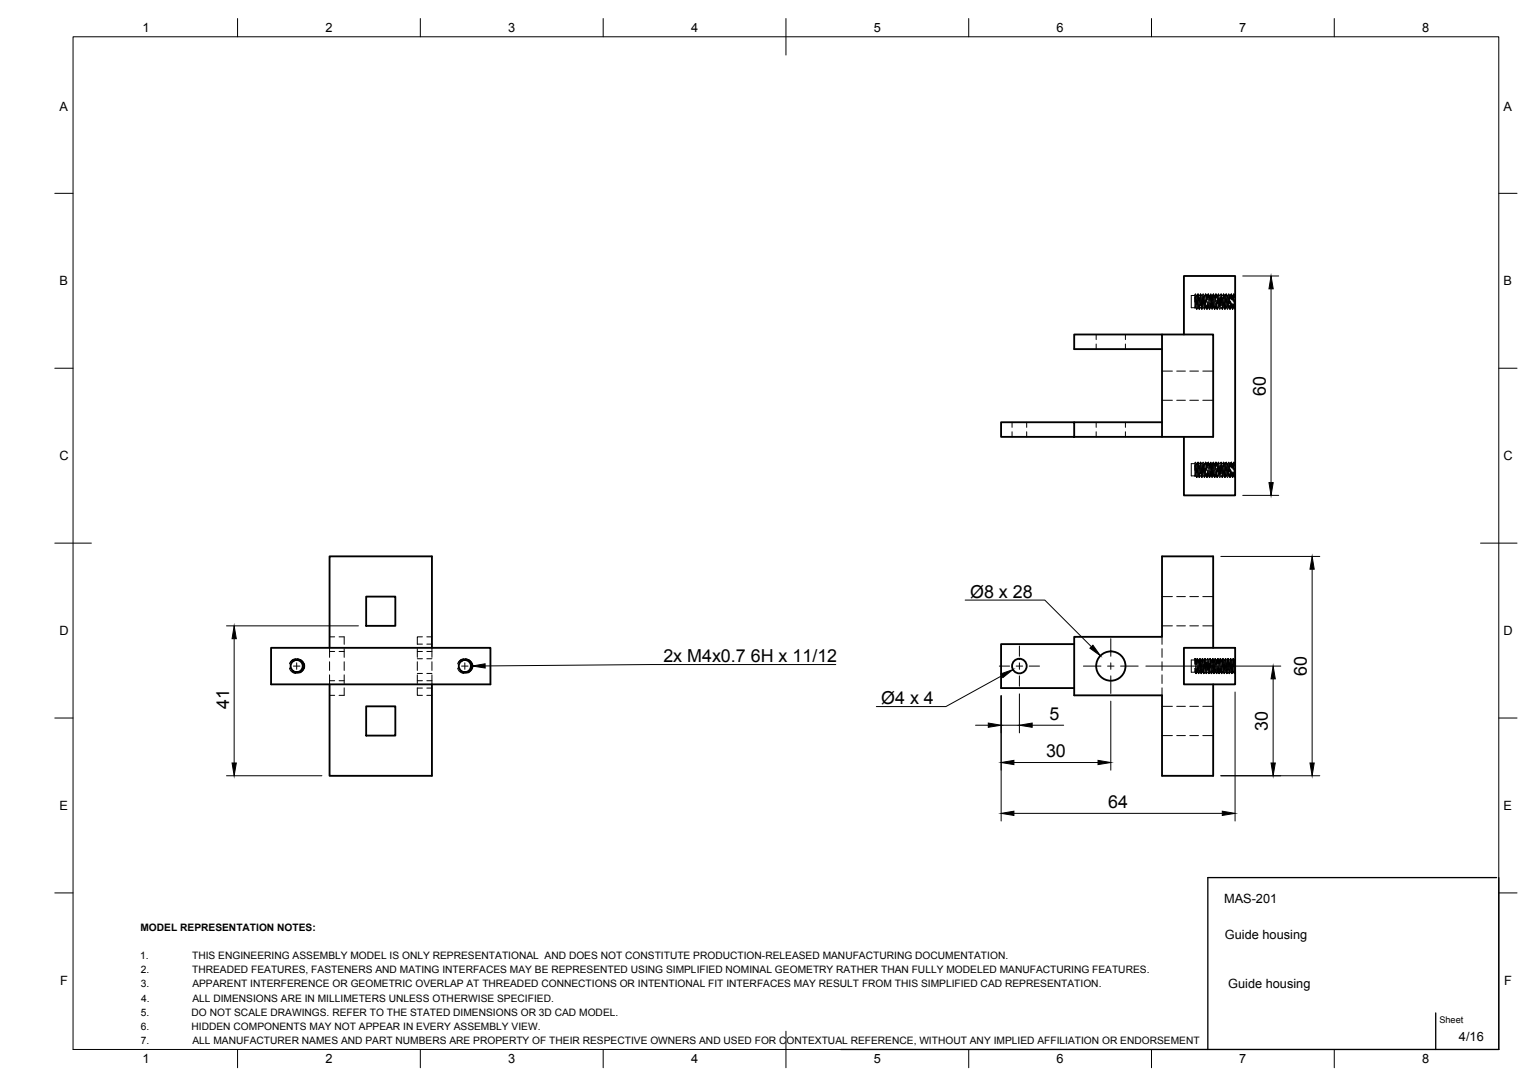
ISO-10303-21;
HEADER;
/* Generated by software containing ST-Developer
 * from STEP Tools, Inc. (www.steptools.com) 
 */

FILE_DESCRIPTION(
/* description */ ('Independent manual two-gate roller-track escapement for nominal30mm d
iameter20mm wide feed rollers. Opposed gates are driven by native capt
ured pin-slot loops with positive curved-slot travel stops at\X\B116de
g. Repeated gate/pin/washer/clip instances, adapted native common bear
ing families, full retaining lips and rotating polymer grip. External 
workpieces, gravity feeder/incline and mount anchors outside assembly.
 No powered-feed compatibility, impact, capacity, safety, force, wear 
or life rating.'),
/* implementation_level */ '2;1');

FILE_NAME(
/* name */ 'Guide housing.step',
/* time_stamp */ '2026-11-08T18:43:23-08:00',
/* author */ (''),
/* organization */ (''),
/* preprocessor_version */ 'ST-DEVELOPER v20.2',
/* originating_system */ 'Autodesk Translation Framework v15.17.0.0',
/* authorisation */ '');

FILE_SCHEMA (('AUTOMOTIVE_DESIGN { 1 0 10303 214 3 1 1 }'));
ENDSEC;

DATA;
#10=MECHANICAL_DESIGN_GEOMETRIC_PRESENTATION_REPRESENTATION('',(#456),#19863);
#117=B_SPLINE_SURFACE_WITH_KNOTS('',3,3,((#11345,#11346,#11347,#11348,#11349,
#11350,#11351,#11352,#11353,#11354,#11355,#11356,#11357,#11358,#11359,#11360,
#11361,#11362,#11363,#11364,#11365,#11366,#11367,#11368,#11369,#11370,#11371,
#11372,#11373,#11374,#11375,#11376,#11377,#11378,#11379,#11380,#11381,#11382,
#11383,#11384,#11385,#11386,#11387,#11388,#11389,#11390,#11391,#11392,#11393,
#11394,#11395,#11396,#11397,#11398,#11399,#11400,#11401,#11402,#11403,#11404,
#11405,#11406,#11407,#11408,#11409,#11410,#11411,#11412,#11413,#11414,#11415,
#11416,#11417,#11418,#11419,#11420,#11421,#11422,#11423,#11424,#11425,#11426,
#11427,#11428,#11429,#11430,#11431,#11432,#11433,#11434,#11435,#11436,#11437,
#11438,#11439,#11440,#11441,#11442,#11443,#11444,#11445,#11446,#11447,#11448),
(#11449,#11450,#11451,#11452,#11453,#11454,#11455,#11456,#11457,#11458,
#11459,#11460,#11461,#11462,#11463,#11464,#11465,#11466,#11467,#11468,#11469,
#11470,#11471,#11472,#11473,#11474,#11475,#11476,#11477,#11478,#11479,#11480,
#11481,#11482,#11483,#11484,#11485,#11486,#11487,#11488,#11489,#11490,#11491,
#11492,#11493,#11494,#11495,#11496,#11497,#11498,#11499,#11500,#11501,#11502,
#11503,#11504,#11505,#11506,#11507,#11508,#11509,#11510,#11511,#11512,#11513,
#11514,#11515,#11516,#11517,#11518,#11519,#11520,#11521,#11522,#11523,#11524,
#11525,#11526,#11527,#11528,#11529,#11530,#11531,#11532,#11533,#11534,#11535,
#11536,#11537,#11538,#11539,#11540,#11541,#11542,#11543,#11544,#11545,#11546,
#11547,#11548,#11549,#11550,#11551,#11552),(#11553,#11554,#11555,#11556,
#11557,#11558,#11559,#11560,#11561,#11562,#11563,#11564,#11565,#11566,#11567,
#11568,#11569,#11570,#11571,#11572,#11573,#11574,#11575,#11576,#11577,#11578,
#11579,#11580,#11581,#11582,#11583,#11584,#11585,#11586,#11587,#11588,#11589,
#11590,#11591,#11592,#11593,#11594,#11595,#11596,#11597,#11598,#11599,#11600,
#11601,#11602,#11603,#11604,#11605,#11606,#11607,#11608,#11609,#11610,#11611,
#11612,#11613,#11614,#11615,#11616,#11617,#11618,#11619,#11620,#11621,#11622,
#11623,#11624,#11625,#11626,#11627,#11628,#11629,#11630,#11631,#11632,#11633,
#11634,#11635,#11636,#11637,#11638,#11639,#11640,#11641,#11642,#11643,#11644,
#11645,#11646,#11647,#11648,#11649,#11650,#11651,#11652,#11653,#11654,#11655,
#11656),(#11657,#11658,#11659,#11660,#11661,#11662,#11663,#11664,#11665,
#11666,#11667,#11668,#11669,#11670,#11671,#11672,#11673,#11674,#11675,#11676,
#11677,#11678,#11679,#11680,#11681,#11682,#11683,#11684,#11685,#11686,#11687,
#11688,#11689,#11690,#11691,#11692,#11693,#11694,#11695,#11696,#11697,#11698,
#11699,#11700,#11701,#11702,#11703,#11704,#11705,#11706,#11707,#11708,#11709,
#11710,#11711,#11712,#11713,#11714,#11715,#11716,#11717,#11718,#11719,#11720,
#11721,#11722,#11723,#11724,#11725,#11726,#11727,#11728,#11729,#11730,#11731,
#11732,#11733,#11734,#11735,#11736,#11737,#11738,#11739,#11740,#11741,#11742,
#11743,#11744,#11745,#11746,#11747,#11748,#11749,#11750,#11751,#11752,#11753,
#11754,#11755,#11756,#11757,#11758,#11759,#11760)),.UNSPECIFIED.,.F.,.F.,
 .F.,(4,4),(4,1,1,1,1,1,1,1,1,1,1,1,1,1,1,1,1,1,1,1,1,1,1,1,1,1,1,1,1,1,
1,1,1,1,1,1,1,1,1,1,1,1,1,1,1,1,1,1,1,1,1,1,1,1,1,1,1,1,1,1,1,1,1,1,1,1,
1,1,1,1,1,1,1,1,1,1,1,1,1,1,1,1,1,1,1,1,1,1,1,1,1,1,1,1,1,1,1,1,1,1,1,4),
(0.,0.0448889834294942),(11.8615800042566,12.8591085386932,13.8566370731298,
14.8541656075664,15.851694142003,16.8492226764396,17.8467512108762,18.8442797453128,
19.8418082797494,20.839336814186,21.8368653486226,22.8343938830592,23.8319224174958,
24.8294509519324,25.826979486369,26.8245080208056,27.8220365552422,28.8195650896788,
29.8170936241154,30.814622158552,31.8121506929886,32.8096792274252,33.8072077618618,
34.8047362962984,35.802264830735,36.7997933651716,37.7973218996082,38.7948504340448,
39.7923789684814,40.789907502918,41.7874360373546,42.7849645717912,43.7824931062278,
44.7800216406644,45.777550175101,46.7750787095376,47.7726072439742,48.7701357784108,
49.7676643128474,50.765192847284,51.7627213817206,52.7602499161572,53.7577784505938,
54.7553069850304,55.752835519467,56.7503640539036,57.7478925883402,58.7454211227768,
59.7429496572134,60.74047819165,61.7380067260866,62.7355352605232,63.7330637949598,
64.7305923293964,65.728120863833,66.7256493982696,67.7231779327062,68.7207064671428,
69.7182350015794,70.715763536016,71.7132920704526,72.7108206048892,73.7083491393258,
74.7058776737624,75.703406208199,76.7009347426356,77.6984632770722,78.6959918115088,
79.6935203459454,80.691048880382,81.6885774148186,82.6861059492552,83.6836344836918,
84.6811630181284,85.678691552565,86.6762200870016,87.6737486214382,88.6712771558748,
89.6688056903114,90.666334224748,91.6638627591846,92.6613912936212,93.6589198280578,
94.6564483624944,95.653976896931,96.6515054313676,97.6490339658042,98.6465625002408,
99.6440910346774,100.641619569114,101.639148103551,102.636676637987,103.634205172424,
104.63173370686,105.629262241297,106.626790775734,107.62431931017,108.621847844607,
109.619376379043,110.61690491348,111.614433447917,112.611961982353),
 .UNSPECIFIED.);
#118=B_SPLINE_SURFACE_WITH_KNOTS('',3,3,((#11868,#11869,#11870,#11871,#11872,
#11873,#11874,#11875,#11876,#11877,#11878,#11879,#11880,#11881,#11882,#11883,
#11884,#11885,#11886,#11887,#11888,#11889,#11890,#11891,#11892,#11893,#11894,
#11895,#11896,#11897,#11898,#11899,#11900,#11901,#11902,#11903,#11904,#11905,
#11906,#11907,#11908,#11909,#11910,#11911,#11912,#11913,#11914,#11915,#11916,
#11917,#11918,#11919,#11920,#11921,#11922,#11923,#11924,#11925,#11926,#11927,
#11928,#11929,#11930,#11931,#11932,#11933,#11934,#11935,#11936,#11937,#11938,
#11939,#11940,#11941,#11942,#11943,#11944,#11945,#11946,#11947,#11948,#11949,
#11950,#11951,#11952,#11953,#11954,#11955,#11956,#11957,#11958,#11959,#11960,
#11961,#11962,#11963,#11964,#11965,#11966,#11967,#11968,#11969,#11970,#11971),
(#11972,#11973,#11974,#11975,#11976,#11977,#11978,#11979,#11980,#11981,
#11982,#11983,#11984,#11985,#11986,#11987,#11988,#11989,#11990,#11991,#11992,
#11993,#11994,#11995,#11996,#11997,#11998,#11999,#12000,#12001,#12002,#12003,
#12004,#12005,#12006,#12007,#12008,#12009,#12010,#12011,#12012,#12013,#12014,
#12015,#12016,#12017,#12018,#12019,#12020,#12021,#12022,#12023,#12024,#12025,
#12026,#12027,#12028,#12029,#12030,#12031,#12032,#12033,#12034,#12035,#12036,
#12037,#12038,#12039,#12040,#12041,#12042,#12043,#12044,#12045,#12046,#12047,
#12048,#12049,#12050,#12051,#12052,#12053,#12054,#12055,#12056,#12057,#12058,
#12059,#12060,#12061,#12062,#12063,#12064,#12065,#12066,#12067,#12068,#12069,
#12070,#12071,#12072,#12073,#12074,#12075),(#12076,#12077,#12078,#12079,
#12080,#12081,#12082,#12083,#12084,#12085,#12086,#12087,#12088,#12089,#12090,
#12091,#12092,#12093,#12094,#12095,#12096,#12097,#12098,#12099,#12100,#12101,
#12102,#12103,#12104,#12105,#12106,#12107,#12108,#12109,#12110,#12111,#12112,
#12113,#12114,#12115,#12116,#12117,#12118,#12119,#12120,#12121,#12122,#12123,
#12124,#12125,#12126,#12127,#12128,#12129,#12130,#12131,#12132,#12133,#12134,
#12135,#12136,#12137,#12138,#12139,#12140,#12141,#12142,#12143,#12144,#12145,
#12146,#12147,#12148,#12149,#12150,#12151,#12152,#12153,#12154,#12155,#12156,
#12157,#12158,#12159,#12160,#12161,#12162,#12163,#12164,#12165,#12166,#12167,
#12168,#12169,#12170,#12171,#12172,#12173,#12174,#12175,#12176,#12177,#12178,
#12179),(#12180,#12181,#12182,#12183,#12184,#12185,#12186,#12187,#12188,
#12189,#12190,#12191,#12192,#12193,#12194,#12195,#12196,#12197,#12198,#12199,
#12200,#12201,#12202,#12203,#12204,#12205,#12206,#12207,#12208,#12209,#12210,
#12211,#12212,#12213,#12214,#12215,#12216,#12217,#12218,#12219,#12220,#12221,
#12222,#12223,#12224,#12225,#12226,#12227,#12228,#12229,#12230,#12231,#12232,
#12233,#12234,#12235,#12236,#12237,#12238,#12239,#12240,#12241,#12242,#12243,
#12244,#12245,#12246,#12247,#12248,#12249,#12250,#12251,#12252,#12253,#12254,
#12255,#12256,#12257,#12258,#12259,#12260,#12261,#12262,#12263,#12264,#12265,
#12266,#12267,#12268,#12269,#12270,#12271,#12272,#12273,#12274,#12275,#12276,
#12277,#12278,#12279,#12280,#12281,#12282,#12283)),.UNSPECIFIED.,.F.,.F.,
 .F.,(4,4),(4,1,1,1,1,1,1,1,1,1,1,1,1,1,1,1,1,1,1,1,1,1,1,1,1,1,1,1,1,1,
1,1,1,1,1,1,1,1,1,1,1,1,1,1,1,1,1,1,1,1,1,1,1,1,1,1,1,1,1,1,1,1,1,1,1,1,
1,1,1,1,1,1,1,1,1,1,1,1,1,1,1,1,1,1,1,1,1,1,1,1,1,1,1,1,1,1,1,1,1,1,1,4),
(0.,0.0448889834294942),(14.3981410127769,15.3956695472135,16.3931980816501,
17.3907266160867,18.3882551505233,19.3857836849599,20.3833122193965,21.3808407538331,
22.3783692882697,23.3758978227063,24.3734263571429,25.3709548915795,26.3684834260161,
27.3660119604527,28.3635404948893,29.3610690293259,30.3585975637625,31.3561260981991,
32.3536546326357,33.3511831670723,34.3487117015089,35.3462402359455,36.3437687703821,
37.3412973048187,38.3388258392553,39.3363543736919,40.3338829081285,41.3314114425651,
42.3289399770017,43.3264685114383,44.3239970458749,45.3215255803115,46.3190541147481,
47.3165826491847,48.3141111836213,49.3116397180579,50.3091682524945,51.3066967869311,
52.3042253213677,53.3017538558043,54.2992823902409,55.2968109246775,56.294339459114,
57.2918679935507,58.2893965279873,59.2869250624238,60.2844535968605,61.281982131297,
62.2795106657336,63.2770392001703,64.2745677346068,65.2720962690434,66.26962480348,
67.2671533379167,68.2646818723532,69.2622104067898,70.2597389412264,71.257267475663,
72.2547960100996,73.2523245445362,74.2498530789728,75.2473816134094,76.244910147846,
77.2424386822826,78.2399672167192,79.2374957511558,80.2350242855924,81.232552820029,
82.2300813544656,83.2276098889022,84.2251384233388,85.2226669577754,86.220195492212,
87.2177240266486,88.2152525610852,89.2127810955218,90.2103096299584,91.207838164395,
92.2053666988316,93.2028952332682,94.2004237677048,95.1979523021414,96.195480836578,
97.1930093710146,98.1905379054512,99.1880664398878,100.185594974324,101.183123508761,
102.180652043198,103.178180577634,104.175709112071,105.173237646507,106.170766180944,
107.168294715381,108.165823249817,109.163351784254,110.16088031869,111.158408853127,
112.155937387564,113.153465922,114.150994456437,115.148522990873),
 .UNSPECIFIED.);
#119=B_SPLINE_SURFACE_WITH_KNOTS('',3,3,((#12588,#12589,#12590,#12591,#12592,
#12593,#12594,#12595,#12596,#12597,#12598,#12599,#12600,#12601,#12602,#12603,
#12604,#12605,#12606,#12607,#12608,#12609,#12610,#12611,#12612,#12613,#12614,
#12615,#12616,#12617,#12618,#12619,#12620,#12621,#12622,#12623,#12624,#12625,
#12626,#12627,#12628,#12629,#12630,#12631,#12632,#12633,#12634,#12635,#12636,
#12637,#12638,#12639,#12640,#12641,#12642,#12643,#12644,#12645,#12646,#12647,
#12648,#12649,#12650,#12651,#12652,#12653,#12654,#12655,#12656,#12657,#12658,
#12659,#12660,#12661,#12662,#12663,#12664,#12665,#12666,#12667,#12668,#12669,
#12670,#12671,#12672,#12673,#12674,#12675,#12676,#12677,#12678,#12679,#12680,
#12681,#12682,#12683,#12684,#12685,#12686,#12687,#12688,#12689,#12690,#12691),
(#12692,#12693,#12694,#12695,#12696,#12697,#12698,#12699,#12700,#12701,
#12702,#12703,#12704,#12705,#12706,#12707,#12708,#12709,#12710,#12711,#12712,
#12713,#12714,#12715,#12716,#12717,#12718,#12719,#12720,#12721,#12722,#12723,
#12724,#12725,#12726,#12727,#12728,#12729,#12730,#12731,#12732,#12733,#12734,
#12735,#12736,#12737,#12738,#12739,#12740,#12741,#12742,#12743,#12744,#12745,
#12746,#12747,#12748,#12749,#12750,#12751,#12752,#12753,#12754,#12755,#12756,
#12757,#12758,#12759,#12760,#12761,#12762,#12763,#12764,#12765,#12766,#12767,
#12768,#12769,#12770,#12771,#12772,#12773,#12774,#12775,#12776,#12777,#12778,
#12779,#12780,#12781,#12782,#12783,#12784,#12785,#12786,#12787,#12788,#12789,
#12790,#12791,#12792,#12793,#12794,#12795),(#12796,#12797,#12798,#12799,
#12800,#12801,#12802,#12803,#12804,#12805,#12806,#12807,#12808,#12809,#12810,
#12811,#12812,#12813,#12814,#12815,#12816,#12817,#12818,#12819,#12820,#12821,
#12822,#12823,#12824,#12825,#12826,#12827,#12828,#12829,#12830,#12831,#12832,
#12833,#12834,#12835,#12836,#12837,#12838,#12839,#12840,#12841,#12842,#12843,
#12844,#12845,#12846,#12847,#12848,#12849,#12850,#12851,#12852,#12853,#12854,
#12855,#12856,#12857,#12858,#12859,#12860,#12861,#12862,#12863,#12864,#12865,
#12866,#12867,#12868,#12869,#12870,#12871,#12872,#12873,#12874,#12875,#12876,
#12877,#12878,#12879,#12880,#12881,#12882,#12883,#12884,#12885,#12886,#12887,
#12888,#12889,#12890,#12891,#12892,#12893,#12894,#12895,#12896,#12897,#12898,
#12899),(#12900,#12901,#12902,#12903,#12904,#12905,#12906,#12907,#12908,
#12909,#12910,#12911,#12912,#12913,#12914,#12915,#12916,#12917,#12918,#12919,
#12920,#12921,#12922,#12923,#12924,#12925,#12926,#12927,#12928,#12929,#12930,
#12931,#12932,#12933,#12934,#12935,#12936,#12937,#12938,#12939,#12940,#12941,
#12942,#12943,#12944,#12945,#12946,#12947,#12948,#12949,#12950,#12951,#12952,
#12953,#12954,#12955,#12956,#12957,#12958,#12959,#12960,#12961,#12962,#12963,
#12964,#12965,#12966,#12967,#12968,#12969,#12970,#12971,#12972,#12973,#12974,
#12975,#12976,#12977,#12978,#12979,#12980,#12981,#12982,#12983,#12984,#12985,
#12986,#12987,#12988,#12989,#12990,#12991,#12992,#12993,#12994,#12995,#12996,
#12997,#12998,#12999,#13000,#13001,#13002,#13003)),.UNSPECIFIED.,.F.,.F.,
 .F.,(4,4),(4,1,1,1,1,1,1,1,1,1,1,1,1,1,1,1,1,1,1,1,1,1,1,1,1,1,1,1,1,1,
1,1,1,1,1,1,1,1,1,1,1,1,1,1,1,1,1,1,1,1,1,1,1,1,1,1,1,1,1,1,1,1,1,1,1,1,
1,1,1,1,1,1,1,1,1,1,1,1,1,1,1,1,1,1,1,1,1,1,1,1,1,1,1,1,1,1,1,1,1,1,1,4),
(0.,0.0448889834294942),(11.8615800042566,12.8591085386932,13.8566370731298,
14.8541656075664,15.851694142003,16.8492226764396,17.8467512108762,18.8442797453128,
19.8418082797494,20.839336814186,21.8368653486226,22.8343938830592,23.8319224174958,
24.8294509519324,25.826979486369,26.8245080208056,27.8220365552422,28.8195650896788,
29.8170936241154,30.814622158552,31.8121506929886,32.8096792274252,33.8072077618618,
34.8047362962984,35.802264830735,36.7997933651716,37.7973218996082,38.7948504340448,
39.7923789684814,40.789907502918,41.7874360373546,42.7849645717912,43.7824931062278,
44.7800216406644,45.777550175101,46.7750787095376,47.7726072439742,48.7701357784108,
49.7676643128474,50.765192847284,51.7627213817206,52.7602499161572,53.7577784505938,
54.7553069850304,55.752835519467,56.7503640539036,57.7478925883402,58.7454211227768,
59.7429496572134,60.74047819165,61.7380067260866,62.7355352605232,63.7330637949598,
64.7305923293964,65.728120863833,66.7256493982696,67.7231779327062,68.7207064671428,
69.7182350015794,70.715763536016,71.7132920704526,72.7108206048892,73.7083491393258,
74.7058776737624,75.703406208199,76.7009347426356,77.6984632770722,78.6959918115088,
79.6935203459454,80.691048880382,81.6885774148186,82.6861059492552,83.6836344836918,
84.6811630181284,85.678691552565,86.6762200870016,87.6737486214382,88.6712771558748,
89.6688056903114,90.666334224748,91.6638627591846,92.6613912936212,93.6589198280578,
94.6564483624944,95.653976896931,96.6515054313676,97.6490339658042,98.6465625002408,
99.6440910346774,100.641619569114,101.639148103551,102.636676637987,103.634205172424,
104.63173370686,105.629262241297,106.626790775734,107.62431931017,108.621847844607,
109.619376379043,110.61690491348,111.614433447917,112.611961982353),
 .UNSPECIFIED.);
#120=B_SPLINE_SURFACE_WITH_KNOTS('',3,3,((#13111,#13112,#13113,#13114,#13115,
#13116,#13117,#13118,#13119,#13120,#13121,#13122,#13123,#13124,#13125,#13126,
#13127,#13128,#13129,#13130,#13131,#13132,#13133,#13134,#13135,#13136,#13137,
#13138,#13139,#13140,#13141,#13142,#13143,#13144,#13145,#13146,#13147,#13148,
#13149,#13150,#13151,#13152,#13153,#13154,#13155,#13156,#13157,#13158,#13159,
#13160,#13161,#13162,#13163,#13164,#13165,#13166,#13167,#13168,#13169,#13170,
#13171,#13172,#13173,#13174,#13175,#13176,#13177,#13178,#13179,#13180,#13181,
#13182,#13183,#13184,#13185,#13186,#13187,#13188,#13189,#13190,#13191,#13192,
#13193,#13194,#13195,#13196,#13197,#13198,#13199,#13200,#13201,#13202,#13203,
#13204,#13205,#13206,#13207,#13208,#13209,#13210,#13211,#13212,#13213,#13214),
(#13215,#13216,#13217,#13218,#13219,#13220,#13221,#13222,#13223,#13224,
#13225,#13226,#13227,#13228,#13229,#13230,#13231,#13232,#13233,#13234,#13235,
#13236,#13237,#13238,#13239,#13240,#13241,#13242,#13243,#13244,#13245,#13246,
#13247,#13248,#13249,#13250,#13251,#13252,#13253,#13254,#13255,#13256,#13257,
#13258,#13259,#13260,#13261,#13262,#13263,#13264,#13265,#13266,#13267,#13268,
#13269,#13270,#13271,#13272,#13273,#13274,#13275,#13276,#13277,#13278,#13279,
#13280,#13281,#13282,#13283,#13284,#13285,#13286,#13287,#13288,#13289,#13290,
#13291,#13292,#13293,#13294,#13295,#13296,#13297,#13298,#13299,#13300,#13301,
#13302,#13303,#13304,#13305,#13306,#13307,#13308,#13309,#13310,#13311,#13312,
#13313,#13314,#13315,#13316,#13317,#13318),(#13319,#13320,#13321,#13322,
#13323,#13324,#13325,#13326,#13327,#13328,#13329,#13330,#13331,#13332,#13333,
#13334,#13335,#13336,#13337,#13338,#13339,#13340,#13341,#13342,#13343,#13344,
#13345,#13346,#13347,#13348,#13349,#13350,#13351,#13352,#13353,#13354,#13355,
#13356,#13357,#13358,#13359,#13360,#13361,#13362,#13363,#13364,#13365,#13366,
#13367,#13368,#13369,#13370,#13371,#13372,#13373,#13374,#13375,#13376,#13377,
#13378,#13379,#13380,#13381,#13382,#13383,#13384,#13385,#13386,#13387,#13388,
#13389,#13390,#13391,#13392,#13393,#13394,#13395,#13396,#13397,#13398,#13399,
#13400,#13401,#13402,#13403,#13404,#13405,#13406,#13407,#13408,#13409,#13410,
#13411,#13412,#13413,#13414,#13415,#13416,#13417,#13418,#13419,#13420,#13421,
#13422),(#13423,#13424,#13425,#13426,#13427,#13428,#13429,#13430,#13431,
#13432,#13433,#13434,#13435,#13436,#13437,#13438,#13439,#13440,#13441,#13442,
#13443,#13444,#13445,#13446,#13447,#13448,#13449,#13450,#13451,#13452,#13453,
#13454,#13455,#13456,#13457,#13458,#13459,#13460,#13461,#13462,#13463,#13464,
#13465,#13466,#13467,#13468,#13469,#13470,#13471,#13472,#13473,#13474,#13475,
#13476,#13477,#13478,#13479,#13480,#13481,#13482,#13483,#13484,#13485,#13486,
#13487,#13488,#13489,#13490,#13491,#13492,#13493,#13494,#13495,#13496,#13497,
#13498,#13499,#13500,#13501,#13502,#13503,#13504,#13505,#13506,#13507,#13508,
#13509,#13510,#13511,#13512,#13513,#13514,#13515,#13516,#13517,#13518,#13519,
#13520,#13521,#13522,#13523,#13524,#13525,#13526)),.UNSPECIFIED.,.F.,.F.,
 .F.,(4,4),(4,1,1,1,1,1,1,1,1,1,1,1,1,1,1,1,1,1,1,1,1,1,1,1,1,1,1,1,1,1,
1,1,1,1,1,1,1,1,1,1,1,1,1,1,1,1,1,1,1,1,1,1,1,1,1,1,1,1,1,1,1,1,1,1,1,1,
1,1,1,1,1,1,1,1,1,1,1,1,1,1,1,1,1,1,1,1,1,1,1,1,1,1,1,1,1,1,1,1,1,1,1,4),
(0.,0.0448889834294942),(14.3981410127769,15.3956695472135,16.3931980816501,
17.3907266160867,18.3882551505233,19.3857836849599,20.3833122193965,21.3808407538331,
22.3783692882697,23.3758978227063,24.3734263571429,25.3709548915795,26.3684834260161,
27.3660119604527,28.3635404948893,29.3610690293259,30.3585975637625,31.3561260981991,
32.3536546326357,33.3511831670723,34.3487117015089,35.3462402359455,36.3437687703821,
37.3412973048187,38.3388258392553,39.3363543736919,40.3338829081285,41.3314114425651,
42.3289399770017,43.3264685114383,44.3239970458749,45.3215255803115,46.3190541147481,
47.3165826491847,48.3141111836213,49.3116397180579,50.3091682524945,51.3066967869311,
52.3042253213677,53.3017538558043,54.2992823902409,55.2968109246775,56.294339459114,
57.2918679935507,58.2893965279873,59.2869250624238,60.2844535968605,61.281982131297,
62.2795106657336,63.2770392001703,64.2745677346068,65.2720962690434,66.26962480348,
67.2671533379167,68.2646818723532,69.2622104067898,70.2597389412264,71.257267475663,
72.2547960100996,73.2523245445362,74.2498530789728,75.2473816134094,76.244910147846,
77.2424386822826,78.2399672167192,79.2374957511558,80.2350242855924,81.232552820029,
82.2300813544656,83.2276098889022,84.2251384233388,85.2226669577754,86.220195492212,
87.2177240266486,88.2152525610852,89.2127810955218,90.2103096299584,91.207838164395,
92.2053666988316,93.2028952332682,94.2004237677048,95.1979523021414,96.195480836578,
97.1930093710146,98.1905379054512,99.1880664398878,100.185594974324,101.183123508761,
102.180652043198,103.178180577634,104.175709112071,105.173237646507,106.170766180944,
107.168294715381,108.165823249817,109.163351784254,110.16088031869,111.158408853127,
112.155937387564,113.153465922,114.150994456437,115.148522990873),
 .UNSPECIFIED.);
#127=B_SPLINE_CURVE_WITH_KNOTS('',3,(#8912,#8913,#8914,#8915,#8916,#8917,
#8918,#8919,#8920,#8921,#8922,#8923,#8924,#8925,#8926,#8927,#8928,#8929,
#8930),.UNSPECIFIED.,.F.,.F.,(4,3,3,3,3,3,4),(95.5576018628658,95.7627393059135,
96.7602678403501,97.7577963747867,98.7553249092233,99.7528534436599,100.750381978097),
 .UNSPECIFIED.);
#128=B_SPLINE_CURVE_WITH_KNOTS('',3,(#8934,#8935,#8936,#8937),
 .UNSPECIFIED.,.F.,.F.,(4,4),(-98.7357691128221,-98.0941628713861),
 .UNSPECIFIED.);
#129=B_SPLINE_CURVE_WITH_KNOTS('',3,(#8941,#8942,#8943,#8944,#8945,#8946,
#8947,#8948,#8949,#8950,#8951,#8952,#8953,#8954,#8955,#8956,#8957,#8958,
#8959,#8960,#8961,#8962),.UNSPECIFIED.,.F.,.F.,(4,3,3,3,3,3,3,4),(-98.0941628713861,
-97.7577963747867,-96.7602678403501,-95.7627393059135,-94.7652107714769,
-93.7676822370403,-92.7701537026037,-91.8109775642065),.UNSPECIFIED.);
#130=B_SPLINE_CURVE_WITH_KNOTS('',3,(#8967,#8968,#8969,#8970,#8971,#8972,
#8973,#8974,#8975,#8976,#8977,#8978,#8979,#8980,#8981,#8982,#8983,#8984,
#8985,#8986,#8987,#8988),.UNSPECIFIED.,.F.,.F.,(4,3,3,3,3,3,3,4),(89.2744165556862,
89.7775680992939,90.7750966337306,91.7726251681671,92.7701537026037,93.7676822370403,
94.7652107714769,95.5576018628658),.UNSPECIFIED.);
#131=B_SPLINE_CURVE_WITH_KNOTS('',3,(#8989,#8990,#8991,#8992,#8993,#8994,
#8995,#8996,#8997,#8998,#8999,#9000,#9001,#9002,#9003,#9004,#9005,#9006,
#9007,#9008,#9009,#9010,#9011,#9012,#9013),.UNSPECIFIED.,.F.,.F.,(4,3,3,
3,3,3,3,3,4),(-91.8109775642065,-91.7726251681671,-90.7750966337305,-89.7775680992939,
-88.7800395648573,-87.7825110304207,-86.7849824959842,-85.7874539615476,
-85.5277922570269),.UNSPECIFIED.);
#132=B_SPLINE_CURVE_WITH_KNOTS('',3,(#9018,#9019,#9020,#9021,#9022,#9023,
#9024,#9025,#9026,#9027,#9028,#9029,#9030,#9031,#9032,#9033,#9034,#9035,
#9036,#9037,#9038,#9039),.UNSPECIFIED.,.F.,.F.,(4,3,3,3,3,3,3,4),(82.9912312485066,
83.7923968926743,84.7899254271109,85.7874539615476,86.7849824959841,87.7825110304207,
88.7800395648573,89.2744165556862),.UNSPECIFIED.);
#133=B_SPLINE_CURVE_WITH_KNOTS('',3,(#9040,#9041,#9042,#9043,#9044,#9045,
#9046,#9047,#9048,#9049,#9050,#9051,#9052,#9053,#9054,#9055,#9056,#9057,
#9058,#9059,#9060,#9061),.UNSPECIFIED.,.F.,.F.,(4,3,3,3,3,3,3,4),(-85.5277922570269,
-84.789925427111,-83.7923968926743,-82.7948683582377,-81.7973398238011,
-80.7998112893646,-79.8022827549279,-79.2446069498473),.UNSPECIFIED.);
#134=B_SPLINE_CURVE_WITH_KNOTS('',3,(#9066,#9067,#9068,#9069,#9070,#9071,
#9072,#9073,#9074,#9075,#9076,#9077,#9078,#9079,#9080,#9081,#9082,#9083,
#9084,#9085,#9086,#9087,#9088,#9089,#9090),.UNSPECIFIED.,.F.,.F.,(4,3,3,
3,3,3,3,3,4),(76.708045941327,76.8096971516181,77.8072256860547,78.8047542204914,
79.8022827549279,80.7998112893646,81.7973398238011,82.7948683582377,82.9912312485066),
 .UNSPECIFIED.);
#135=B_SPLINE_CURVE_WITH_KNOTS('',3,(#9091,#9092,#9093,#9094,#9095,#9096,
#9097,#9098,#9099,#9100,#9101,#9102,#9103,#9104,#9105,#9106,#9107,#9108,
#9109,#9110,#9111,#9112),.UNSPECIFIED.,.F.,.F.,(4,3,3,3,3,3,3,4),(-79.2446069498473,
-78.8047542204913,-77.8072256860547,-76.8096971516181,-75.8121686171815,
-74.8146400827449,-73.8171115483083,-72.9614216426677),.UNSPECIFIED.);
#136=B_SPLINE_CURVE_WITH_KNOTS('',3,(#9117,#9118,#9119,#9120,#9121,#9122,
#9123,#9124,#9125,#9126,#9127,#9128,#9129,#9130,#9131,#9132,#9133,#9134,
#9135,#9136,#9137,#9138),.UNSPECIFIED.,.F.,.F.,(4,3,3,3,3,3,3,4),(70.4248606341474,
70.8245259449985,71.8220544794352,72.8195830138717,73.8171115483084,74.8146400827449,
75.8121686171816,76.708045941327),.UNSPECIFIED.);
#137=B_SPLINE_CURVE_WITH_KNOTS('',3,(#9139,#9140,#9141,#9142,#9143,#9144,
#9145,#9146,#9147,#9148,#9149,#9150,#9151,#9152,#9153,#9154,#9155,#9156,
#9157,#9158,#9159,#9160,#9161,#9162,#9163),.UNSPECIFIED.,.F.,.F.,(4,3,3,
3,3,3,3,3,4),(-72.9614216426677,-72.8195830138717,-71.8220544794352,-70.8245259449986,
-69.8269974105619,-68.8294688761253,-67.8319403416887,-66.8344118072522,
-66.6782363354881),.UNSPECIFIED.);
#138=B_SPLINE_CURVE_WITH_KNOTS('',3,(#9168,#9169,#9170,#9171,#9172,#9173,
#9174,#9175,#9176,#9177,#9178,#9179,#9180,#9181,#9182,#9183,#9184,#9185,
#9186,#9187,#9188,#9189),.UNSPECIFIED.,.F.,.F.,(4,3,3,3,3,3,3,4),(64.1416753269678,
64.839354738379,65.8368832728156,66.8344118072522,67.8319403416887,68.8294688761253,
69.8269974105619,70.4248606341474),.UNSPECIFIED.);
#139=B_SPLINE_CURVE_WITH_KNOTS('',3,(#9190,#9191,#9192,#9193,#9194,#9195,
#9196,#9197,#9198,#9199,#9200,#9201,#9202,#9203,#9204,#9205,#9206,#9207,
#9208,#9209,#9210,#9211),.UNSPECIFIED.,.F.,.F.,(4,3,3,3,3,3,3,4),(-66.6782363354881,
-65.8368832728156,-64.839354738379,-63.8418262039424,-62.8442976695058,
-61.8467691350692,-60.8492406006326,-60.3950510283086),.UNSPECIFIED.);
#140=B_SPLINE_CURVE_WITH_KNOTS('',3,(#9216,#9217,#9218,#9219,#9220,#9221,
#9222,#9223,#9224,#9225,#9226,#9227,#9228,#9229,#9230,#9231,#9232,#9233,
#9234,#9235,#9236,#9237),.UNSPECIFIED.,.F.,.F.,(4,3,3,3,3,3,3,4),(57.8584900197882,
58.8541835317594,59.851712066196,60.8492406006326,61.8467691350692,62.8442976695058,
63.8418262039424,64.1416753269678),.UNSPECIFIED.);
#141=B_SPLINE_CURVE_WITH_KNOTS('',3,(#9238,#9239,#9240,#9241,#9242,#9243,
#9244,#9245,#9246,#9247,#9248,#9249,#9250,#9251,#9252,#9253,#9254,#9255,
#9256,#9257,#9258,#9259),.UNSPECIFIED.,.F.,.F.,(4,3,3,3,3,3,3,4),(-60.3950510283086,
-59.851712066196,-58.8541835317594,-57.8566549973228,-56.8591264628862,
-55.8615979284496,-54.864069394013,-54.111865721129),.UNSPECIFIED.);
#142=B_SPLINE_CURVE_WITH_KNOTS('',3,(#9264,#9265,#9266,#9267,#9268,#9269,
#9270,#9271,#9272,#9273,#9274,#9275,#9276,#9277,#9278,#9279,#9280,#9281,
#9282,#9283,#9284,#9285),.UNSPECIFIED.,.F.,.F.,(4,3,3,3,3,3,3,4),(51.5753047126086,
51.8714837907032,52.8690123251398,53.8665408595764,54.864069394013,55.8615979284496,
56.8591264628862,57.8584900197882),.UNSPECIFIED.);
#143=B_SPLINE_CURVE_WITH_KNOTS('',3,(#9286,#9287,#9288,#9289,#9290,#9291,
#9292,#9293,#9294,#9295,#9296,#9297,#9298,#9299,#9300,#9301,#9302,#9303,
#9304,#9305,#9306,#9307,#9308,#9309,#9310),.UNSPECIFIED.,.F.,.F.,(4,3,3,
3,3,3,3,3,4),(-54.111865721129,-53.8665408595764,-52.8690123251398,-51.8714837907032,
-50.8739552562666,-49.87642672183,-48.8788981873934,-47.8813696529568,-47.8286804139494),
 .UNSPECIFIED.);
#144=B_SPLINE_CURVE_WITH_KNOTS('',3,(#9315,#9316,#9317,#9318,#9319,#9320,
#9321,#9322,#9323,#9324,#9325,#9326,#9327,#9328,#9329,#9330,#9331,#9332,
#9333,#9334,#9335,#9336),.UNSPECIFIED.,.F.,.F.,(4,3,3,3,3,3,3,4),(45.2921194054291,
45.8863125840836,46.8838411185202,47.8813696529568,48.8788981873934,49.87642672183,
50.8739552562666,51.5753047126086),.UNSPECIFIED.);
#145=B_SPLINE_CURVE_WITH_KNOTS('',3,(#9337,#9338,#9339,#9340,#9341,#9342,
#9343,#9344,#9345,#9346,#9347,#9348,#9349,#9350,#9351,#9352,#9353,#9354,
#9355,#9356,#9357,#9358),.UNSPECIFIED.,.F.,.F.,(4,3,3,3,3,3,3,4),(-47.8286804139494,
-46.8838411185202,-45.8863125840836,-44.888784049647,-43.8912555152104,
-42.8937269807738,-41.8961984463372,-41.5454951067698),.UNSPECIFIED.);
#146=B_SPLINE_CURVE_WITH_KNOTS('',3,(#9363,#9364,#9365,#9366,#9367,#9368,
#9369,#9370,#9371,#9372,#9373,#9374,#9375,#9376,#9377,#9378,#9379,#9380,
#9381,#9382,#9383,#9384),.UNSPECIFIED.,.F.,.F.,(4,3,3,3,3,3,3,4),(39.0089340982495,
39.901141377464,40.8986699119006,41.8961984463372,42.8937269807738,43.8912555152104,
44.888784049647,45.2921194054291),.UNSPECIFIED.);
#147=B_SPLINE_CURVE_WITH_KNOTS('',3,(#9385,#9386,#9387,#9388,#9389,#9390,
#9391,#9392,#9393,#9394,#9395,#9396,#9397,#9398,#9399,#9400,#9401,#9402,
#9403,#9404,#9405,#9406),.UNSPECIFIED.,.F.,.F.,(4,3,3,3,3,3,3,4),(-41.5454951067698,
-40.8986699119006,-39.901141377464,-38.9036128430274,-37.9060843085908,
-36.9085557741542,-35.9110272397176,-35.2623097995902),.UNSPECIFIED.);
#148=B_SPLINE_CURVE_WITH_KNOTS('',3,(#9411,#9412,#9413,#9414,#9415,#9416,
#9417,#9418,#9419,#9420,#9421,#9422,#9423,#9424,#9425,#9426,#9427,#9428,
#9429,#9430,#9431,#9432,#9433,#9434,#9435),.UNSPECIFIED.,.F.,.F.,(4,3,3,
3,3,3,3,3,4),(32.7257487910699,32.9184416364078,33.9159701708444,34.913498705281,
35.9110272397176,36.9085557741542,37.9060843085908,38.9036128430274,39.0089340982495),
 .UNSPECIFIED.);
#149=B_SPLINE_CURVE_WITH_KNOTS('',3,(#9436,#9437,#9438,#9439,#9440,#9441,
#9442,#9443,#9444,#9445,#9446,#9447,#9448,#9449,#9450,#9451,#9452,#9453,
#9454,#9455,#9456,#9457),.UNSPECIFIED.,.F.,.F.,(4,3,3,3,3,3,3,4),(-35.2623097995902,
-34.913498705281,-33.9159701708444,-32.9184416364078,-31.9209131019712,
-30.9233845675346,-29.925856033098,-28.9791244924106),.UNSPECIFIED.);
#150=B_SPLINE_CURVE_WITH_KNOTS('',3,(#9462,#9463,#9464,#9465,#9466,#9467,
#9468,#9469,#9470,#9471,#9472,#9473,#9474,#9475,#9476,#9477,#9478,#9479,
#9480,#9481,#9482,#9483),.UNSPECIFIED.,.F.,.F.,(4,3,3,3,3,3,3,4),(26.4425634838903,
26.9332704297882,27.9307989642248,28.9283274986614,29.925856033098,30.9233845675346,
31.9209131019712,32.7257487910699),.UNSPECIFIED.);
#151=B_SPLINE_CURVE_WITH_KNOTS('',3,(#9484,#9485,#9486,#9487,#9488,#9489,
#9490,#9491,#9492,#9493,#9494,#9495,#9496,#9497,#9498,#9499,#9500,#9501,
#9502,#9503,#9504,#9505,#9506,#9507,#9508),.UNSPECIFIED.,.F.,.F.,(4,3,3,
3,3,3,3,3,4),(-28.9791244924106,-28.9283274986614,-27.9307989642248,-26.9332704297882,
-25.9357418953516,-24.938213360915,-23.9406848264784,-22.9431562920418,
-22.695939185231),.UNSPECIFIED.);
#152=B_SPLINE_CURVE_WITH_KNOTS('',3,(#9513,#9514,#9515,#9516,#9517,#9518,
#9519,#9520,#9521,#9522,#9523,#9524,#9525,#9526,#9527,#9528,#9529,#9530,
#9531,#9532,#9533,#9534),.UNSPECIFIED.,.F.,.F.,(4,3,3,3,3,3,3,4),(20.1593781767107,
20.9480992231686,21.9456277576052,22.9431562920418,23.9406848264784,24.938213360915,
25.9357418953516,26.4425634838903),.UNSPECIFIED.);
#153=B_SPLINE_CURVE_WITH_KNOTS('',3,(#9535,#9536,#9537,#9538,#9539,#9540,
#9541,#9542,#9543,#9544,#9545,#9546,#9547,#9548,#9549,#9550,#9551,#9552,
#9553,#9554,#9555,#9556),.UNSPECIFIED.,.F.,.F.,(4,3,3,3,3,3,3,4),(-22.695939185231,
-21.9456277576052,-20.9480992231686,-19.950570688732,-18.9530421542954,
-17.9555136198588,-16.9579850854222,-16.4127538780514),.UNSPECIFIED.);
#154=B_SPLINE_CURVE_WITH_KNOTS('',3,(#9561,#9562,#9563,#9564,#9565,#9566,
#9567,#9568,#9569,#9570,#9571,#9572,#9573,#9574,#9575,#9576,#9577,#9578,
#9579,#9580,#9581,#9582,#9583,#9584,#9585),.UNSPECIFIED.,.F.,.F.,(4,3,3,
3,3,3,3,3,4),(13.8761928695311,13.9653994821124,14.962928016549,15.9604565509856,
16.9579850854222,17.9555136198588,18.9530421542954,19.950570688732,20.1593781767107),
 .UNSPECIFIED.);
#155=B_SPLINE_CURVE_WITH_KNOTS('',3,(#9586,#9587,#9588,#9589,#9590,#9591,
#9592,#9593,#9594,#9595,#9596,#9597,#9598,#9599,#9600,#9601,#9602,#9603,
#9604,#9605,#9606,#9607),.UNSPECIFIED.,.F.,.F.,(4,3,3,3,3,3,3,4),(-16.4127538780514,
-15.9604565509856,-14.962928016549,-13.9653994821124,-12.9678709476758,
-11.9703424132392,-10.9728138788026,-10.1295685708718),.UNSPECIFIED.);
#156=B_SPLINE_CURVE_WITH_KNOTS('',3,(#9613,#9614,#9615,#9616,#9617,#9618,
#9619,#9620,#9621,#9622,#9623,#9624,#9625),.UNSPECIFIED.,.F.,.F.,(4,3,3,
3,4),(-3.84638326369226,-2.9925856033098,-1.9950570688732,-0.997528534436599,
0.),.UNSPECIFIED.);
#157=B_SPLINE_CURVE_WITH_KNOTS('',3,(#9628,#9629,#9630,#9631,#9632,#9633,
#9634,#9635,#9636,#9637,#9638,#9639,#9640,#9641,#9642,#9643,#9644,#9645,
#9646),.UNSPECIFIED.,.F.,.F.,(4,3,3,3,3,3,4),(2.01461286527441,2.99258560330979,
3.99011413774639,4.98764267218299,5.9851712066196,6.98269974105619,7.59300756235152),
 .UNSPECIFIED.);
#158=B_SPLINE_CURVE_WITH_KNOTS('',3,(#9652,#9653,#9654,#9655,#9656,#9657),
 .UNSPECIFIED.,.F.,.F.,(4,1,1,4),(109.955742875643,110.61690491348,111.614433447917,
112.611961982353),.UNSPECIFIED.);
#159=B_SPLINE_CURVE_WITH_KNOTS('',3,(#9660,#9661,#9662,#9663,#9664,#9665,
#9666),.UNSPECIFIED.,.F.,.F.,(4,1,1,1,4),(109.955742875643,110.16088031869,
111.158408853127,112.155937387564,113.133910125599),.UNSPECIFIED.);
#160=B_SPLINE_CURVE_WITH_KNOTS('',3,(#9671,#9672,#9673,#9674,#9675,#9676,
#9677,#9678,#9679,#9680),.UNSPECIFIED.,.F.,.F.,(4,1,1,1,1,1,1,4),(103.672557568463,
104.63173370686,105.629262241297,106.626790775734,107.62431931017,108.621847844607,
109.619376379043,109.955742875643),.UNSPECIFIED.);
#161=B_SPLINE_CURVE_WITH_KNOTS('',3,(#9681,#9682,#9683,#9684,#9685,#9686,
#9687,#9688,#9689,#9690),.UNSPECIFIED.,.F.,.F.,(4,1,1,1,1,1,1,4),(103.672557568463,
104.175709112071,105.173237646507,106.170766180944,107.168294715381,108.165823249817,
109.163351784254,109.955742875643),.UNSPECIFIED.);
#162=B_SPLINE_CURVE_WITH_KNOTS('',3,(#9695,#9696,#9697,#9698,#9699,#9700,
#9701,#9702,#9703,#9704,#9705),.UNSPECIFIED.,.F.,.F.,(4,1,1,1,1,1,1,1,4),
(97.3893722612836,97.6490339658042,98.6465625002408,99.6440910346774,100.641619569114,
101.639148103551,102.636676637987,103.634205172424,103.672557568463),
 .UNSPECIFIED.);
#163=B_SPLINE_CURVE_WITH_KNOTS('',3,(#9706,#9707,#9708,#9709,#9710,#9711,
#9712,#9713,#9714,#9715),.UNSPECIFIED.,.F.,.F.,(4,1,1,1,1,1,1,4),(97.3893722612836,
98.1905379054512,99.1880664398878,100.185594974324,101.183123508761,102.180652043198,
103.178180577634,103.672557568463),.UNSPECIFIED.);
#164=B_SPLINE_CURVE_WITH_KNOTS('',3,(#9720,#9721,#9722,#9723,#9724,#9725,
#9726,#9727,#9728,#9729),.UNSPECIFIED.,.F.,.F.,(4,1,1,1,1,1,1,4),(91.106186954104,
91.6638627591846,92.6613912936212,93.6589198280578,94.6564483624944,95.653976896931,
96.6515054313676,97.3893722612836),.UNSPECIFIED.);
#165=B_SPLINE_CURVE_WITH_KNOTS('',3,(#9730,#9731,#9732,#9733,#9734,#9735,
#9736,#9737,#9738,#9739,#9740),.UNSPECIFIED.,.F.,.F.,(4,1,1,1,1,1,1,1,4),
(91.106186954104,91.207838164395,92.2053666988316,93.2028952332682,94.2004237677048,
95.1979523021414,96.195480836578,97.1930093710146,97.3893722612836),
 .UNSPECIFIED.);
#166=B_SPLINE_CURVE_WITH_KNOTS('',3,(#9745,#9746,#9747,#9748,#9749,#9750,
#9751,#9752,#9753,#9754),.UNSPECIFIED.,.F.,.F.,(4,1,1,1,1,1,1,4),(84.8230016469244,
85.678691552565,86.6762200870016,87.6737486214382,88.6712771558748,89.6688056903114,
90.666334224748,91.106186954104),.UNSPECIFIED.);
#167=B_SPLINE_CURVE_WITH_KNOTS('',3,(#9755,#9756,#9757,#9758,#9759,#9760,
#9761,#9762,#9763,#9764),.UNSPECIFIED.,.F.,.F.,(4,1,1,1,1,1,1,4),(84.8230016469244,
85.2226669577754,86.220195492212,87.2177240266486,88.2152525610852,89.2127810955218,
90.2103096299584,91.106186954104),.UNSPECIFIED.);
#168=B_SPLINE_CURVE_WITH_KNOTS('',3,(#9769,#9770,#9771,#9772,#9773,#9774,
#9775,#9776,#9777,#9778,#9779),.UNSPECIFIED.,.F.,.F.,(4,1,1,1,1,1,1,1,4),
(78.5398163397448,78.6959918115088,79.6935203459454,80.691048880382,81.6885774148186,
82.6861059492552,83.6836344836918,84.6811630181284,84.8230016469244),
 .UNSPECIFIED.);
#169=B_SPLINE_CURVE_WITH_KNOTS('',3,(#9780,#9781,#9782,#9783,#9784,#9785,
#9786,#9787,#9788,#9789),.UNSPECIFIED.,.F.,.F.,(4,1,1,1,1,1,1,4),(78.5398163397448,
79.2374957511558,80.2350242855924,81.232552820029,82.2300813544656,83.2276098889022,
84.2251384233388,84.8230016469244),.UNSPECIFIED.);
#170=B_SPLINE_CURVE_WITH_KNOTS('',3,(#9794,#9795,#9796,#9797,#9798,#9799,
#9800,#9801,#9802,#9803),.UNSPECIFIED.,.F.,.F.,(4,1,1,1,1,1,1,4),(72.2566310325652,
72.7108206048892,73.7083491393258,74.7058776737624,75.703406208199,76.7009347426356,
77.6984632770722,78.5398163397448),.UNSPECIFIED.);
#171=B_SPLINE_CURVE_WITH_KNOTS('',3,(#9804,#9805,#9806,#9807,#9808,#9809,
#9810,#9811,#9812,#9813),.UNSPECIFIED.,.F.,.F.,(4,1,1,1,1,1,1,4),(72.2566310325652,
73.2523245445362,74.2498530789728,75.2473816134094,76.244910147846,77.2424386822826,
78.2399672167192,78.5398163397448),.UNSPECIFIED.);
#172=B_SPLINE_CURVE_WITH_KNOTS('',3,(#9818,#9819,#9820,#9821,#9822,#9823,
#9824,#9825,#9826,#9827),.UNSPECIFIED.,.F.,.F.,(4,1,1,1,1,1,1,4),(65.9734457253856,
66.7256493982696,67.7231779327062,68.7207064671428,69.7182350015794,70.715763536016,
71.7132920704526,72.2566310325652),.UNSPECIFIED.);
#173=B_SPLINE_CURVE_WITH_KNOTS('',3,(#9828,#9829,#9830,#9831,#9832,#9833,
#9834,#9835,#9836,#9837,#9838),.UNSPECIFIED.,.F.,.F.,(4,1,1,1,1,1,1,1,4),
(65.9734457253856,66.26962480348,67.2671533379167,68.2646818723532,69.2622104067898,
70.2597389412264,71.257267475663,72.2547960100996,72.2566310325652),
 .UNSPECIFIED.);
#174=B_SPLINE_CURVE_WITH_KNOTS('',3,(#9843,#9844,#9845,#9846,#9847,#9848,
#9849,#9850,#9851,#9852,#9853),.UNSPECIFIED.,.F.,.F.,(4,1,1,1,1,1,1,1,4),
(59.690260418206,59.7429496572134,60.74047819165,61.7380067260866,62.7355352605232,
63.7330637949598,64.7305923293964,65.728120863833,65.9734457253856),
 .UNSPECIFIED.);
#175=B_SPLINE_CURVE_WITH_KNOTS('',3,(#9854,#9855,#9856,#9857,#9858,#9859,
#9860,#9861,#9862,#9863),.UNSPECIFIED.,.F.,.F.,(4,1,1,1,1,1,1,4),(59.690260418206,
60.2844535968605,61.281982131297,62.2795106657336,63.2770392001703,64.2745677346068,
65.2720962690434,65.9734457253856),.UNSPECIFIED.);
#176=B_SPLINE_CURVE_WITH_KNOTS('',3,(#9868,#9869,#9870,#9871,#9872,#9873,
#9874,#9875,#9876,#9877),.UNSPECIFIED.,.F.,.F.,(4,1,1,1,1,1,1,4),(53.4070751110264,
53.7577784505938,54.7553069850304,55.752835519467,56.7503640539036,57.7478925883402,
58.7454211227768,59.690260418206),.UNSPECIFIED.);
#177=B_SPLINE_CURVE_WITH_KNOTS('',3,(#9878,#9879,#9880,#9881,#9882,#9883,
#9884,#9885,#9886,#9887),.UNSPECIFIED.,.F.,.F.,(4,1,1,1,1,1,1,4),(53.4070751110264,
54.2992823902409,55.2968109246775,56.294339459114,57.2918679935507,58.2893965279873,
59.2869250624238,59.690260418206),.UNSPECIFIED.);
#178=B_SPLINE_CURVE_WITH_KNOTS('',3,(#9892,#9893,#9894,#9895,#9896,#9897,
#9898,#9899,#9900,#9901),.UNSPECIFIED.,.F.,.F.,(4,1,1,1,1,1,1,4),(47.1238898038468,
47.7726072439742,48.7701357784108,49.7676643128474,50.765192847284,51.7627213817206,
52.7602499161572,53.4070751110264),.UNSPECIFIED.);
#179=B_SPLINE_CURVE_WITH_KNOTS('',3,(#9902,#9903,#9904,#9905,#9906,#9907,
#9908,#9909,#9910,#9911,#9912),.UNSPECIFIED.,.F.,.F.,(4,1,1,1,1,1,1,1,4),
(47.1238898038468,47.3165826491847,48.3141111836213,49.3116397180579,50.3091682524945,
51.3066967869311,52.3042253213677,53.3017538558043,53.4070751110264),
 .UNSPECIFIED.);
#180=B_SPLINE_CURVE_WITH_KNOTS('',3,(#9917,#9918,#9919,#9920,#9921,#9922,
#9923,#9924,#9925,#9926),.UNSPECIFIED.,.F.,.F.,(4,1,1,1,1,1,1,4),(40.8407044966673,
41.7874360373546,42.7849645717912,43.7824931062278,44.7800216406644,45.777550175101,
46.7750787095376,47.1238898038468),.UNSPECIFIED.);
#181=B_SPLINE_CURVE_WITH_KNOTS('',3,(#9927,#9928,#9929,#9930,#9931,#9932,
#9933,#9934,#9935,#9936),.UNSPECIFIED.,.F.,.F.,(4,1,1,1,1,1,1,4),(40.8407044966672,
41.3314114425651,42.3289399770017,43.3264685114383,44.3239970458749,45.3215255803115,
46.3190541147481,47.1238898038468),.UNSPECIFIED.);
#182=B_SPLINE_CURVE_WITH_KNOTS('',3,(#9941,#9942,#9943,#9944,#9945,#9946,
#9947,#9948,#9949,#9950,#9951),.UNSPECIFIED.,.F.,.F.,(4,1,1,1,1,1,1,1,4),
(34.5575191894876,34.8047362962984,35.802264830735,36.7997933651716,37.7973218996082,
38.7948504340448,39.7923789684814,40.789907502918,40.8407044966673),
 .UNSPECIFIED.);
#183=B_SPLINE_CURVE_WITH_KNOTS('',3,(#9952,#9953,#9954,#9955,#9956,#9957,
#9958,#9959,#9960,#9961),.UNSPECIFIED.,.F.,.F.,(4,1,1,1,1,1,1,4),(34.5575191894876,
35.3462402359455,36.3437687703821,37.3412973048187,38.3388258392553,39.3363543736919,
40.3338829081285,40.8407044966672),.UNSPECIFIED.);
#184=B_SPLINE_CURVE_WITH_KNOTS('',3,(#9966,#9967,#9968,#9969,#9970,#9971,
#9972,#9973,#9974,#9975),.UNSPECIFIED.,.F.,.F.,(4,1,1,1,1,1,1,4),(28.2743338823081,
28.8195650896788,29.8170936241154,30.814622158552,31.8121506929886,32.8096792274252,
33.8072077618618,34.5575191894876),.UNSPECIFIED.);
#185=B_SPLINE_CURVE_WITH_KNOTS('',3,(#9976,#9977,#9978,#9979,#9980,#9981,
#9982,#9983,#9984,#9985,#9986),.UNSPECIFIED.,.F.,.F.,(4,1,1,1,1,1,1,1,4),
(28.274333882308,28.3635404948893,29.3610690293259,30.3585975637625,31.3561260981991,
32.3536546326357,33.3511831670723,34.3487117015089,34.5575191894876),
 .UNSPECIFIED.);
#186=B_SPLINE_CURVE_WITH_KNOTS('',3,(#9991,#9992,#9993,#9994,#9995,#9996,
#9997,#9998,#9999,#10000),.UNSPECIFIED.,.F.,.F.,(4,1,1,1,1,1,1,4),(21.9911485751285,
22.8343938830592,23.8319224174958,24.8294509519324,25.826979486369,26.8245080208056,
27.8220365552422,28.2743338823081),.UNSPECIFIED.);
#187=B_SPLINE_CURVE_WITH_KNOTS('',3,(#10001,#10002,#10003,#10004,#10005,
#10006,#10007,#10008,#10009,#10010),.UNSPECIFIED.,.F.,.F.,(4,1,1,1,1,1,
1,4),(21.9911485751285,22.3783692882697,23.3758978227063,24.3734263571429,
25.3709548915795,26.3684834260161,27.3660119604527,28.274333882308),
 .UNSPECIFIED.);
#188=B_SPLINE_CURVE_WITH_KNOTS('',3,(#10016,#10017,#10018,#10019,#10020),
 .UNSPECIFIED.,.F.,.F.,(4,1,4),(14.3981410127769,15.3956695472135,15.7079632679489),
 .UNSPECIFIED.);
#189=B_SPLINE_CURVE_WITH_KNOTS('',3,(#10023,#10024,#10025,#10026,#10027),
 .UNSPECIFIED.,.F.,.F.,(4,1,4),(13.8761928695311,14.8541656075664,15.7079632679489),
 .UNSPECIFIED.);
#190=B_SPLINE_CURVE_WITH_KNOTS('',3,(#10033,#10034,#10035,#10036,#10037,
#10038,#10039,#10040,#10041,#10042,#10043,#10044,#10045,#10046,#10047,#10048,
#10049,#10050,#10051),.UNSPECIFIED.,.F.,.F.,(4,3,3,3,3,3,4),(95.5576018628658,
95.7627393059135,96.7602678403501,97.7577963747867,98.7553249092233,99.7528534436599,
100.750381978097),.UNSPECIFIED.);
#191=B_SPLINE_CURVE_WITH_KNOTS('',3,(#10055,#10056,#10057,#10058),
 .UNSPECIFIED.,.F.,.F.,(4,4),(-98.7357691128221,-98.0941628713861),
 .UNSPECIFIED.);
#192=B_SPLINE_CURVE_WITH_KNOTS('',3,(#10062,#10063,#10064,#10065,#10066,
#10067,#10068,#10069,#10070,#10071,#10072,#10073,#10074,#10075,#10076,#10077,
#10078,#10079,#10080,#10081,#10082,#10083),.UNSPECIFIED.,.F.,.F.,(4,3,3,
3,3,3,3,4),(-98.0941628713861,-97.7577963747867,-96.7602678403501,-95.7627393059135,
-94.7652107714769,-93.7676822370403,-92.7701537026037,-91.8109775642065),
 .UNSPECIFIED.);
#193=B_SPLINE_CURVE_WITH_KNOTS('',3,(#10088,#10089,#10090,#10091,#10092,
#10093,#10094,#10095,#10096,#10097,#10098,#10099,#10100,#10101,#10102,#10103,
#10104,#10105,#10106,#10107,#10108,#10109),.UNSPECIFIED.,.F.,.F.,(4,3,3,
3,3,3,3,4),(89.2744165556862,89.7775680992939,90.7750966337306,91.7726251681671,
92.7701537026037,93.7676822370403,94.7652107714769,95.5576018628658),
 .UNSPECIFIED.);
#194=B_SPLINE_CURVE_WITH_KNOTS('',3,(#10110,#10111,#10112,#10113,#10114,
#10115,#10116,#10117,#10118,#10119,#10120,#10121,#10122,#10123,#10124,#10125,
#10126,#10127,#10128,#10129,#10130,#10131,#10132,#10133,#10134),
 .UNSPECIFIED.,.F.,.F.,(4,3,3,3,3,3,3,3,4),(-91.8109775642065,-91.7726251681671,
-90.7750966337305,-89.7775680992939,-88.7800395648573,-87.7825110304207,
-86.7849824959842,-85.7874539615476,-85.5277922570269),.UNSPECIFIED.);
#195=B_SPLINE_CURVE_WITH_KNOTS('',3,(#10139,#10140,#10141,#10142,#10143,
#10144,#10145,#10146,#10147,#10148,#10149,#10150,#10151,#10152,#10153,#10154,
#10155,#10156,#10157,#10158,#10159,#10160),.UNSPECIFIED.,.F.,.F.,(4,3,3,
3,3,3,3,4),(82.9912312485066,83.7923968926743,84.7899254271109,85.7874539615476,
86.7849824959841,87.7825110304207,88.7800395648573,89.2744165556862),
 .UNSPECIFIED.);
#196=B_SPLINE_CURVE_WITH_KNOTS('',3,(#10161,#10162,#10163,#10164,#10165,
#10166,#10167,#10168,#10169,#10170,#10171,#10172,#10173,#10174,#10175,#10176,
#10177,#10178,#10179,#10180,#10181,#10182),.UNSPECIFIED.,.F.,.F.,(4,3,3,
3,3,3,3,4),(-85.5277922570269,-84.789925427111,-83.7923968926743,-82.7948683582377,
-81.7973398238011,-80.7998112893646,-79.8022827549279,-79.2446069498473),
 .UNSPECIFIED.);
#197=B_SPLINE_CURVE_WITH_KNOTS('',3,(#10187,#10188,#10189,#10190,#10191,
#10192,#10193,#10194,#10195,#10196,#10197,#10198,#10199,#10200,#10201,#10202,
#10203,#10204,#10205,#10206,#10207,#10208,#10209,#10210,#10211),
 .UNSPECIFIED.,.F.,.F.,(4,3,3,3,3,3,3,3,4),(76.708045941327,76.8096971516181,
77.8072256860547,78.8047542204914,79.8022827549279,80.7998112893646,81.7973398238011,
82.7948683582377,82.9912312485066),.UNSPECIFIED.);
#198=B_SPLINE_CURVE_WITH_KNOTS('',3,(#10212,#10213,#10214,#10215,#10216,
#10217,#10218,#10219,#10220,#10221,#10222,#10223,#10224,#10225,#10226,#10227,
#10228,#10229,#10230,#10231,#10232,#10233),.UNSPECIFIED.,.F.,.F.,(4,3,3,
3,3,3,3,4),(-79.2446069498473,-78.8047542204913,-77.8072256860547,-76.8096971516181,
-75.8121686171815,-74.8146400827449,-73.8171115483083,-72.9614216426677),
 .UNSPECIFIED.);
#199=B_SPLINE_CURVE_WITH_KNOTS('',3,(#10238,#10239,#10240,#10241,#10242,
#10243,#10244,#10245,#10246,#10247,#10248,#10249,#10250,#10251,#10252,#10253,
#10254,#10255,#10256,#10257,#10258,#10259),.UNSPECIFIED.,.F.,.F.,(4,3,3,
3,3,3,3,4),(70.4248606341474,70.8245259449985,71.8220544794352,72.8195830138717,
73.8171115483084,74.8146400827449,75.8121686171816,76.708045941327),
 .UNSPECIFIED.);
#200=B_SPLINE_CURVE_WITH_KNOTS('',3,(#10260,#10261,#10262,#10263,#10264,
#10265,#10266,#10267,#10268,#10269,#10270,#10271,#10272,#10273,#10274,#10275,
#10276,#10277,#10278,#10279,#10280,#10281,#10282,#10283,#10284),
 .UNSPECIFIED.,.F.,.F.,(4,3,3,3,3,3,3,3,4),(-72.9614216426677,-72.8195830138717,
-71.8220544794352,-70.8245259449986,-69.8269974105619,-68.8294688761253,
-67.8319403416887,-66.8344118072522,-66.6782363354881),.UNSPECIFIED.);
#201=B_SPLINE_CURVE_WITH_KNOTS('',3,(#10289,#10290,#10291,#10292,#10293,
#10294,#10295,#10296,#10297,#10298,#10299,#10300,#10301,#10302,#10303,#10304,
#10305,#10306,#10307,#10308,#10309,#10310),.UNSPECIFIED.,.F.,.F.,(4,3,3,
3,3,3,3,4),(64.1416753269678,64.839354738379,65.8368832728156,66.8344118072522,
67.8319403416887,68.8294688761253,69.8269974105619,70.4248606341474),
 .UNSPECIFIED.);
#202=B_SPLINE_CURVE_WITH_KNOTS('',3,(#10311,#10312,#10313,#10314,#10315,
#10316,#10317,#10318,#10319,#10320,#10321,#10322,#10323,#10324,#10325,#10326,
#10327,#10328,#10329,#10330,#10331,#10332),.UNSPECIFIED.,.F.,.F.,(4,3,3,
3,3,3,3,4),(-66.6782363354881,-65.8368832728156,-64.839354738379,-63.8418262039424,
-62.8442976695058,-61.8467691350692,-60.8492406006326,-60.3950510283086),
 .UNSPECIFIED.);
#203=B_SPLINE_CURVE_WITH_KNOTS('',3,(#10337,#10338,#10339,#10340,#10341,
#10342,#10343,#10344,#10345,#10346,#10347,#10348,#10349,#10350,#10351,#10352,
#10353,#10354,#10355,#10356,#10357,#10358),.UNSPECIFIED.,.F.,.F.,(4,3,3,
3,3,3,3,4),(57.8584900197882,58.8541835317594,59.851712066196,60.8492406006326,
61.8467691350692,62.8442976695058,63.8418262039424,64.1416753269678),
 .UNSPECIFIED.);
#204=B_SPLINE_CURVE_WITH_KNOTS('',3,(#10359,#10360,#10361,#10362,#10363,
#10364,#10365,#10366,#10367,#10368,#10369,#10370,#10371,#10372,#10373,#10374,
#10375,#10376,#10377,#10378,#10379,#10380),.UNSPECIFIED.,.F.,.F.,(4,3,3,
3,3,3,3,4),(-60.3950510283086,-59.851712066196,-58.8541835317594,-57.8566549973228,
-56.8591264628862,-55.8615979284496,-54.864069394013,-54.111865721129),
 .UNSPECIFIED.);
#205=B_SPLINE_CURVE_WITH_KNOTS('',3,(#10385,#10386,#10387,#10388,#10389,
#10390,#10391,#10392,#10393,#10394,#10395,#10396,#10397,#10398,#10399,#10400,
#10401,#10402,#10403,#10404,#10405,#10406),.UNSPECIFIED.,.F.,.F.,(4,3,3,
3,3,3,3,4),(51.5753047126086,51.8714837907032,52.8690123251398,53.8665408595764,
54.864069394013,55.8615979284496,56.8591264628862,57.8584900197882),
 .UNSPECIFIED.);
#206=B_SPLINE_CURVE_WITH_KNOTS('',3,(#10407,#10408,#10409,#10410,#10411,
#10412,#10413,#10414,#10415,#10416,#10417,#10418,#10419,#10420,#10421,#10422,
#10423,#10424,#10425,#10426,#10427,#10428,#10429,#10430,#10431),
 .UNSPECIFIED.,.F.,.F.,(4,3,3,3,3,3,3,3,4),(-54.111865721129,-53.8665408595764,
-52.8690123251398,-51.8714837907032,-50.8739552562666,-49.87642672183,-48.8788981873934,
-47.8813696529568,-47.8286804139494),.UNSPECIFIED.);
#207=B_SPLINE_CURVE_WITH_KNOTS('',3,(#10436,#10437,#10438,#10439,#10440,
#10441,#10442,#10443,#10444,#10445,#10446,#10447,#10448,#10449,#10450,#10451,
#10452,#10453,#10454,#10455,#10456,#10457),.UNSPECIFIED.,.F.,.F.,(4,3,3,
3,3,3,3,4),(45.2921194054291,45.8863125840836,46.8838411185202,47.8813696529568,
48.8788981873934,49.87642672183,50.8739552562666,51.5753047126086),
 .UNSPECIFIED.);
#208=B_SPLINE_CURVE_WITH_KNOTS('',3,(#10458,#10459,#10460,#10461,#10462,
#10463,#10464,#10465,#10466,#10467,#10468,#10469,#10470,#10471,#10472,#10473,
#10474,#10475,#10476,#10477,#10478,#10479),.UNSPECIFIED.,.F.,.F.,(4,3,3,
3,3,3,3,4),(-47.8286804139494,-46.8838411185202,-45.8863125840836,-44.888784049647,
-43.8912555152104,-42.8937269807738,-41.8961984463372,-41.5454951067698),
 .UNSPECIFIED.);
#209=B_SPLINE_CURVE_WITH_KNOTS('',3,(#10484,#10485,#10486,#10487,#10488,
#10489,#10490,#10491,#10492,#10493,#10494,#10495,#10496,#10497,#10498,#10499,
#10500,#10501,#10502,#10503,#10504,#10505),.UNSPECIFIED.,.F.,.F.,(4,3,3,
3,3,3,3,4),(39.0089340982495,39.901141377464,40.8986699119006,41.8961984463372,
42.8937269807738,43.8912555152104,44.888784049647,45.2921194054291),
 .UNSPECIFIED.);
#210=B_SPLINE_CURVE_WITH_KNOTS('',3,(#10506,#10507,#10508,#10509,#10510,
#10511,#10512,#10513,#10514,#10515,#10516,#10517,#10518,#10519,#10520,#10521,
#10522,#10523,#10524,#10525,#10526,#10527),.UNSPECIFIED.,.F.,.F.,(4,3,3,
3,3,3,3,4),(-41.5454951067698,-40.8986699119006,-39.901141377464,-38.9036128430274,
-37.9060843085908,-36.9085557741542,-35.9110272397176,-35.2623097995902),
 .UNSPECIFIED.);
#211=B_SPLINE_CURVE_WITH_KNOTS('',3,(#10532,#10533,#10534,#10535,#10536,
#10537,#10538,#10539,#10540,#10541,#10542,#10543,#10544,#10545,#10546,#10547,
#10548,#10549,#10550,#10551,#10552,#10553,#10554,#10555,#10556),
 .UNSPECIFIED.,.F.,.F.,(4,3,3,3,3,3,3,3,4),(32.7257487910699,32.9184416364078,
33.9159701708444,34.913498705281,35.9110272397176,36.9085557741542,37.9060843085908,
38.9036128430274,39.0089340982495),.UNSPECIFIED.);
#212=B_SPLINE_CURVE_WITH_KNOTS('',3,(#10557,#10558,#10559,#10560,#10561,
#10562,#10563,#10564,#10565,#10566,#10567,#10568,#10569,#10570,#10571,#10572,
#10573,#10574,#10575,#10576,#10577,#10578),.UNSPECIFIED.,.F.,.F.,(4,3,3,
3,3,3,3,4),(-35.2623097995902,-34.913498705281,-33.9159701708444,-32.9184416364078,
-31.9209131019712,-30.9233845675346,-29.925856033098,-28.9791244924106),
 .UNSPECIFIED.);
#213=B_SPLINE_CURVE_WITH_KNOTS('',3,(#10583,#10584,#10585,#10586,#10587,
#10588,#10589,#10590,#10591,#10592,#10593,#10594,#10595,#10596,#10597,#10598,
#10599,#10600,#10601,#10602,#10603,#10604),.UNSPECIFIED.,.F.,.F.,(4,3,3,
3,3,3,3,4),(26.4425634838903,26.9332704297882,27.9307989642248,28.9283274986614,
29.925856033098,30.9233845675346,31.9209131019712,32.7257487910699),
 .UNSPECIFIED.);
#214=B_SPLINE_CURVE_WITH_KNOTS('',3,(#10605,#10606,#10607,#10608,#10609,
#10610,#10611,#10612,#10613,#10614,#10615,#10616,#10617,#10618,#10619,#10620,
#10621,#10622,#10623,#10624,#10625,#10626,#10627,#10628,#10629),
 .UNSPECIFIED.,.F.,.F.,(4,3,3,3,3,3,3,3,4),(-28.9791244924106,-28.9283274986614,
-27.9307989642248,-26.9332704297882,-25.9357418953516,-24.938213360915,
-23.9406848264784,-22.9431562920418,-22.695939185231),.UNSPECIFIED.);
#215=B_SPLINE_CURVE_WITH_KNOTS('',3,(#10634,#10635,#10636,#10637,#10638,
#10639,#10640,#10641,#10642,#10643,#10644,#10645,#10646,#10647,#10648,#10649,
#10650,#10651,#10652,#10653,#10654,#10655),.UNSPECIFIED.,.F.,.F.,(4,3,3,
3,3,3,3,4),(20.1593781767107,20.9480992231686,21.9456277576052,22.9431562920418,
23.9406848264784,24.938213360915,25.9357418953516,26.4425634838903),
 .UNSPECIFIED.);
#216=B_SPLINE_CURVE_WITH_KNOTS('',3,(#10656,#10657,#10658,#10659,#10660,
#10661,#10662,#10663,#10664,#10665,#10666,#10667,#10668,#10669,#10670,#10671,
#10672,#10673,#10674,#10675,#10676,#10677),.UNSPECIFIED.,.F.,.F.,(4,3,3,
3,3,3,3,4),(-22.695939185231,-21.9456277576052,-20.9480992231686,-19.950570688732,
-18.9530421542954,-17.9555136198588,-16.9579850854222,-16.4127538780514),
 .UNSPECIFIED.);
#217=B_SPLINE_CURVE_WITH_KNOTS('',3,(#10682,#10683,#10684,#10685,#10686,
#10687,#10688,#10689,#10690,#10691,#10692,#10693,#10694,#10695,#10696,#10697,
#10698,#10699,#10700,#10701,#10702,#10703,#10704,#10705,#10706),
 .UNSPECIFIED.,.F.,.F.,(4,3,3,3,3,3,3,3,4),(13.8761928695311,13.9653994821124,
14.962928016549,15.9604565509856,16.9579850854222,17.9555136198588,18.9530421542954,
19.950570688732,20.1593781767107),.UNSPECIFIED.);
#218=B_SPLINE_CURVE_WITH_KNOTS('',3,(#10707,#10708,#10709,#10710,#10711,
#10712,#10713,#10714,#10715,#10716,#10717,#10718,#10719,#10720,#10721,#10722,
#10723,#10724,#10725,#10726,#10727,#10728),.UNSPECIFIED.,.F.,.F.,(4,3,3,
3,3,3,3,4),(-16.4127538780514,-15.9604565509856,-14.962928016549,-13.9653994821124,
-12.9678709476758,-11.9703424132392,-10.9728138788026,-10.1295685708718),
 .UNSPECIFIED.);
#219=B_SPLINE_CURVE_WITH_KNOTS('',3,(#10734,#10735,#10736,#10737,#10738,
#10739,#10740,#10741,#10742,#10743,#10744,#10745,#10746),.UNSPECIFIED.,
 .F.,.F.,(4,3,3,3,4),(-3.84638326369226,-2.9925856033098,-1.9950570688732,
-0.997528534436599,0.),.UNSPECIFIED.);
#220=B_SPLINE_CURVE_WITH_KNOTS('',3,(#10749,#10750,#10751,#10752,#10753,
#10754,#10755,#10756,#10757,#10758,#10759,#10760,#10761,#10762,#10763,#10764,
#10765,#10766,#10767),.UNSPECIFIED.,.F.,.F.,(4,3,3,3,3,3,4),(2.01461286527441,
2.99258560330979,3.99011413774639,4.98764267218299,5.9851712066196,6.98269974105619,
7.59300756235152),.UNSPECIFIED.);
#221=B_SPLINE_CURVE_WITH_KNOTS('',3,(#10773,#10774,#10775,#10776,#10777,
#10778),.UNSPECIFIED.,.F.,.F.,(4,1,1,4),(109.955742875643,110.61690491348,
111.614433447917,112.611961982353),.UNSPECIFIED.);
#222=B_SPLINE_CURVE_WITH_KNOTS('',3,(#10781,#10782,#10783,#10784,#10785,
#10786,#10787),.UNSPECIFIED.,.F.,.F.,(4,1,1,1,4),(109.955742875643,110.16088031869,
111.158408853127,112.155937387564,113.133910125599),.UNSPECIFIED.);
#223=B_SPLINE_CURVE_WITH_KNOTS('',3,(#10792,#10793,#10794,#10795,#10796,
#10797,#10798,#10799,#10800,#10801),.UNSPECIFIED.,.F.,.F.,(4,1,1,1,1,1,
1,4),(103.672557568463,104.63173370686,105.629262241297,106.626790775734,
107.62431931017,108.621847844607,109.619376379043,109.955742875643),
 .UNSPECIFIED.);
#224=B_SPLINE_CURVE_WITH_KNOTS('',3,(#10802,#10803,#10804,#10805,#10806,
#10807,#10808,#10809,#10810,#10811),.UNSPECIFIED.,.F.,.F.,(4,1,1,1,1,1,
1,4),(103.672557568463,104.175709112071,105.173237646507,106.170766180944,
107.168294715381,108.165823249817,109.163351784254,109.955742875643),
 .UNSPECIFIED.);
#225=B_SPLINE_CURVE_WITH_KNOTS('',3,(#10816,#10817,#10818,#10819,#10820,
#10821,#10822,#10823,#10824,#10825,#10826),.UNSPECIFIED.,.F.,.F.,(4,1,1,
1,1,1,1,1,4),(97.3893722612836,97.6490339658042,98.6465625002408,99.6440910346774,
100.641619569114,101.639148103551,102.636676637987,103.634205172424,103.672557568463),
 .UNSPECIFIED.);
#226=B_SPLINE_CURVE_WITH_KNOTS('',3,(#10827,#10828,#10829,#10830,#10831,
#10832,#10833,#10834,#10835,#10836),.UNSPECIFIED.,.F.,.F.,(4,1,1,1,1,1,
1,4),(97.3893722612836,98.1905379054512,99.1880664398878,100.185594974324,
101.183123508761,102.180652043198,103.178180577634,103.672557568463),
 .UNSPECIFIED.);
#227=B_SPLINE_CURVE_WITH_KNOTS('',3,(#10841,#10842,#10843,#10844,#10845,
#10846,#10847,#10848,#10849,#10850),.UNSPECIFIED.,.F.,.F.,(4,1,1,1,1,1,
1,4),(91.106186954104,91.6638627591846,92.6613912936212,93.6589198280578,
94.6564483624944,95.653976896931,96.6515054313676,97.3893722612836),
 .UNSPECIFIED.);
#228=B_SPLINE_CURVE_WITH_KNOTS('',3,(#10851,#10852,#10853,#10854,#10855,
#10856,#10857,#10858,#10859,#10860,#10861),.UNSPECIFIED.,.F.,.F.,(4,1,1,
1,1,1,1,1,4),(91.106186954104,91.207838164395,92.2053666988316,93.2028952332682,
94.2004237677048,95.1979523021414,96.195480836578,97.1930093710146,97.3893722612836),
 .UNSPECIFIED.);
#229=B_SPLINE_CURVE_WITH_KNOTS('',3,(#10866,#10867,#10868,#10869,#10870,
#10871,#10872,#10873,#10874,#10875),.UNSPECIFIED.,.F.,.F.,(4,1,1,1,1,1,
1,4),(84.8230016469244,85.678691552565,86.6762200870016,87.6737486214382,
88.6712771558748,89.6688056903114,90.666334224748,91.106186954104),
 .UNSPECIFIED.);
#230=B_SPLINE_CURVE_WITH_KNOTS('',3,(#10876,#10877,#10878,#10879,#10880,
#10881,#10882,#10883,#10884,#10885),.UNSPECIFIED.,.F.,.F.,(4,1,1,1,1,1,
1,4),(84.8230016469244,85.2226669577754,86.220195492212,87.2177240266486,
88.2152525610852,89.2127810955218,90.2103096299584,91.106186954104),
 .UNSPECIFIED.);
#231=B_SPLINE_CURVE_WITH_KNOTS('',3,(#10890,#10891,#10892,#10893,#10894,
#10895,#10896,#10897,#10898,#10899,#10900),.UNSPECIFIED.,.F.,.F.,(4,1,1,
1,1,1,1,1,4),(78.5398163397448,78.6959918115088,79.6935203459454,80.691048880382,
81.6885774148186,82.6861059492552,83.6836344836918,84.6811630181284,84.8230016469244),
 .UNSPECIFIED.);
#232=B_SPLINE_CURVE_WITH_KNOTS('',3,(#10901,#10902,#10903,#10904,#10905,
#10906,#10907,#10908,#10909,#10910),.UNSPECIFIED.,.F.,.F.,(4,1,1,1,1,1,
1,4),(78.5398163397448,79.2374957511558,80.2350242855924,81.232552820029,
82.2300813544656,83.2276098889022,84.2251384233388,84.8230016469244),
 .UNSPECIFIED.);
#233=B_SPLINE_CURVE_WITH_KNOTS('',3,(#10915,#10916,#10917,#10918,#10919,
#10920,#10921,#10922,#10923,#10924),.UNSPECIFIED.,.F.,.F.,(4,1,1,1,1,1,
1,4),(72.2566310325652,72.7108206048892,73.7083491393258,74.7058776737624,
75.703406208199,76.7009347426356,77.6984632770722,78.5398163397448),
 .UNSPECIFIED.);
#234=B_SPLINE_CURVE_WITH_KNOTS('',3,(#10925,#10926,#10927,#10928,#10929,
#10930,#10931,#10932,#10933,#10934),.UNSPECIFIED.,.F.,.F.,(4,1,1,1,1,1,
1,4),(72.2566310325652,73.2523245445362,74.2498530789728,75.2473816134094,
76.244910147846,77.2424386822826,78.2399672167192,78.5398163397448),
 .UNSPECIFIED.);
#235=B_SPLINE_CURVE_WITH_KNOTS('',3,(#10939,#10940,#10941,#10942,#10943,
#10944,#10945,#10946,#10947,#10948),.UNSPECIFIED.,.F.,.F.,(4,1,1,1,1,1,
1,4),(65.9734457253856,66.7256493982696,67.7231779327062,68.7207064671428,
69.7182350015794,70.715763536016,71.7132920704526,72.2566310325652),
 .UNSPECIFIED.);
#236=B_SPLINE_CURVE_WITH_KNOTS('',3,(#10949,#10950,#10951,#10952,#10953,
#10954,#10955,#10956,#10957,#10958,#10959),.UNSPECIFIED.,.F.,.F.,(4,1,1,
1,1,1,1,1,4),(65.9734457253856,66.26962480348,67.2671533379167,68.2646818723532,
69.2622104067898,70.2597389412264,71.257267475663,72.2547960100996,72.2566310325652),
 .UNSPECIFIED.);
#237=B_SPLINE_CURVE_WITH_KNOTS('',3,(#10964,#10965,#10966,#10967,#10968,
#10969,#10970,#10971,#10972,#10973,#10974),.UNSPECIFIED.,.F.,.F.,(4,1,1,
1,1,1,1,1,4),(59.690260418206,59.7429496572134,60.74047819165,61.7380067260866,
62.7355352605232,63.7330637949598,64.7305923293964,65.728120863833,65.9734457253856),
 .UNSPECIFIED.);
#238=B_SPLINE_CURVE_WITH_KNOTS('',3,(#10975,#10976,#10977,#10978,#10979,
#10980,#10981,#10982,#10983,#10984),.UNSPECIFIED.,.F.,.F.,(4,1,1,1,1,1,
1,4),(59.690260418206,60.2844535968605,61.281982131297,62.2795106657336,
63.2770392001703,64.2745677346068,65.2720962690434,65.9734457253856),
 .UNSPECIFIED.);
#239=B_SPLINE_CURVE_WITH_KNOTS('',3,(#10989,#10990,#10991,#10992,#10993,
#10994,#10995,#10996,#10997,#10998),.UNSPECIFIED.,.F.,.F.,(4,1,1,1,1,1,
1,4),(53.4070751110264,53.7577784505938,54.7553069850304,55.752835519467,
56.7503640539036,57.7478925883402,58.7454211227768,59.690260418206),
 .UNSPECIFIED.);
#240=B_SPLINE_CURVE_WITH_KNOTS('',3,(#10999,#11000,#11001,#11002,#11003,
#11004,#11005,#11006,#11007,#11008),.UNSPECIFIED.,.F.,.F.,(4,1,1,1,1,1,
1,4),(53.4070751110264,54.2992823902409,55.2968109246775,56.294339459114,
57.2918679935507,58.2893965279873,59.2869250624238,59.690260418206),
 .UNSPECIFIED.);
#241=B_SPLINE_CURVE_WITH_KNOTS('',3,(#11013,#11014,#11015,#11016,#11017,
#11018,#11019,#11020,#11021,#11022),.UNSPECIFIED.,.F.,.F.,(4,1,1,1,1,1,
1,4),(47.1238898038468,47.7726072439742,48.7701357784108,49.7676643128474,
50.765192847284,51.7627213817206,52.7602499161572,53.4070751110264),
 .UNSPECIFIED.);
#242=B_SPLINE_CURVE_WITH_KNOTS('',3,(#11023,#11024,#11025,#11026,#11027,
#11028,#11029,#11030,#11031,#11032,#11033),.UNSPECIFIED.,.F.,.F.,(4,1,1,
1,1,1,1,1,4),(47.1238898038468,47.3165826491847,48.3141111836213,49.3116397180579,
50.3091682524945,51.3066967869311,52.3042253213677,53.3017538558043,53.4070751110264),
 .UNSPECIFIED.);
#243=B_SPLINE_CURVE_WITH_KNOTS('',3,(#11038,#11039,#11040,#11041,#11042,
#11043,#11044,#11045,#11046,#11047),.UNSPECIFIED.,.F.,.F.,(4,1,1,1,1,1,
1,4),(40.8407044966673,41.7874360373546,42.7849645717912,43.7824931062278,
44.7800216406644,45.777550175101,46.7750787095376,47.1238898038468),
 .UNSPECIFIED.);
#244=B_SPLINE_CURVE_WITH_KNOTS('',3,(#11048,#11049,#11050,#11051,#11052,
#11053,#11054,#11055,#11056,#11057),.UNSPECIFIED.,.F.,.F.,(4,1,1,1,1,1,
1,4),(40.8407044966672,41.3314114425651,42.3289399770017,43.3264685114383,
44.3239970458749,45.3215255803115,46.3190541147481,47.1238898038468),
 .UNSPECIFIED.);
#245=B_SPLINE_CURVE_WITH_KNOTS('',3,(#11062,#11063,#11064,#11065,#11066,
#11067,#11068,#11069,#11070,#11071,#11072),.UNSPECIFIED.,.F.,.F.,(4,1,1,
1,1,1,1,1,4),(34.5575191894876,34.8047362962984,35.802264830735,36.7997933651716,
37.7973218996082,38.7948504340448,39.7923789684814,40.789907502918,40.8407044966673),
 .UNSPECIFIED.);
#246=B_SPLINE_CURVE_WITH_KNOTS('',3,(#11073,#11074,#11075,#11076,#11077,
#11078,#11079,#11080,#11081,#11082),.UNSPECIFIED.,.F.,.F.,(4,1,1,1,1,1,
1,4),(34.5575191894876,35.3462402359455,36.3437687703821,37.3412973048187,
38.3388258392553,39.3363543736919,40.3338829081285,40.8407044966672),
 .UNSPECIFIED.);
#247=B_SPLINE_CURVE_WITH_KNOTS('',3,(#11087,#11088,#11089,#11090,#11091,
#11092,#11093,#11094,#11095,#11096),.UNSPECIFIED.,.F.,.F.,(4,1,1,1,1,1,
1,4),(28.2743338823081,28.8195650896788,29.8170936241154,30.814622158552,
31.8121506929886,32.8096792274252,33.8072077618618,34.5575191894876),
 .UNSPECIFIED.);
#248=B_SPLINE_CURVE_WITH_KNOTS('',3,(#11097,#11098,#11099,#11100,#11101,
#11102,#11103,#11104,#11105,#11106,#11107),.UNSPECIFIED.,.F.,.F.,(4,1,1,
1,1,1,1,1,4),(28.274333882308,28.3635404948893,29.3610690293259,30.3585975637625,
31.3561260981991,32.3536546326357,33.3511831670723,34.3487117015089,34.5575191894876),
 .UNSPECIFIED.);
#249=B_SPLINE_CURVE_WITH_KNOTS('',3,(#11112,#11113,#11114,#11115,#11116,
#11117,#11118,#11119,#11120,#11121),.UNSPECIFIED.,.F.,.F.,(4,1,1,1,1,1,
1,4),(21.9911485751285,22.8343938830592,23.8319224174958,24.8294509519324,
25.826979486369,26.8245080208056,27.8220365552422,28.2743338823081),
 .UNSPECIFIED.);
#250=B_SPLINE_CURVE_WITH_KNOTS('',3,(#11122,#11123,#11124,#11125,#11126,
#11127,#11128,#11129,#11130,#11131),.UNSPECIFIED.,.F.,.F.,(4,1,1,1,1,1,
1,4),(21.9911485751285,22.3783692882697,23.3758978227063,24.3734263571429,
25.3709548915795,26.3684834260161,27.3660119604527,28.274333882308),
 .UNSPECIFIED.);
#251=B_SPLINE_CURVE_WITH_KNOTS('',3,(#11137,#11138,#11139,#11140,#11141),
 .UNSPECIFIED.,.F.,.F.,(4,1,4),(14.3981410127769,15.3956695472135,15.7079632679489),
 .UNSPECIFIED.);
#252=B_SPLINE_CURVE_WITH_KNOTS('',3,(#11144,#11145,#11146,#11147,#11148),
 .UNSPECIFIED.,.F.,.F.,(4,1,4),(13.8761928695311,14.8541656075664,15.7079632679489),
 .UNSPECIFIED.);
#253=B_SPLINE_CURVE_WITH_KNOTS('',3,(#11150,#11151,#11152,#11153,#11154,
#11155,#11156,#11157,#11158,#11159,#11160,#11161,#11162,#11163,#11164,#11165,
#11166,#11167,#11168,#11169,#11170,#11171,#11172,#11173,#11174,#11175,#11176,
#11177,#11178,#11179,#11180,#11181,#11182,#11183,#11184,#11185,#11186,#11187,
#11188,#11189,#11190,#11191,#11192,#11193,#11194,#11195,#11196,#11197,#11198,
#11199,#11200,#11201,#11202,#11203,#11204,#11205,#11206,#11207,#11208,#11209,
#11210,#11211,#11212,#11213,#11214,#11215,#11216,#11217,#11218,#11219,#11220,
#11221,#11222,#11223,#11224,#11225,#11226,#11227,#11228,#11229,#11230,#11231,
#11232,#11233,#11234,#11235,#11236,#11237),.UNSPECIFIED.,.F.,.F.,(4,3,3,
3,3,3,3,3,3,3,3,3,3,3,3,3,3,3,3,3,3,3,3,3,3,3,3,3,3,4),(-0.378621596831286,
-0.35979753708714,-0.347859687182163,-0.339722489331693,-0.33538424950682,
-0.315512590853311,-0.301178211065556,-0.297261960366015,-0.293227388694864,
-0.272825172423111,-0.252127510483728,-0.239305021000613,-0.228805794178289,
-0.224505212292546,-0.203200653905749,-0.200837552551268,-0.18035021613173,
-0.158310724015752,-0.15433010633306,-0.150809400457636,-0.129426099231333,
-0.10759191519814,-0.0856252932872589,-0.0802029863915961,-0.0759441290511527,
-0.053396549390214,-0.0308243813684254,-0.00876573827391309,-0.00403427920390719,
0.),.UNSPECIFIED.);
#254=B_SPLINE_CURVE_WITH_KNOTS('',3,(#11238,#11239,#11240,#11241,#11242,
#11243,#11244,#11245,#11246,#11247,#11248,#11249,#11250,#11251,#11252,#11253,
#11254,#11255,#11256,#11257,#11258,#11259,#11260,#11261,#11262,#11263,#11264,
#11265,#11266,#11267,#11268,#11269,#11270,#11271,#11272,#11273,#11274,#11275,
#11276,#11277,#11278,#11279,#11280,#11281,#11282,#11283,#11284,#11285,#11286,
#11287,#11288,#11289,#11290,#11291,#11292,#11293,#11294,#11295,#11296,#11297,
#11298,#11299,#11300,#11301,#11302,#11303,#11304,#11305,#11306,#11307,#11308,
#11309,#11310,#11311,#11312,#11313,#11314,#11315,#11316,#11317,#11318,#11319,
#11320,#11321,#11322),.UNSPECIFIED.,.F.,.F.,(4,3,3,3,3,3,3,3,3,3,3,3,3,
3,3,3,3,3,3,3,3,3,3,3,3,3,3,3,4),(-0.37694081721167,-0.354634302100723,
-0.332912872548166,-0.328064580792288,-0.305815981116835,-0.290196841687263,
-0.284261051704666,-0.278600436316194,-0.256917265324022,-0.235699702105988,
-0.21494747804995,-0.20819720640224,-0.204402057236322,-0.183825922858711,
-0.180862865680265,-0.159880209104345,-0.140305785739984,-0.136021305575262,
-0.132587894912548,-0.11212857689637,-0.091763985715855,-0.0718357358806271,
-0.0676216261694051,-0.0636601282916112,-0.044102241112633,-0.0249163068456578,
-0.00635333976700777,-0.00328482218945702,0.),.UNSPECIFIED.);
#255=B_SPLINE_CURVE_WITH_KNOTS('',3,(#11324,#11325,#11326,#11327,#11328,
#11329,#11330,#11331,#11332,#11333,#11334),.UNSPECIFIED.,.F.,.F.,(4,1,1,
1,1,1,1,1,4),(15.7079632679489,15.851694142003,16.8492226764396,17.8467512108762,
18.8442797453128,19.8418082797494,20.839336814186,21.8368653486226,21.9911485751285),
 .UNSPECIFIED.);
#256=B_SPLINE_CURVE_WITH_KNOTS('',3,(#11335,#11336,#11337,#11338,#11339,
#11340,#11341,#11342,#11343,#11344),.UNSPECIFIED.,.F.,.F.,(4,1,1,1,1,1,
1,4),(15.7079632679489,16.3931980816501,17.3907266160867,18.3882551505233,
19.3857836849599,20.3833122193965,21.3808407538331,21.9911485751285),
 .UNSPECIFIED.);
#257=B_SPLINE_CURVE_WITH_KNOTS('',3,(#11761,#11762,#11763,#11764,#11765,
#11766,#11767,#11768,#11769,#11770,#11771,#11772,#11773,#11774,#11775,#11776,
#11777,#11778,#11779,#11780,#11781,#11782,#11783,#11784,#11785,#11786,#11787,
#11788,#11789,#11790,#11791,#11792,#11793,#11794,#11795,#11796,#11797,#11798,
#11799,#11800,#11801,#11802,#11803,#11804,#11805,#11806,#11807,#11808,#11809,
#11810,#11811,#11812,#11813,#11814,#11815,#11816,#11817,#11818,#11819,#11820,
#11821,#11822,#11823,#11824,#11825,#11826,#11827,#11828,#11829,#11830,#11831,
#11832,#11833,#11834,#11835,#11836,#11837,#11838,#11839,#11840,#11841,#11842),
 .UNSPECIFIED.,.F.,.F.,(4,3,3,3,3,3,3,3,3,3,3,3,3,3,3,3,3,3,3,3,3,3,3,3,
3,3,3,4),(0.,0.0185974621992716,0.0384224336108711,0.0557692835960208,0.0644714038145787,
0.0684505970799104,0.0885047587343187,0.108914678740463,0.125985317428364,
0.133848187707592,0.137284575106013,0.158359458782245,0.177197233492068,
0.197725010283636,0.205649646146363,0.209125337461315,0.230131020660481,
0.251623277314659,0.268075188611861,0.278317572045085,0.284044650132327,
0.306313638421511,0.322966021230938,0.32817264982967,0.333184030557865,
0.355705445009595,0.372923169659219,0.376940817211665),.UNSPECIFIED.);
#258=B_SPLINE_CURVE_WITH_KNOTS('',3,(#11843,#11844,#11845,#11846,#11847,
#11848,#11849,#11850,#11851,#11852,#11853,#11854,#11855,#11856,#11857,#11858,
#11859,#11860,#11861,#11862,#11863,#11864,#11865,#11866,#11867),
 .UNSPECIFIED.,.F.,.F.,(4,3,3,3,3,3,3,3,4),(-10.1295685708718,-9.97528534436599,
-8.97775680992939,-7.98022827549279,-6.98269974105619,-5.9851712066196,
-4.987642672183,-3.9901141377464,-3.84638326369226),.UNSPECIFIED.);
#259=B_SPLINE_CURVE_WITH_KNOTS('',3,(#12284,#12285,#12286,#12287,#12288,
#12289,#12290,#12291,#12292,#12293,#12294,#12295,#12296,#12297,#12298,#12299,
#12300,#12301,#12302,#12303,#12304,#12305),.UNSPECIFIED.,.F.,.F.,(4,3,3,
3,3,3,3,4),(7.59300756235152,7.9802282754928,8.9777568099294,9.97528534436599,
10.9728138788026,11.9703424132392,12.9678709476758,13.8761928695311),
 .UNSPECIFIED.);
#260=B_SPLINE_CURVE_WITH_KNOTS('',3,(#12306,#12307,#12308,#12309,#12310,
#12311,#12312,#12313,#12314,#12315,#12316,#12317,#12318,#12319,#12320,#12321,
#12322,#12323,#12324,#12325,#12326,#12327,#12328,#12329,#12330,#12331,#12332,
#12333,#12334,#12335,#12336,#12337,#12338,#12339,#12340,#12341,#12342,#12343,
#12344,#12345,#12346,#12347,#12348,#12349,#12350,#12351,#12352,#12353,#12354,
#12355,#12356,#12357,#12358,#12359,#12360,#12361,#12362,#12363,#12364,#12365,
#12366,#12367,#12368,#12369,#12370,#12371,#12372,#12373,#12374,#12375,#12376,
#12377,#12378,#12379,#12380,#12381,#12382,#12383,#12384,#12385,#12386,#12387,
#12388,#12389,#12390),.UNSPECIFIED.,.F.,.F.,(4,3,3,3,3,3,3,3,3,3,3,3,3,
3,3,3,3,3,3,3,3,3,3,3,3,3,3,3,4),(0.,0.0219660882001754,0.0445435574926492,
0.0636200527620001,0.072096934670327,0.0767543921860232,0.0810485334836077,
0.102995134794825,0.124771443916311,0.142867462849098,0.150422747843521,
0.153917793932026,0.157566639164433,0.178337409068225,0.197155519647456,
0.219426672701598,0.224328243169774,0.229401233280989,0.250066316947288,
0.270727133327362,0.285676274903019,0.296892293101634,0.3006231612417,0.320395528034006,
0.334302244254764,0.33876864872058,0.357793747762356,0.375324744080587,
0.378621596831435),.UNSPECIFIED.);
#261=B_SPLINE_CURVE_WITH_KNOTS('',3,(#12393,#12394,#12395,#12396,#12397,
#12398,#12399,#12400,#12401,#12402,#12403,#12404,#12405,#12406,#12407,#12408,
#12409,#12410,#12411,#12412,#12413,#12414,#12415,#12416,#12417,#12418,#12419,
#12420,#12421,#12422,#12423,#12424,#12425,#12426,#12427,#12428,#12429,#12430,
#12431,#12432,#12433,#12434,#12435,#12436,#12437,#12438,#12439,#12440,#12441,
#12442,#12443,#12444,#12445,#12446,#12447,#12448,#12449,#12450,#12451,#12452,
#12453,#12454,#12455,#12456,#12457,#12458,#12459,#12460,#12461,#12462,#12463,
#12464,#12465,#12466,#12467,#12468,#12469,#12470,#12471,#12472,#12473,#12474,
#12475,#12476,#12477,#12478,#12479,#12480),.UNSPECIFIED.,.F.,.F.,(4,3,3,
3,3,3,3,3,3,3,3,3,3,3,3,3,3,3,3,3,3,3,3,3,3,3,3,3,3,4),(-0.378621596831286,
-0.359797531939329,-0.347859674088644,-0.339722371887868,-0.335384191996609,
-0.315512528545638,-0.301178156546342,-0.297261836653107,-0.293227372722428,
-0.272825152816335,-0.252127491378394,-0.239305006671613,-0.228805773055512,
-0.224505205545998,-0.203200647370982,-0.200837552551268,-0.180350219633511,
-0.158310727079811,-0.154330126777592,-0.15080940414484,-0.129426105765746,
-0.107591922992953,-0.0856253011071385,-0.0802030000345852,-0.0759441337694857,
-0.0533965546995145,-0.030824386572716,-0.00876574406647046,-0.00403427920390719,
0.),.UNSPECIFIED.);
#262=B_SPLINE_CURVE_WITH_KNOTS('',3,(#12481,#12482,#12483,#12484,#12485,
#12486,#12487,#12488,#12489,#12490,#12491,#12492,#12493,#12494,#12495,#12496,
#12497,#12498,#12499,#12500,#12501,#12502,#12503,#12504,#12505,#12506,#12507,
#12508,#12509,#12510,#12511,#12512,#12513,#12514,#12515,#12516,#12517,#12518,
#12519,#12520,#12521,#12522,#12523,#12524,#12525,#12526,#12527,#12528,#12529,
#12530,#12531,#12532,#12533,#12534,#12535,#12536,#12537,#12538,#12539,#12540,
#12541,#12542,#12543,#12544,#12545,#12546,#12547,#12548,#12549,#12550,#12551,
#12552,#12553,#12554,#12555,#12556,#12557,#12558,#12559,#12560,#12561,#12562,
#12563,#12564,#12565),.UNSPECIFIED.,.F.,.F.,(4,3,3,3,3,3,3,3,3,3,3,3,3,
3,3,3,3,3,3,3,3,3,3,3,3,3,3,3,4),(-0.37694081721167,-0.354634311564495,
-0.332912880828966,-0.328064590370635,-0.305815990568489,-0.290196849957461,
-0.284261070057056,-0.278600435131014,-0.256917262572502,-0.235699695321403,
-0.214947468634417,-0.208197212481371,-0.20440205636235,-0.183825918074776,
-0.180862865680265,-0.159880209071646,-0.140305785711372,-0.136021299100323,
-0.132587889613715,-0.112128572210918,-0.091763979903476,-0.0718357249425283,
-0.0676215956084049,-0.0636601180723756,-0.0441022280989914,-0.0249162877192308,
-0.00635331060543922,-0.00328482218945702,0.),.UNSPECIFIED.);
#263=B_SPLINE_CURVE_WITH_KNOTS('',3,(#12567,#12568,#12569,#12570,#12571,
#12572,#12573,#12574,#12575,#12576,#12577),.UNSPECIFIED.,.F.,.F.,(4,1,1,
1,1,1,1,1,4),(15.7079632679489,15.851694142003,16.8492226764396,17.8467512108762,
18.8442797453128,19.8418082797494,20.839336814186,21.8368653486226,21.9911485751285),
 .UNSPECIFIED.);
#264=B_SPLINE_CURVE_WITH_KNOTS('',3,(#12578,#12579,#12580,#12581,#12582,
#12583,#12584,#12585,#12586,#12587),.UNSPECIFIED.,.F.,.F.,(4,1,1,1,1,1,
1,4),(15.7079632679489,16.3931980816501,17.3907266160867,18.3882551505233,
19.3857836849599,20.3833122193965,21.3808407538331,21.9911485751285),
 .UNSPECIFIED.);
#265=B_SPLINE_CURVE_WITH_KNOTS('',3,(#13004,#13005,#13006,#13007,#13008,
#13009,#13010,#13011,#13012,#13013,#13014,#13015,#13016,#13017,#13018,#13019,
#13020,#13021,#13022,#13023,#13024,#13025,#13026,#13027,#13028,#13029,#13030,
#13031,#13032,#13033,#13034,#13035,#13036,#13037,#13038,#13039,#13040,#13041,
#13042,#13043,#13044,#13045,#13046,#13047,#13048,#13049,#13050,#13051,#13052,
#13053,#13054,#13055,#13056,#13057,#13058,#13059,#13060,#13061,#13062,#13063,
#13064,#13065,#13066,#13067,#13068,#13069,#13070,#13071,#13072,#13073,#13074,
#13075,#13076,#13077,#13078,#13079,#13080,#13081,#13082,#13083,#13084,#13085),
 .UNSPECIFIED.,.F.,.F.,(4,3,3,3,3,3,3,3,3,3,3,3,3,3,3,3,3,3,3,3,3,3,3,3,
3,3,3,4),(0.,0.018597446670301,0.0384224200230219,0.0557692717066527,0.0644713832373243,
0.0684505917335086,0.0885047423038066,0.108914657526654,0.125985301518008,
0.133848162658074,0.137284562057273,0.158359447175397,0.177197233492068,
0.197725018062199,0.205649650255122,0.209125340384878,0.230131032726425,
0.2516232941941,0.268075184696176,0.278317563017783,0.284044652367558,0.306313641227486,
0.32296602333542,0.328172654498713,0.333184032913153,0.35570544729198,0.372923169659219,
0.376940817211665),.UNSPECIFIED.);
#266=B_SPLINE_CURVE_WITH_KNOTS('',3,(#13086,#13087,#13088,#13089,#13090,
#13091,#13092,#13093,#13094,#13095,#13096,#13097,#13098,#13099,#13100,#13101,
#13102,#13103,#13104,#13105,#13106,#13107,#13108,#13109,#13110),
 .UNSPECIFIED.,.F.,.F.,(4,3,3,3,3,3,3,3,4),(-10.1295685708718,-9.97528534436599,
-8.97775680992939,-7.98022827549279,-6.98269974105619,-5.9851712066196,
-4.987642672183,-3.9901141377464,-3.84638326369226),.UNSPECIFIED.);
#267=B_SPLINE_CURVE_WITH_KNOTS('',3,(#13527,#13528,#13529,#13530,#13531,
#13532,#13533,#13534,#13535,#13536,#13537,#13538,#13539,#13540,#13541,#13542,
#13543,#13544,#13545,#13546,#13547,#13548),.UNSPECIFIED.,.F.,.F.,(4,3,3,
3,3,3,3,4),(7.59300756235152,7.9802282754928,8.9777568099294,9.97528534436599,
10.9728138788026,11.9703424132392,12.9678709476758,13.8761928695311),
 .UNSPECIFIED.);
#268=B_SPLINE_CURVE_WITH_KNOTS('',3,(#13549,#13550,#13551,#13552,#13553,
#13554,#13555,#13556,#13557,#13558,#13559,#13560,#13561,#13562,#13563,#13564,
#13565,#13566,#13567,#13568,#13569,#13570,#13571,#13572,#13573,#13574,#13575,
#13576,#13577,#13578,#13579,#13580,#13581,#13582,#13583,#13584,#13585,#13586,
#13587,#13588,#13589,#13590,#13591,#13592,#13593,#13594,#13595,#13596,#13597,
#13598,#13599,#13600,#13601,#13602,#13603,#13604,#13605,#13606,#13607,#13608,
#13609,#13610,#13611,#13612,#13613,#13614,#13615,#13616,#13617,#13618,#13619,
#13620,#13621,#13622,#13623,#13624,#13625,#13626,#13627,#13628,#13629,#13630,
#13631,#13632,#13633),.UNSPECIFIED.,.F.,.F.,(4,3,3,3,3,3,3,3,3,3,3,3,3,
3,3,3,3,3,3,3,3,3,3,3,3,3,3,3,4),(0.,0.0219660926710697,0.0445435623967901,
0.0636200570531234,0.0720969359510079,0.0767543948971924,0.0810485342081409,
0.102995135433386,0.124771443207436,0.142867462317441,0.150422748080518,
0.153917795373617,0.157566639616675,0.178337408178314,0.197155519647456,
0.219426672701598,0.224328242817097,0.22940123326696,0.250066317110923,
0.270727133335975,0.285676270869573,0.296892286105422,0.30062315925361,
0.320395524461199,0.334302238332921,0.338768643269476,0.357793739793908,
0.375324744080587,0.378621596831435),.UNSPECIFIED.);
#418=SHAPE_REPRESENTATION_RELATIONSHIP('SRR','None',#19936,#437);
#437=ADVANCED_BREP_SHAPE_REPRESENTATION('',(#475),#19845);
#456=STYLED_ITEM('',(#20040),#475);
#475=MANIFOLD_SOLID_BREP('Body1',#6425);
#561=LINE('',#8910,#1026);
#562=LINE('',#8939,#1027);
#563=LINE('',#8966,#1028);
#564=LINE('',#9017,#1029);
#565=LINE('',#9065,#1030);
#566=LINE('',#9116,#1031);
#567=LINE('',#9167,#1032);
#568=LINE('',#9215,#1033);
#569=LINE('',#9263,#1034);
#570=LINE('',#9314,#1035);
#571=LINE('',#9362,#1036);
#572=LINE('',#9410,#1037);
#573=LINE('',#9461,#1038);
#574=LINE('',#9512,#1039);
#575=LINE('',#9560,#1040);
#576=LINE('',#9611,#1041);
#577=LINE('',#9650,#1042);
#578=LINE('',#9670,#1043);
#579=LINE('',#9694,#1044);
#580=LINE('',#9719,#1045);
#581=LINE('',#9744,#1046);
#582=LINE('',#9768,#1047);
#583=LINE('',#9793,#1048);
#584=LINE('',#9817,#1049);
#585=LINE('',#9842,#1050);
#586=LINE('',#9867,#1051);
#587=LINE('',#9891,#1052);
#588=LINE('',#9916,#1053);
#589=LINE('',#9940,#1054);
#590=LINE('',#9965,#1055);
#591=LINE('',#9990,#1056);
#592=LINE('',#10014,#1057);
#593=LINE('',#10031,#1058);
#594=LINE('',#10060,#1059);
#595=LINE('',#10087,#1060);
#596=LINE('',#10138,#1061);
#597=LINE('',#10186,#1062);
#598=LINE('',#10237,#1063);
#599=LINE('',#10288,#1064);
#600=LINE('',#10336,#1065);
#601=LINE('',#10384,#1066);
#602=LINE('',#10435,#1067);
#603=LINE('',#10483,#1068);
#604=LINE('',#10531,#1069);
#605=LINE('',#10582,#1070);
#606=LINE('',#10633,#1071);
#607=LINE('',#10681,#1072);
#608=LINE('',#10732,#1073);
#609=LINE('',#10771,#1074);
#610=LINE('',#10791,#1075);
#611=LINE('',#10815,#1076);
#612=LINE('',#10840,#1077);
#613=LINE('',#10865,#1078);
#614=LINE('',#10889,#1079);
#615=LINE('',#10914,#1080);
#616=LINE('',#10938,#1081);
#617=LINE('',#10963,#1082);
#618=LINE('',#10988,#1083);
#619=LINE('',#11012,#1084);
#620=LINE('',#11037,#1085);
#621=LINE('',#11061,#1086);
#622=LINE('',#11086,#1087);
#623=LINE('',#11111,#1088);
#624=LINE('',#11135,#1089);
#625=LINE('',#13641,#1090);
#626=LINE('',#13647,#1091);
#627=LINE('',#13653,#1092);
#628=LINE('',#13658,#1093);
#629=LINE('',#13660,#1094);
#630=LINE('',#13662,#1095);
#631=LINE('',#13663,#1096);
#632=LINE('',#13667,#1097);
#633=LINE('',#13669,#1098);
#634=LINE('',#13671,#1099);
#635=LINE('',#13672,#1100);
#636=LINE('',#13674,#1101);
#637=LINE('',#13675,#1102);
#638=LINE('',#13678,#1103);
#639=LINE('',#13680,#1104);
#640=LINE('',#13681,#1105);
#641=LINE('',#13684,#1106);
#642=LINE('',#13686,#1107);
#643=LINE('',#13687,#1108);
#644=LINE('',#13691,#1109);
#645=LINE('',#13693,#1110);
#646=LINE('',#13695,#1111);
#647=LINE('',#13696,#1112);
#648=LINE('',#13699,#1113);
#649=LINE('',#13701,#1114);
#650=LINE('',#13702,#1115);
#651=LINE('',#13705,#1116);
#652=LINE('',#13707,#1117);
#653=LINE('',#13708,#1118);
#654=LINE('',#13710,#1119);
#655=LINE('',#13713,#1120);
#656=LINE('',#13715,#1121);
#657=LINE('',#13717,#1122);
#658=LINE('',#13719,#1123);
#659=LINE('',#13721,#1124);
#660=LINE('',#13723,#1125);
#661=LINE('',#13725,#1126);
#662=LINE('',#13727,#1127);
#663=LINE('',#13728,#1128);
#664=LINE('',#13731,#1129);
#665=LINE('',#13733,#1130);
#666=LINE('',#13735,#1131);
#667=LINE('',#13736,#1132);
#668=LINE('',#13739,#1133);
#669=LINE('',#13741,#1134);
#670=LINE('',#13743,#1135);
#671=LINE('',#13744,#1136);
#672=LINE('',#13746,#1137);
#673=LINE('',#13747,#1138);
#674=LINE('',#13749,#1139);
#675=LINE('',#13751,#1140);
#676=LINE('',#13754,#1141);
#677=LINE('',#13756,#1142);
#678=LINE('',#13758,#1143);
#679=LINE('',#13760,#1144);
#680=LINE('',#13762,#1145);
#681=LINE('',#13764,#1146);
#682=LINE('',#13765,#1147);
#683=LINE('',#13769,#1148);
#684=LINE('',#13770,#1149);
#685=LINE('',#13771,#1150);
#686=LINE('',#13774,#1151);
#687=LINE('',#13775,#1152);
#688=LINE('',#13778,#1153);
#689=LINE('',#13779,#1154);
#690=LINE('',#13781,#1155);
#691=LINE('',#13785,#1156);
#692=LINE('',#13786,#1157);
#693=LINE('',#13787,#1158);
#694=LINE('',#13790,#1159);
#695=LINE('',#13791,#1160);
#696=LINE('',#13794,#1161);
#697=LINE('',#13795,#1162);
#698=LINE('',#13797,#1163);
#699=LINE('',#13801,#1164);
#700=LINE('',#13802,#1165);
#701=LINE('',#13804,#1166);
#702=LINE('',#13806,#1167);
#703=LINE('',#13808,#1168);
#704=LINE('',#13810,#1169);
#705=LINE('',#13811,#1170);
#706=LINE('',#13814,#1171);
#707=LINE('',#13815,#1172);
#708=LINE('',#13818,#1173);
#709=LINE('',#13820,#1174);
#710=LINE('',#13821,#1175);
#711=LINE('',#13824,#1176);
#712=LINE('',#13825,#1177);
#713=LINE('',#13828,#1178);
#714=LINE('',#13830,#1179);
#715=LINE('',#13831,#1180);
#716=LINE('',#13832,#1181);
#717=LINE('',#13834,#1182);
#718=LINE('',#13838,#1183);
#719=LINE('',#13839,#1184);
#720=LINE('',#13842,#1185);
#721=LINE('',#13843,#1186);
#722=LINE('',#13845,#1187);
#723=LINE('',#13846,#1188);
#1026=VECTOR('',#7363,2.);
#1027=VECTOR('',#7366,2.);
#1028=VECTOR('',#7371,2.);
#1029=VECTOR('',#7374,2.);
#1030=VECTOR('',#7377,2.);
#1031=VECTOR('',#7380,2.);
#1032=VECTOR('',#7383,2.);
#1033=VECTOR('',#7386,2.);
#1034=VECTOR('',#7389,2.);
#1035=VECTOR('',#7392,2.);
#1036=VECTOR('',#7395,2.);
#1037=VECTOR('',#7398,2.);
#1038=VECTOR('',#7401,2.);
#1039=VECTOR('',#7404,2.);
#1040=VECTOR('',#7407,2.);
#1041=VECTOR('',#7410,2.);
#1042=VECTOR('',#7415,2.05475);
#1043=VECTOR('',#7420,2.05475);
#1044=VECTOR('',#7423,2.05475);
#1045=VECTOR('',#7426,2.05475);
#1046=VECTOR('',#7429,2.05475);
#1047=VECTOR('',#7432,2.05475);
#1048=VECTOR('',#7435,2.05475);
#1049=VECTOR('',#7438,2.05475);
#1050=VECTOR('',#7441,2.05475);
#1051=VECTOR('',#7444,2.05475);
#1052=VECTOR('',#7447,2.05475);
#1053=VECTOR('',#7450,2.05475);
#1054=VECTOR('',#7453,2.05475);
#1055=VECTOR('',#7456,2.05475);
#1056=VECTOR('',#7459,2.05475);
#1057=VECTOR('',#7462,2.05475);
#1058=VECTOR('',#7467,2.);
#1059=VECTOR('',#7470,2.);
#1060=VECTOR('',#7475,2.);
#1061=VECTOR('',#7478,2.);
#1062=VECTOR('',#7481,2.);
#1063=VECTOR('',#7484,2.);
#1064=VECTOR('',#7487,2.);
#1065=VECTOR('',#7490,2.);
#1066=VECTOR('',#7493,2.);
#1067=VECTOR('',#7496,2.);
#1068=VECTOR('',#7499,2.);
#1069=VECTOR('',#7502,2.);
#1070=VECTOR('',#7505,2.);
#1071=VECTOR('',#7508,2.);
#1072=VECTOR('',#7511,2.);
#1073=VECTOR('',#7514,2.);
#1074=VECTOR('',#7519,2.05475);
#1075=VECTOR('',#7524,2.05475);
#1076=VECTOR('',#7527,2.05475);
#1077=VECTOR('',#7530,2.05475);
#1078=VECTOR('',#7533,2.05475);
#1079=VECTOR('',#7536,2.05475);
#1080=VECTOR('',#7539,2.05475);
#1081=VECTOR('',#7542,2.05475);
#1082=VECTOR('',#7545,2.05475);
#1083=VECTOR('',#7548,2.05475);
#1084=VECTOR('',#7551,2.05475);
#1085=VECTOR('',#7554,2.05475);
#1086=VECTOR('',#7557,2.05475);
#1087=VECTOR('',#7560,2.05475);
#1088=VECTOR('',#7563,2.05475);
#1089=VECTOR('',#7566,2.05475);
#1090=VECTOR('',#7589,2.);
#1091=VECTOR('',#7596,4.);
#1092=VECTOR('',#7603,4.);
#1093=VECTOR('',#7608,10.);
#1094=VECTOR('',#7609,10.);
#1095=VECTOR('',#7610,10.);
#1096=VECTOR('',#7611,10.);
#1097=VECTOR('',#7614,10.);
#1098=VECTOR('',#7615,10.);
#1099=VECTOR('',#7616,10.);
#1100=VECTOR('',#7617,10.);
#1101=VECTOR('',#7620,10.);
#1102=VECTOR('',#7621,10.);
#1103=VECTOR('',#7624,10.);
#1104=VECTOR('',#7625,10.);
#1105=VECTOR('',#7626,10.);
#1106=VECTOR('',#7629,10.);
#1107=VECTOR('',#7630,10.);
#1108=VECTOR('',#7631,10.);
#1109=VECTOR('',#7634,10.);
#1110=VECTOR('',#7635,10.);
#1111=VECTOR('',#7636,10.);
#1112=VECTOR('',#7637,10.);
#1113=VECTOR('',#7640,10.);
#1114=VECTOR('',#7641,10.);
#1115=VECTOR('',#7642,10.);
#1116=VECTOR('',#7645,10.);
#1117=VECTOR('',#7646,10.);
#1118=VECTOR('',#7647,10.);
#1119=VECTOR('',#7650,10.);
#1120=VECTOR('',#7653,10.);
#1121=VECTOR('',#7654,10.);
#1122=VECTOR('',#7655,10.);
#1123=VECTOR('',#7656,10.);
#1124=VECTOR('',#7657,10.);
#1125=VECTOR('',#7658,10.);
#1126=VECTOR('',#7659,10.);
#1127=VECTOR('',#7660,10.);
#1128=VECTOR('',#7661,10.);
#1129=VECTOR('',#7662,10.);
#1130=VECTOR('',#7663,10.);
#1131=VECTOR('',#7664,10.);
#1132=VECTOR('',#7665,10.);
#1133=VECTOR('',#7666,10.);
#1134=VECTOR('',#7667,10.);
#1135=VECTOR('',#7668,10.);
#1136=VECTOR('',#7669,10.);
#1137=VECTOR('',#7672,10.);
#1138=VECTOR('',#7673,10.);
#1139=VECTOR('',#7676,10.);
#1140=VECTOR('',#7679,10.);
#1141=VECTOR('',#7682,10.);
#1142=VECTOR('',#7683,10.);
#1143=VECTOR('',#7684,10.);
#1144=VECTOR('',#7685,10.);
#1145=VECTOR('',#7686,10.);
#1146=VECTOR('',#7687,10.);
#1147=VECTOR('',#7688,10.);
#1148=VECTOR('',#7691,10.);
#1149=VECTOR('',#7692,10.);
#1150=VECTOR('',#7693,10.);
#1151=VECTOR('',#7696,10.);
#1152=VECTOR('',#7697,10.);
#1153=VECTOR('',#7700,10.);
#1154=VECTOR('',#7701,10.);
#1155=VECTOR('',#7704,10.);
#1156=VECTOR('',#7707,10.);
#1157=VECTOR('',#7708,10.);
#1158=VECTOR('',#7709,10.);
#1159=VECTOR('',#7712,10.);
#1160=VECTOR('',#7713,10.);
#1161=VECTOR('',#7716,10.);
#1162=VECTOR('',#7717,10.);
#1163=VECTOR('',#7720,10.);
#1164=VECTOR('',#7723,10.);
#1165=VECTOR('',#7724,10.);
#1166=VECTOR('',#7725,10.);
#1167=VECTOR('',#7726,10.);
#1168=VECTOR('',#7727,10.);
#1169=VECTOR('',#7728,10.);
#1170=VECTOR('',#7729,10.);
#1171=VECTOR('',#7732,10.);
#1172=VECTOR('',#7733,10.);
#1173=VECTOR('',#7736,10.);
#1174=VECTOR('',#7737,10.);
#1175=VECTOR('',#7738,10.);
#1176=VECTOR('',#7741,10.);
#1177=VECTOR('',#7742,10.);
#1178=VECTOR('',#7745,10.);
#1179=VECTOR('',#7746,10.);
#1180=VECTOR('',#7747,10.);
#1181=VECTOR('',#7748,10.);
#1182=VECTOR('',#7751,10.);
#1183=VECTOR('',#7756,10.);
#1184=VECTOR('',#7757,10.);
#1185=VECTOR('',#7760,10.);
#1186=VECTOR('',#7761,10.);
#1187=VECTOR('',#7764,10.);
#1188=VECTOR('',#7765,10.);
#1431=CYLINDRICAL_SURFACE('',#6704,1.666);
#1432=CYLINDRICAL_SURFACE('',#6707,1.666);
#1433=CYLINDRICAL_SURFACE('',#6708,1.666);
#1434=CYLINDRICAL_SURFACE('',#6709,1.666);
#1435=CYLINDRICAL_SURFACE('',#6710,1.666);
#1436=CYLINDRICAL_SURFACE('',#6711,1.666);
#1437=CYLINDRICAL_SURFACE('',#6712,1.666);
#1438=CYLINDRICAL_SURFACE('',#6713,1.666);
#1439=CYLINDRICAL_SURFACE('',#6714,1.666);
#1440=CYLINDRICAL_SURFACE('',#6715,1.666);
#1441=CYLINDRICAL_SURFACE('',#6716,1.666);
#1442=CYLINDRICAL_SURFACE('',#6717,1.666);
#1443=CYLINDRICAL_SURFACE('',#6718,1.666);
#1444=CYLINDRICAL_SURFACE('',#6719,1.666);
#1445=CYLINDRICAL_SURFACE('',#6720,1.666);
#1446=CYLINDRICAL_SURFACE('',#6722,2.05475);
#1447=CYLINDRICAL_SURFACE('',#6724,2.05475);
#1448=CYLINDRICAL_SURFACE('',#6725,2.05475);
#1449=CYLINDRICAL_SURFACE('',#6726,2.05475);
#1450=CYLINDRICAL_SURFACE('',#6727,2.05475);
#1451=CYLINDRICAL_SURFACE('',#6728,2.05475);
#1452=CYLINDRICAL_SURFACE('',#6729,2.05475);
#1453=CYLINDRICAL_SURFACE('',#6730,2.05475);
#1454=CYLINDRICAL_SURFACE('',#6731,2.05475);
#1455=CYLINDRICAL_SURFACE('',#6732,2.05475);
#1456=CYLINDRICAL_SURFACE('',#6733,2.05475);
#1457=CYLINDRICAL_SURFACE('',#6734,2.05475);
#1458=CYLINDRICAL_SURFACE('',#6735,2.05475);
#1459=CYLINDRICAL_SURFACE('',#6736,2.05475);
#1460=CYLINDRICAL_SURFACE('',#6737,2.05475);
#1461=CYLINDRICAL_SURFACE('',#6738,2.05475);
#1462=CYLINDRICAL_SURFACE('',#6740,1.666);
#1463=CYLINDRICAL_SURFACE('',#6743,1.666);
#1464=CYLINDRICAL_SURFACE('',#6744,1.666);
#1465=CYLINDRICAL_SURFACE('',#6745,1.666);
#1466=CYLINDRICAL_SURFACE('',#6746,1.666);
#1467=CYLINDRICAL_SURFACE('',#6747,1.666);
#1468=CYLINDRICAL_SURFACE('',#6748,1.666);
#1469=CYLINDRICAL_SURFACE('',#6749,1.666);
#1470=CYLINDRICAL_SURFACE('',#6750,1.666);
#1471=CYLINDRICAL_SURFACE('',#6751,1.666);
#1472=CYLINDRICAL_SURFACE('',#6752,1.666);
#1473=CYLINDRICAL_SURFACE('',#6753,1.666);
#1474=CYLINDRICAL_SURFACE('',#6754,1.666);
#1475=CYLINDRICAL_SURFACE('',#6755,1.666);
#1476=CYLINDRICAL_SURFACE('',#6756,1.666);
#1477=CYLINDRICAL_SURFACE('',#6758,2.05475);
#1478=CYLINDRICAL_SURFACE('',#6760,2.05475);
#1479=CYLINDRICAL_SURFACE('',#6761,2.05475);
#1480=CYLINDRICAL_SURFACE('',#6762,2.05475);
#1481=CYLINDRICAL_SURFACE('',#6763,2.05475);
#1482=CYLINDRICAL_SURFACE('',#6764,2.05475);
#1483=CYLINDRICAL_SURFACE('',#6765,2.05475);
#1484=CYLINDRICAL_SURFACE('',#6766,2.05475);
#1485=CYLINDRICAL_SURFACE('',#6767,2.05475);
#1486=CYLINDRICAL_SURFACE('',#6768,2.05475);
#1487=CYLINDRICAL_SURFACE('',#6769,2.05475);
#1488=CYLINDRICAL_SURFACE('',#6770,2.05475);
#1489=CYLINDRICAL_SURFACE('',#6771,2.05475);
#1490=CYLINDRICAL_SURFACE('',#6772,2.05475);
#1491=CYLINDRICAL_SURFACE('',#6773,2.05475);
#1492=CYLINDRICAL_SURFACE('',#6774,2.05475);
#1493=CYLINDRICAL_SURFACE('',#6777,2.05475);
#1494=CYLINDRICAL_SURFACE('',#6778,1.666);
#1495=CYLINDRICAL_SURFACE('',#6780,2.05475);
#1496=CYLINDRICAL_SURFACE('',#6781,1.666);
#1497=CYLINDRICAL_SURFACE('',#6784,2.);
#1498=CYLINDRICAL_SURFACE('',#6787,4.);
#1499=CYLINDRICAL_SURFACE('',#6790,4.);
#1634=FACE_BOUND('',#2178,.T.);
#1635=FACE_BOUND('',#2183,.T.);
#1636=FACE_BOUND('',#2184,.T.);
#1637=FACE_BOUND('',#2186,.T.);
#1638=FACE_BOUND('',#2187,.T.);
#1639=FACE_BOUND('',#2191,.T.);
#1640=FACE_BOUND('',#2192,.T.);
#1641=FACE_BOUND('',#2208,.T.);
#1642=FACE_BOUND('',#2209,.T.);
#1643=FACE_BOUND('',#2211,.T.);
#1644=FACE_BOUND('',#2213,.T.);
#1645=FACE_BOUND('',#2215,.T.);
#1719=FACE_OUTER_BOUND('',#2095,.T.);
#1720=FACE_OUTER_BOUND('',#2096,.T.);
#1721=FACE_OUTER_BOUND('',#2097,.T.);
#1722=FACE_OUTER_BOUND('',#2098,.T.);
#1723=FACE_OUTER_BOUND('',#2099,.T.);
#1724=FACE_OUTER_BOUND('',#2100,.T.);
#1725=FACE_OUTER_BOUND('',#2101,.T.);
#1726=FACE_OUTER_BOUND('',#2102,.T.);
#1727=FACE_OUTER_BOUND('',#2103,.T.);
#1728=FACE_OUTER_BOUND('',#2104,.T.);
#1729=FACE_OUTER_BOUND('',#2105,.T.);
#1730=FACE_OUTER_BOUND('',#2106,.T.);
#1731=FACE_OUTER_BOUND('',#2107,.T.);
#1732=FACE_OUTER_BOUND('',#2108,.T.);
#1733=FACE_OUTER_BOUND('',#2109,.T.);
#1734=FACE_OUTER_BOUND('',#2110,.T.);
#1735=FACE_OUTER_BOUND('',#2111,.T.);
#1736=FACE_OUTER_BOUND('',#2112,.T.);
#1737=FACE_OUTER_BOUND('',#2113,.T.);
#1738=FACE_OUTER_BOUND('',#2114,.T.);
#1739=FACE_OUTER_BOUND('',#2115,.T.);
#1740=FACE_OUTER_BOUND('',#2116,.T.);
#1741=FACE_OUTER_BOUND('',#2117,.T.);
#1742=FACE_OUTER_BOUND('',#2118,.T.);
#1743=FACE_OUTER_BOUND('',#2119,.T.);
#1744=FACE_OUTER_BOUND('',#2120,.T.);
#1745=FACE_OUTER_BOUND('',#2121,.T.);
#1746=FACE_OUTER_BOUND('',#2122,.T.);
#1747=FACE_OUTER_BOUND('',#2123,.T.);
#1748=FACE_OUTER_BOUND('',#2124,.T.);
#1749=FACE_OUTER_BOUND('',#2125,.T.);
#1750=FACE_OUTER_BOUND('',#2126,.T.);
#1751=FACE_OUTER_BOUND('',#2127,.T.);
#1752=FACE_OUTER_BOUND('',#2128,.T.);
#1753=FACE_OUTER_BOUND('',#2129,.T.);
#1754=FACE_OUTER_BOUND('',#2130,.T.);
#1755=FACE_OUTER_BOUND('',#2131,.T.);
#1756=FACE_OUTER_BOUND('',#2132,.T.);
#1757=FACE_OUTER_BOUND('',#2133,.T.);
#1758=FACE_OUTER_BOUND('',#2134,.T.);
#1759=FACE_OUTER_BOUND('',#2135,.T.);
#1760=FACE_OUTER_BOUND('',#2136,.T.);
#1761=FACE_OUTER_BOUND('',#2137,.T.);
#1762=FACE_OUTER_BOUND('',#2138,.T.);
#1763=FACE_OUTER_BOUND('',#2139,.T.);
#1764=FACE_OUTER_BOUND('',#2140,.T.);
#1765=FACE_OUTER_BOUND('',#2141,.T.);
#1766=FACE_OUTER_BOUND('',#2142,.T.);
#1767=FACE_OUTER_BOUND('',#2143,.T.);
#1768=FACE_OUTER_BOUND('',#2144,.T.);
#1769=FACE_OUTER_BOUND('',#2145,.T.);
#1770=FACE_OUTER_BOUND('',#2146,.T.);
#1771=FACE_OUTER_BOUND('',#2147,.T.);
#1772=FACE_OUTER_BOUND('',#2148,.T.);
#1773=FACE_OUTER_BOUND('',#2149,.T.);
#1774=FACE_OUTER_BOUND('',#2150,.T.);
#1775=FACE_OUTER_BOUND('',#2151,.T.);
#1776=FACE_OUTER_BOUND('',#2152,.T.);
#1777=FACE_OUTER_BOUND('',#2153,.T.);
#1778=FACE_OUTER_BOUND('',#2154,.T.);
#1779=FACE_OUTER_BOUND('',#2155,.T.);
#1780=FACE_OUTER_BOUND('',#2156,.T.);
#1781=FACE_OUTER_BOUND('',#2157,.T.);
#1782=FACE_OUTER_BOUND('',#2158,.T.);
#1783=FACE_OUTER_BOUND('',#2159,.T.);
#1784=FACE_OUTER_BOUND('',#2160,.T.);
#1785=FACE_OUTER_BOUND('',#2161,.T.);
#1786=FACE_OUTER_BOUND('',#2162,.T.);
#1787=FACE_OUTER_BOUND('',#2163,.T.);
#1788=FACE_OUTER_BOUND('',#2164,.T.);
#1789=FACE_OUTER_BOUND('',#2165,.T.);
#1790=FACE_OUTER_BOUND('',#2166,.T.);
#1791=FACE_OUTER_BOUND('',#2167,.T.);
#1792=FACE_OUTER_BOUND('',#2168,.T.);
#1793=FACE_OUTER_BOUND('',#2169,.T.);
#1794=FACE_OUTER_BOUND('',#2170,.T.);
#1795=FACE_OUTER_BOUND('',#2171,.T.);
#1796=FACE_OUTER_BOUND('',#2172,.T.);
#1797=FACE_OUTER_BOUND('',#2173,.T.);
#1798=FACE_OUTER_BOUND('',#2174,.T.);
#1799=FACE_OUTER_BOUND('',#2175,.T.);
#1800=FACE_OUTER_BOUND('',#2176,.T.);
#1801=FACE_OUTER_BOUND('',#2177,.T.);
#1802=FACE_OUTER_BOUND('',#2179,.T.);
#1803=FACE_OUTER_BOUND('',#2180,.T.);
#1804=FACE_OUTER_BOUND('',#2181,.T.);
#1805=FACE_OUTER_BOUND('',#2182,.T.);
#1806=FACE_OUTER_BOUND('',#2185,.T.);
#1807=FACE_OUTER_BOUND('',#2188,.T.);
#1808=FACE_OUTER_BOUND('',#2189,.T.);
#1809=FACE_OUTER_BOUND('',#2190,.T.);
#1810=FACE_OUTER_BOUND('',#2193,.T.);
#1811=FACE_OUTER_BOUND('',#2194,.T.);
#1812=FACE_OUTER_BOUND('',#2195,.T.);
#1813=FACE_OUTER_BOUND('',#2196,.T.);
#1814=FACE_OUTER_BOUND('',#2197,.T.);
#1815=FACE_OUTER_BOUND('',#2198,.T.);
#1816=FACE_OUTER_BOUND('',#2199,.T.);
#1817=FACE_OUTER_BOUND('',#2200,.T.);
#1818=FACE_OUTER_BOUND('',#2201,.T.);
#1819=FACE_OUTER_BOUND('',#2202,.T.);
#1820=FACE_OUTER_BOUND('',#2203,.T.);
#1821=FACE_OUTER_BOUND('',#2204,.T.);
#1822=FACE_OUTER_BOUND('',#2205,.T.);
#1823=FACE_OUTER_BOUND('',#2206,.T.);
#1824=FACE_OUTER_BOUND('',#2207,.T.);
#1825=FACE_OUTER_BOUND('',#2210,.T.);
#1826=FACE_OUTER_BOUND('',#2212,.T.);
#1827=FACE_OUTER_BOUND('',#2214,.T.);
#1828=FACE_OUTER_BOUND('',#2216,.T.);
#1829=FACE_OUTER_BOUND('',#2217,.T.);
#2095=EDGE_LOOP('',(#4283,#4284,#4285,#4286,#4287,#4288,#4289,#4290));
#2096=EDGE_LOOP('',(#4291,#4292,#4293,#4294));
#2097=EDGE_LOOP('',(#4295,#4296,#4297,#4298));
#2098=EDGE_LOOP('',(#4299,#4300,#4301,#4302));
#2099=EDGE_LOOP('',(#4303,#4304,#4305,#4306));
#2100=EDGE_LOOP('',(#4307,#4308,#4309,#4310));
#2101=EDGE_LOOP('',(#4311,#4312,#4313,#4314));
#2102=EDGE_LOOP('',(#4315,#4316,#4317,#4318));
#2103=EDGE_LOOP('',(#4319,#4320,#4321,#4322));
#2104=EDGE_LOOP('',(#4323,#4324,#4325,#4326));
#2105=EDGE_LOOP('',(#4327,#4328,#4329,#4330));
#2106=EDGE_LOOP('',(#4331,#4332,#4333,#4334));
#2107=EDGE_LOOP('',(#4335,#4336,#4337,#4338));
#2108=EDGE_LOOP('',(#4339,#4340,#4341,#4342));
#2109=EDGE_LOOP('',(#4343,#4344,#4345,#4346));
#2110=EDGE_LOOP('',(#4347,#4348,#4349,#4350));
#2111=EDGE_LOOP('',(#4351,#4352,#4353,#4354));
#2112=EDGE_LOOP('',(#4355,#4356,#4357,#4358));
#2113=EDGE_LOOP('',(#4359,#4360,#4361,#4362));
#2114=EDGE_LOOP('',(#4363,#4364,#4365,#4366));
#2115=EDGE_LOOP('',(#4367,#4368,#4369,#4370));
#2116=EDGE_LOOP('',(#4371,#4372,#4373,#4374));
#2117=EDGE_LOOP('',(#4375,#4376,#4377,#4378));
#2118=EDGE_LOOP('',(#4379,#4380,#4381,#4382));
#2119=EDGE_LOOP('',(#4383,#4384,#4385,#4386));
#2120=EDGE_LOOP('',(#4387,#4388,#4389,#4390));
#2121=EDGE_LOOP('',(#4391,#4392,#4393,#4394));
#2122=EDGE_LOOP('',(#4395,#4396,#4397,#4398));
#2123=EDGE_LOOP('',(#4399,#4400,#4401,#4402));
#2124=EDGE_LOOP('',(#4403,#4404,#4405,#4406));
#2125=EDGE_LOOP('',(#4407,#4408,#4409,#4410));
#2126=EDGE_LOOP('',(#4411,#4412,#4413,#4414,#4415,#4416,#4417,#4418));
#2127=EDGE_LOOP('',(#4419,#4420,#4421,#4422));
#2128=EDGE_LOOP('',(#4423,#4424,#4425,#4426));
#2129=EDGE_LOOP('',(#4427,#4428,#4429,#4430));
#2130=EDGE_LOOP('',(#4431,#4432,#4433,#4434));
#2131=EDGE_LOOP('',(#4435,#4436,#4437,#4438));
#2132=EDGE_LOOP('',(#4439,#4440,#4441,#4442));
#2133=EDGE_LOOP('',(#4443,#4444,#4445,#4446));
#2134=EDGE_LOOP('',(#4447,#4448,#4449,#4450));
#2135=EDGE_LOOP('',(#4451,#4452,#4453,#4454));
#2136=EDGE_LOOP('',(#4455,#4456,#4457,#4458));
#2137=EDGE_LOOP('',(#4459,#4460,#4461,#4462));
#2138=EDGE_LOOP('',(#4463,#4464,#4465,#4466));
#2139=EDGE_LOOP('',(#4467,#4468,#4469,#4470));
#2140=EDGE_LOOP('',(#4471,#4472,#4473,#4474));
#2141=EDGE_LOOP('',(#4475,#4476,#4477,#4478));
#2142=EDGE_LOOP('',(#4479,#4480,#4481,#4482));
#2143=EDGE_LOOP('',(#4483,#4484,#4485,#4486));
#2144=EDGE_LOOP('',(#4487,#4488,#4489,#4490));
#2145=EDGE_LOOP('',(#4491,#4492,#4493,#4494));
#2146=EDGE_LOOP('',(#4495,#4496,#4497,#4498));
#2147=EDGE_LOOP('',(#4499,#4500,#4501,#4502));
#2148=EDGE_LOOP('',(#4503,#4504,#4505,#4506));
#2149=EDGE_LOOP('',(#4507,#4508,#4509,#4510));
#2150=EDGE_LOOP('',(#4511,#4512,#4513,#4514));
#2151=EDGE_LOOP('',(#4515,#4516,#4517,#4518));
#2152=EDGE_LOOP('',(#4519,#4520,#4521,#4522));
#2153=EDGE_LOOP('',(#4523,#4524,#4525,#4526));
#2154=EDGE_LOOP('',(#4527,#4528,#4529,#4530));
#2155=EDGE_LOOP('',(#4531,#4532,#4533,#4534));
#2156=EDGE_LOOP('',(#4535,#4536,#4537,#4538));
#2157=EDGE_LOOP('',(#4539,#4540,#4541,#4542));
#2158=EDGE_LOOP('',(#4543,#4544,#4545,#4546));
#2159=EDGE_LOOP('',(#4547,#4548,#4549,#4550,#4551,#4552,#4553,#4554,#4555,
#4556,#4557,#4558,#4559,#4560,#4561,#4562,#4563,#4564,#4565,#4566,#4567,
#4568,#4569,#4570,#4571,#4572,#4573,#4574,#4575,#4576,#4577,#4578,#4579,
#4580,#4581,#4582));
#2160=EDGE_LOOP('',(#4583,#4584,#4585,#4586,#4587,#4588,#4589,#4590,#4591,
#4592,#4593,#4594,#4595,#4596,#4597,#4598,#4599,#4600,#4601,#4602,#4603,
#4604,#4605,#4606,#4607,#4608,#4609,#4610,#4611,#4612,#4613,#4614,#4615,
#4616,#4617));
#2161=EDGE_LOOP('',(#4618,#4619,#4620,#4621));
#2162=EDGE_LOOP('',(#4622,#4623,#4624,#4625));
#2163=EDGE_LOOP('',(#4626,#4627,#4628,#4629));
#2164=EDGE_LOOP('',(#4630,#4631,#4632,#4633,#4634,#4635,#4636,#4637,#4638,
#4639,#4640,#4641,#4642,#4643,#4644,#4645,#4646,#4647,#4648,#4649,#4650,
#4651,#4652,#4653,#4654,#4655,#4656,#4657,#4658,#4659,#4660,#4661,#4662,
#4663,#4664,#4665));
#2165=EDGE_LOOP('',(#4666,#4667,#4668,#4669,#4670,#4671,#4672,#4673,#4674,
#4675,#4676,#4677,#4678,#4679,#4680,#4681,#4682,#4683,#4684,#4685,#4686,
#4687,#4688,#4689,#4690,#4691,#4692,#4693,#4694,#4695,#4696,#4697,#4698,
#4699,#4700));
#2166=EDGE_LOOP('',(#4701,#4702,#4703,#4704));
#2167=EDGE_LOOP('',(#4705));
#2168=EDGE_LOOP('',(#4706));
#2169=EDGE_LOOP('',(#4707,#4708,#4709,#4710));
#2170=EDGE_LOOP('',(#4711,#4712,#4713,#4714));
#2171=EDGE_LOOP('',(#4715,#4716,#4717,#4718));
#2172=EDGE_LOOP('',(#4719,#4720,#4721,#4722));
#2173=EDGE_LOOP('',(#4723,#4724,#4725,#4726));
#2174=EDGE_LOOP('',(#4727,#4728,#4729,#4730));
#2175=EDGE_LOOP('',(#4731,#4732,#4733,#4734));
#2176=EDGE_LOOP('',(#4735,#4736,#4737,#4738));
#2177=EDGE_LOOP('',(#4739,#4740,#4741,#4742));
#2178=EDGE_LOOP('',(#4743));
#2179=EDGE_LOOP('',(#4744,#4745,#4746,#4747));
#2180=EDGE_LOOP('',(#4748,#4749,#4750,#4751));
#2181=EDGE_LOOP('',(#4752,#4753,#4754,#4755));
#2182=EDGE_LOOP('',(#4756,#4757,#4758,#4759,#4760,#4761,#4762,#4763,#4764,
#4765,#4766,#4767));
#2183=EDGE_LOOP('',(#4768,#4769,#4770,#4771));
#2184=EDGE_LOOP('',(#4772,#4773,#4774,#4775));
#2185=EDGE_LOOP('',(#4776,#4777,#4778,#4779,#4780,#4781,#4782,#4783));
#2186=EDGE_LOOP('',(#4784));
#2187=EDGE_LOOP('',(#4785));
#2188=EDGE_LOOP('',(#4786,#4787,#4788,#4789));
#2189=EDGE_LOOP('',(#4790,#4791,#4792,#4793));
#2190=EDGE_LOOP('',(#4794,#4795,#4796,#4797,#4798,#4799,#4800,#4801,#4802,
#4803,#4804,#4805,#4806,#4807,#4808,#4809));
#2191=EDGE_LOOP('',(#4810));
#2192=EDGE_LOOP('',(#4811));
#2193=EDGE_LOOP('',(#4812,#4813,#4814,#4815));
#2194=EDGE_LOOP('',(#4816,#4817,#4818,#4819));
#2195=EDGE_LOOP('',(#4820,#4821,#4822,#4823));
#2196=EDGE_LOOP('',(#4824,#4825,#4826,#4827));
#2197=EDGE_LOOP('',(#4828,#4829,#4830,#4831));
#2198=EDGE_LOOP('',(#4832,#4833,#4834,#4835));
#2199=EDGE_LOOP('',(#4836,#4837,#4838,#4839));
#2200=EDGE_LOOP('',(#4840,#4841,#4842,#4843));
#2201=EDGE_LOOP('',(#4844,#4845,#4846,#4847,#4848,#4849,#4850,#4851));
#2202=EDGE_LOOP('',(#4852,#4853,#4854,#4855));
#2203=EDGE_LOOP('',(#4856,#4857,#4858,#4859));
#2204=EDGE_LOOP('',(#4860,#4861,#4862,#4863));
#2205=EDGE_LOOP('',(#4864,#4865,#4866,#4867,#4868,#4869,#4870,#4871));
#2206=EDGE_LOOP('',(#4872,#4873,#4874,#4875));
#2207=EDGE_LOOP('',(#4876,#4877,#4878,#4879));
#2208=EDGE_LOOP('',(#4880,#4881,#4882,#4883));
#2209=EDGE_LOOP('',(#4884,#4885,#4886,#4887));
#2210=EDGE_LOOP('',(#4888,#4889,#4890,#4891));
#2211=EDGE_LOOP('',(#4892,#4893,#4894,#4895));
#2212=EDGE_LOOP('',(#4896,#4897,#4898,#4899));
#2213=EDGE_LOOP('',(#4900,#4901,#4902,#4903));
#2214=EDGE_LOOP('',(#4904,#4905,#4906,#4907,#4908,#4909,#4910,#4911,#4912,
#4913,#4914,#4915));
#2215=EDGE_LOOP('',(#4916));
#2216=EDGE_LOOP('',(#4917,#4918,#4919,#4920));
#2217=EDGE_LOOP('',(#4921,#4922,#4923,#4924));
#2490=CIRCLE('',#6705,1.666);
#2491=CIRCLE('',#6706,1.666);
#2492=CIRCLE('',#6721,1.666);
#2493=CIRCLE('',#6723,2.05475);
#2494=CIRCLE('',#6739,2.05475);
#2495=CIRCLE('',#6741,1.666);
#2496=CIRCLE('',#6742,1.666);
#2497=CIRCLE('',#6757,1.666);
#2498=CIRCLE('',#6759,2.05475);
#2499=CIRCLE('',#6775,2.05475);
#2500=CIRCLE('',#6785,2.);
#2501=CIRCLE('',#6786,2.);
#2502=CIRCLE('',#6788,4.);
#2503=CIRCLE('',#6789,4.);
#2504=CIRCLE('',#6791,4.);
#2505=CIRCLE('',#6792,4.);
#2674=VERTEX_POINT('',#8908);
#2675=VERTEX_POINT('',#8909);
#2676=VERTEX_POINT('',#8911);
#2677=VERTEX_POINT('',#8931);
#2678=VERTEX_POINT('',#8933);
#2679=VERTEX_POINT('',#8938);
#2680=VERTEX_POINT('',#8964);
#2681=VERTEX_POINT('',#8965);
#2682=VERTEX_POINT('',#9015);
#2683=VERTEX_POINT('',#9016);
#2684=VERTEX_POINT('',#9063);
#2685=VERTEX_POINT('',#9064);
#2686=VERTEX_POINT('',#9114);
#2687=VERTEX_POINT('',#9115);
#2688=VERTEX_POINT('',#9165);
#2689=VERTEX_POINT('',#9166);
#2690=VERTEX_POINT('',#9213);
#2691=VERTEX_POINT('',#9214);
#2692=VERTEX_POINT('',#9261);
#2693=VERTEX_POINT('',#9262);
#2694=VERTEX_POINT('',#9312);
#2695=VERTEX_POINT('',#9313);
#2696=VERTEX_POINT('',#9360);
#2697=VERTEX_POINT('',#9361);
#2698=VERTEX_POINT('',#9408);
#2699=VERTEX_POINT('',#9409);
#2700=VERTEX_POINT('',#9459);
#2701=VERTEX_POINT('',#9460);
#2702=VERTEX_POINT('',#9510);
#2703=VERTEX_POINT('',#9511);
#2704=VERTEX_POINT('',#9558);
#2705=VERTEX_POINT('',#9559);
#2706=VERTEX_POINT('',#9609);
#2707=VERTEX_POINT('',#9610);
#2708=VERTEX_POINT('',#9612);
#2709=VERTEX_POINT('',#9626);
#2710=VERTEX_POINT('',#9648);
#2711=VERTEX_POINT('',#9649);
#2712=VERTEX_POINT('',#9651);
#2713=VERTEX_POINT('',#9658);
#2714=VERTEX_POINT('',#9668);
#2715=VERTEX_POINT('',#9669);
#2716=VERTEX_POINT('',#9692);
#2717=VERTEX_POINT('',#9693);
#2718=VERTEX_POINT('',#9717);
#2719=VERTEX_POINT('',#9718);
#2720=VERTEX_POINT('',#9742);
#2721=VERTEX_POINT('',#9743);
#2722=VERTEX_POINT('',#9766);
#2723=VERTEX_POINT('',#9767);
#2724=VERTEX_POINT('',#9791);
#2725=VERTEX_POINT('',#9792);
#2726=VERTEX_POINT('',#9815);
#2727=VERTEX_POINT('',#9816);
#2728=VERTEX_POINT('',#9840);
#2729=VERTEX_POINT('',#9841);
#2730=VERTEX_POINT('',#9865);
#2731=VERTEX_POINT('',#9866);
#2732=VERTEX_POINT('',#9889);
#2733=VERTEX_POINT('',#9890);
#2734=VERTEX_POINT('',#9914);
#2735=VERTEX_POINT('',#9915);
#2736=VERTEX_POINT('',#9938);
#2737=VERTEX_POINT('',#9939);
#2738=VERTEX_POINT('',#9963);
#2739=VERTEX_POINT('',#9964);
#2740=VERTEX_POINT('',#9988);
#2741=VERTEX_POINT('',#9989);
#2742=VERTEX_POINT('',#10012);
#2743=VERTEX_POINT('',#10013);
#2744=VERTEX_POINT('',#10015);
#2745=VERTEX_POINT('',#10021);
#2746=VERTEX_POINT('',#10029);
#2747=VERTEX_POINT('',#10030);
#2748=VERTEX_POINT('',#10032);
#2749=VERTEX_POINT('',#10052);
#2750=VERTEX_POINT('',#10054);
#2751=VERTEX_POINT('',#10059);
#2752=VERTEX_POINT('',#10085);
#2753=VERTEX_POINT('',#10086);
#2754=VERTEX_POINT('',#10136);
#2755=VERTEX_POINT('',#10137);
#2756=VERTEX_POINT('',#10184);
#2757=VERTEX_POINT('',#10185);
#2758=VERTEX_POINT('',#10235);
#2759=VERTEX_POINT('',#10236);
#2760=VERTEX_POINT('',#10286);
#2761=VERTEX_POINT('',#10287);
#2762=VERTEX_POINT('',#10334);
#2763=VERTEX_POINT('',#10335);
#2764=VERTEX_POINT('',#10382);
#2765=VERTEX_POINT('',#10383);
#2766=VERTEX_POINT('',#10433);
#2767=VERTEX_POINT('',#10434);
#2768=VERTEX_POINT('',#10481);
#2769=VERTEX_POINT('',#10482);
#2770=VERTEX_POINT('',#10529);
#2771=VERTEX_POINT('',#10530);
#2772=VERTEX_POINT('',#10580);
#2773=VERTEX_POINT('',#10581);
#2774=VERTEX_POINT('',#10631);
#2775=VERTEX_POINT('',#10632);
#2776=VERTEX_POINT('',#10679);
#2777=VERTEX_POINT('',#10680);
#2778=VERTEX_POINT('',#10730);
#2779=VERTEX_POINT('',#10731);
#2780=VERTEX_POINT('',#10733);
#2781=VERTEX_POINT('',#10747);
#2782=VERTEX_POINT('',#10769);
#2783=VERTEX_POINT('',#10770);
#2784=VERTEX_POINT('',#10772);
#2785=VERTEX_POINT('',#10779);
#2786=VERTEX_POINT('',#10789);
#2787=VERTEX_POINT('',#10790);
#2788=VERTEX_POINT('',#10813);
#2789=VERTEX_POINT('',#10814);
#2790=VERTEX_POINT('',#10838);
#2791=VERTEX_POINT('',#10839);
#2792=VERTEX_POINT('',#10863);
#2793=VERTEX_POINT('',#10864);
#2794=VERTEX_POINT('',#10887);
#2795=VERTEX_POINT('',#10888);
#2796=VERTEX_POINT('',#10912);
#2797=VERTEX_POINT('',#10913);
#2798=VERTEX_POINT('',#10936);
#2799=VERTEX_POINT('',#10937);
#2800=VERTEX_POINT('',#10961);
#2801=VERTEX_POINT('',#10962);
#2802=VERTEX_POINT('',#10986);
#2803=VERTEX_POINT('',#10987);
#2804=VERTEX_POINT('',#11010);
#2805=VERTEX_POINT('',#11011);
#2806=VERTEX_POINT('',#11035);
#2807=VERTEX_POINT('',#11036);
#2808=VERTEX_POINT('',#11059);
#2809=VERTEX_POINT('',#11060);
#2810=VERTEX_POINT('',#11084);
#2811=VERTEX_POINT('',#11085);
#2812=VERTEX_POINT('',#11109);
#2813=VERTEX_POINT('',#11110);
#2814=VERTEX_POINT('',#11133);
#2815=VERTEX_POINT('',#11134);
#2816=VERTEX_POINT('',#11136);
#2817=VERTEX_POINT('',#11142);
#2818=VERTEX_POINT('',#13638);
#2819=VERTEX_POINT('',#13640);
#2820=VERTEX_POINT('',#13644);
#2821=VERTEX_POINT('',#13646);
#2822=VERTEX_POINT('',#13650);
#2823=VERTEX_POINT('',#13652);
#2824=VERTEX_POINT('',#13656);
#2825=VERTEX_POINT('',#13657);
#2826=VERTEX_POINT('',#13659);
#2827=VERTEX_POINT('',#13661);
#2828=VERTEX_POINT('',#13665);
#2829=VERTEX_POINT('',#13666);
#2830=VERTEX_POINT('',#13668);
#2831=VERTEX_POINT('',#13670);
#2832=VERTEX_POINT('',#13677);
#2833=VERTEX_POINT('',#13679);
#2834=VERTEX_POINT('',#13683);
#2835=VERTEX_POINT('',#13685);
#2836=VERTEX_POINT('',#13689);
#2837=VERTEX_POINT('',#13690);
#2838=VERTEX_POINT('',#13692);
#2839=VERTEX_POINT('',#13694);
#2840=VERTEX_POINT('',#13698);
#2841=VERTEX_POINT('',#13700);
#2842=VERTEX_POINT('',#13704);
#2843=VERTEX_POINT('',#13706);
#2844=VERTEX_POINT('',#13712);
#2845=VERTEX_POINT('',#13714);
#2846=VERTEX_POINT('',#13716);
#2847=VERTEX_POINT('',#13718);
#2848=VERTEX_POINT('',#13720);
#2849=VERTEX_POINT('',#13722);
#2850=VERTEX_POINT('',#13724);
#2851=VERTEX_POINT('',#13726);
#2852=VERTEX_POINT('',#13729);
#2853=VERTEX_POINT('',#13730);
#2854=VERTEX_POINT('',#13732);
#2855=VERTEX_POINT('',#13734);
#2856=VERTEX_POINT('',#13737);
#2857=VERTEX_POINT('',#13738);
#2858=VERTEX_POINT('',#13740);
#2859=VERTEX_POINT('',#13742);
#2860=VERTEX_POINT('',#13753);
#2861=VERTEX_POINT('',#13755);
#2862=VERTEX_POINT('',#13757);
#2863=VERTEX_POINT('',#13759);
#2864=VERTEX_POINT('',#13761);
#2865=VERTEX_POINT('',#13763);
#2866=VERTEX_POINT('',#13767);
#2867=VERTEX_POINT('',#13768);
#2868=VERTEX_POINT('',#13773);
#2869=VERTEX_POINT('',#13777);
#2870=VERTEX_POINT('',#13783);
#2871=VERTEX_POINT('',#13784);
#2872=VERTEX_POINT('',#13789);
#2873=VERTEX_POINT('',#13793);
#2874=VERTEX_POINT('',#13799);
#2875=VERTEX_POINT('',#13800);
#2876=VERTEX_POINT('',#13803);
#2877=VERTEX_POINT('',#13805);
#2878=VERTEX_POINT('',#13807);
#2879=VERTEX_POINT('',#13809);
#2880=VERTEX_POINT('',#13813);
#2881=VERTEX_POINT('',#13817);
#2882=VERTEX_POINT('',#13819);
#2883=VERTEX_POINT('',#13823);
#2884=VERTEX_POINT('',#13827);
#2885=VERTEX_POINT('',#13829);
#2886=VERTEX_POINT('',#13837);
#2887=VERTEX_POINT('',#13841);
#3300=EDGE_CURVE('',#2674,#2675,#561,.T.);
#3301=EDGE_CURVE('',#2675,#2676,#127,.T.);
#3302=EDGE_CURVE('',#2676,#2677,#2490,.T.);
#3303=EDGE_CURVE('',#2677,#2678,#128,.T.);
#3304=EDGE_CURVE('',#2678,#2679,#562,.T.);
#3305=EDGE_CURVE('',#2679,#2679,#2491,.F.);
#3306=EDGE_CURVE('',#2678,#2674,#129,.T.);
#3307=EDGE_CURVE('',#2680,#2681,#563,.T.);
#3308=EDGE_CURVE('',#2681,#2675,#130,.T.);
#3309=EDGE_CURVE('',#2674,#2680,#131,.T.);
#3310=EDGE_CURVE('',#2682,#2683,#564,.T.);
#3311=EDGE_CURVE('',#2683,#2681,#132,.T.);
#3312=EDGE_CURVE('',#2680,#2682,#133,.T.);
#3313=EDGE_CURVE('',#2684,#2685,#565,.T.);
#3314=EDGE_CURVE('',#2685,#2683,#134,.T.);
#3315=EDGE_CURVE('',#2682,#2684,#135,.T.);
#3316=EDGE_CURVE('',#2686,#2687,#566,.T.);
#3317=EDGE_CURVE('',#2687,#2685,#136,.T.);
#3318=EDGE_CURVE('',#2684,#2686,#137,.T.);
#3319=EDGE_CURVE('',#2688,#2689,#567,.T.);
#3320=EDGE_CURVE('',#2689,#2687,#138,.T.);
#3321=EDGE_CURVE('',#2686,#2688,#139,.T.);
#3322=EDGE_CURVE('',#2690,#2691,#568,.T.);
#3323=EDGE_CURVE('',#2691,#2689,#140,.T.);
#3324=EDGE_CURVE('',#2688,#2690,#141,.T.);
#3325=EDGE_CURVE('',#2692,#2693,#569,.T.);
#3326=EDGE_CURVE('',#2693,#2691,#142,.T.);
#3327=EDGE_CURVE('',#2690,#2692,#143,.T.);
#3328=EDGE_CURVE('',#2694,#2695,#570,.T.);
#3329=EDGE_CURVE('',#2695,#2693,#144,.T.);
#3330=EDGE_CURVE('',#2692,#2694,#145,.T.);
#3331=EDGE_CURVE('',#2696,#2697,#571,.T.);
#3332=EDGE_CURVE('',#2697,#2695,#146,.T.);
#3333=EDGE_CURVE('',#2694,#2696,#147,.T.);
#3334=EDGE_CURVE('',#2698,#2699,#572,.T.);
#3335=EDGE_CURVE('',#2699,#2697,#148,.T.);
#3336=EDGE_CURVE('',#2696,#2698,#149,.T.);
#3337=EDGE_CURVE('',#2700,#2701,#573,.T.);
#3338=EDGE_CURVE('',#2701,#2699,#150,.T.);
#3339=EDGE_CURVE('',#2698,#2700,#151,.T.);
#3340=EDGE_CURVE('',#2702,#2703,#574,.T.);
#3341=EDGE_CURVE('',#2703,#2701,#152,.T.);
#3342=EDGE_CURVE('',#2700,#2702,#153,.T.);
#3343=EDGE_CURVE('',#2704,#2705,#575,.T.);
#3344=EDGE_CURVE('',#2705,#2703,#154,.T.);
#3345=EDGE_CURVE('',#2702,#2704,#155,.T.);
#3346=EDGE_CURVE('',#2706,#2707,#576,.T.);
#3347=EDGE_CURVE('',#2706,#2708,#156,.T.);
#3348=EDGE_CURVE('',#2709,#2708,#2492,.T.);
#3349=EDGE_CURVE('',#2709,#2707,#157,.T.);
#3350=EDGE_CURVE('',#2710,#2711,#577,.T.);
#3351=EDGE_CURVE('',#2711,#2712,#158,.T.);
#3352=EDGE_CURVE('',#2713,#2712,#2493,.T.);
#3353=EDGE_CURVE('',#2710,#2713,#159,.T.);
#3354=EDGE_CURVE('',#2714,#2715,#578,.T.);
#3355=EDGE_CURVE('',#2715,#2711,#160,.T.);
#3356=EDGE_CURVE('',#2714,#2710,#161,.T.);
#3357=EDGE_CURVE('',#2716,#2717,#579,.T.);
#3358=EDGE_CURVE('',#2717,#2715,#162,.T.);
#3359=EDGE_CURVE('',#2716,#2714,#163,.T.);
#3360=EDGE_CURVE('',#2718,#2719,#580,.T.);
#3361=EDGE_CURVE('',#2719,#2717,#164,.T.);
#3362=EDGE_CURVE('',#2718,#2716,#165,.T.);
#3363=EDGE_CURVE('',#2720,#2721,#581,.T.);
#3364=EDGE_CURVE('',#2721,#2719,#166,.T.);
#3365=EDGE_CURVE('',#2720,#2718,#167,.T.);
#3366=EDGE_CURVE('',#2722,#2723,#582,.T.);
#3367=EDGE_CURVE('',#2723,#2721,#168,.T.);
#3368=EDGE_CURVE('',#2722,#2720,#169,.T.);
#3369=EDGE_CURVE('',#2724,#2725,#583,.T.);
#3370=EDGE_CURVE('',#2725,#2723,#170,.T.);
#3371=EDGE_CURVE('',#2724,#2722,#171,.T.);
#3372=EDGE_CURVE('',#2726,#2727,#584,.T.);
#3373=EDGE_CURVE('',#2727,#2725,#172,.T.);
#3374=EDGE_CURVE('',#2726,#2724,#173,.T.);
#3375=EDGE_CURVE('',#2728,#2729,#585,.T.);
#3376=EDGE_CURVE('',#2729,#2727,#174,.T.);
#3377=EDGE_CURVE('',#2728,#2726,#175,.T.);
#3378=EDGE_CURVE('',#2730,#2731,#586,.T.);
#3379=EDGE_CURVE('',#2731,#2729,#176,.T.);
#3380=EDGE_CURVE('',#2730,#2728,#177,.T.);
#3381=EDGE_CURVE('',#2732,#2733,#587,.T.);
#3382=EDGE_CURVE('',#2733,#2731,#178,.T.);
#3383=EDGE_CURVE('',#2732,#2730,#179,.T.);
#3384=EDGE_CURVE('',#2734,#2735,#588,.T.);
#3385=EDGE_CURVE('',#2735,#2733,#180,.T.);
#3386=EDGE_CURVE('',#2734,#2732,#181,.T.);
#3387=EDGE_CURVE('',#2736,#2737,#589,.T.);
#3388=EDGE_CURVE('',#2737,#2735,#182,.T.);
#3389=EDGE_CURVE('',#2736,#2734,#183,.T.);
#3390=EDGE_CURVE('',#2738,#2739,#590,.T.);
#3391=EDGE_CURVE('',#2739,#2737,#184,.T.);
#3392=EDGE_CURVE('',#2738,#2736,#185,.T.);
#3393=EDGE_CURVE('',#2740,#2741,#591,.T.);
#3394=EDGE_CURVE('',#2741,#2739,#186,.T.);
#3395=EDGE_CURVE('',#2740,#2738,#187,.T.);
#3396=EDGE_CURVE('',#2742,#2743,#592,.T.);
#3397=EDGE_CURVE('',#2744,#2742,#188,.T.);
#3398=EDGE_CURVE('',#2745,#2744,#2494,.T.);
#3399=EDGE_CURVE('',#2745,#2743,#189,.T.);
#3400=EDGE_CURVE('',#2746,#2747,#593,.T.);
#3401=EDGE_CURVE('',#2747,#2748,#190,.T.);
#3402=EDGE_CURVE('',#2748,#2749,#2495,.T.);
#3403=EDGE_CURVE('',#2749,#2750,#191,.T.);
#3404=EDGE_CURVE('',#2750,#2751,#594,.T.);
#3405=EDGE_CURVE('',#2751,#2751,#2496,.F.);
#3406=EDGE_CURVE('',#2750,#2746,#192,.T.);
#3407=EDGE_CURVE('',#2752,#2753,#595,.T.);
#3408=EDGE_CURVE('',#2753,#2747,#193,.T.);
#3409=EDGE_CURVE('',#2746,#2752,#194,.T.);
#3410=EDGE_CURVE('',#2754,#2755,#596,.T.);
#3411=EDGE_CURVE('',#2755,#2753,#195,.T.);
#3412=EDGE_CURVE('',#2752,#2754,#196,.T.);
#3413=EDGE_CURVE('',#2756,#2757,#597,.T.);
#3414=EDGE_CURVE('',#2757,#2755,#197,.T.);
#3415=EDGE_CURVE('',#2754,#2756,#198,.T.);
#3416=EDGE_CURVE('',#2758,#2759,#598,.T.);
#3417=EDGE_CURVE('',#2759,#2757,#199,.T.);
#3418=EDGE_CURVE('',#2756,#2758,#200,.T.);
#3419=EDGE_CURVE('',#2760,#2761,#599,.T.);
#3420=EDGE_CURVE('',#2761,#2759,#201,.T.);
#3421=EDGE_CURVE('',#2758,#2760,#202,.T.);
#3422=EDGE_CURVE('',#2762,#2763,#600,.T.);
#3423=EDGE_CURVE('',#2763,#2761,#203,.T.);
#3424=EDGE_CURVE('',#2760,#2762,#204,.T.);
#3425=EDGE_CURVE('',#2764,#2765,#601,.T.);
#3426=EDGE_CURVE('',#2765,#2763,#205,.T.);
#3427=EDGE_CURVE('',#2762,#2764,#206,.T.);
#3428=EDGE_CURVE('',#2766,#2767,#602,.T.);
#3429=EDGE_CURVE('',#2767,#2765,#207,.T.);
#3430=EDGE_CURVE('',#2764,#2766,#208,.T.);
#3431=EDGE_CURVE('',#2768,#2769,#603,.T.);
#3432=EDGE_CURVE('',#2769,#2767,#209,.T.);
#3433=EDGE_CURVE('',#2766,#2768,#210,.T.);
#3434=EDGE_CURVE('',#2770,#2771,#604,.T.);
#3435=EDGE_CURVE('',#2771,#2769,#211,.T.);
#3436=EDGE_CURVE('',#2768,#2770,#212,.T.);
#3437=EDGE_CURVE('',#2772,#2773,#605,.T.);
#3438=EDGE_CURVE('',#2773,#2771,#213,.T.);
#3439=EDGE_CURVE('',#2770,#2772,#214,.T.);
#3440=EDGE_CURVE('',#2774,#2775,#606,.T.);
#3441=EDGE_CURVE('',#2775,#2773,#215,.T.);
#3442=EDGE_CURVE('',#2772,#2774,#216,.T.);
#3443=EDGE_CURVE('',#2776,#2777,#607,.T.);
#3444=EDGE_CURVE('',#2777,#2775,#217,.T.);
#3445=EDGE_CURVE('',#2774,#2776,#218,.T.);
#3446=EDGE_CURVE('',#2778,#2779,#608,.T.);
#3447=EDGE_CURVE('',#2778,#2780,#219,.T.);
#3448=EDGE_CURVE('',#2781,#2780,#2497,.T.);
#3449=EDGE_CURVE('',#2781,#2779,#220,.T.);
#3450=EDGE_CURVE('',#2782,#2783,#609,.T.);
#3451=EDGE_CURVE('',#2783,#2784,#221,.T.);
#3452=EDGE_CURVE('',#2785,#2784,#2498,.T.);
#3453=EDGE_CURVE('',#2782,#2785,#222,.T.);
#3454=EDGE_CURVE('',#2786,#2787,#610,.T.);
#3455=EDGE_CURVE('',#2787,#2783,#223,.T.);
#3456=EDGE_CURVE('',#2786,#2782,#224,.T.);
#3457=EDGE_CURVE('',#2788,#2789,#611,.T.);
#3458=EDGE_CURVE('',#2789,#2787,#225,.T.);
#3459=EDGE_CURVE('',#2788,#2786,#226,.T.);
#3460=EDGE_CURVE('',#2790,#2791,#612,.T.);
#3461=EDGE_CURVE('',#2791,#2789,#227,.T.);
#3462=EDGE_CURVE('',#2790,#2788,#228,.T.);
#3463=EDGE_CURVE('',#2792,#2793,#613,.T.);
#3464=EDGE_CURVE('',#2793,#2791,#229,.T.);
#3465=EDGE_CURVE('',#2792,#2790,#230,.T.);
#3466=EDGE_CURVE('',#2794,#2795,#614,.T.);
#3467=EDGE_CURVE('',#2795,#2793,#231,.T.);
#3468=EDGE_CURVE('',#2794,#2792,#232,.T.);
#3469=EDGE_CURVE('',#2796,#2797,#615,.T.);
#3470=EDGE_CURVE('',#2797,#2795,#233,.T.);
#3471=EDGE_CURVE('',#2796,#2794,#234,.T.);
#3472=EDGE_CURVE('',#2798,#2799,#616,.T.);
#3473=EDGE_CURVE('',#2799,#2797,#235,.T.);
#3474=EDGE_CURVE('',#2798,#2796,#236,.T.);
#3475=EDGE_CURVE('',#2800,#2801,#617,.T.);
#3476=EDGE_CURVE('',#2801,#2799,#237,.T.);
#3477=EDGE_CURVE('',#2800,#2798,#238,.T.);
#3478=EDGE_CURVE('',#2802,#2803,#618,.T.);
#3479=EDGE_CURVE('',#2803,#2801,#239,.T.);
#3480=EDGE_CURVE('',#2802,#2800,#240,.T.);
#3481=EDGE_CURVE('',#2804,#2805,#619,.T.);
#3482=EDGE_CURVE('',#2805,#2803,#241,.T.);
#3483=EDGE_CURVE('',#2804,#2802,#242,.T.);
#3484=EDGE_CURVE('',#2806,#2807,#620,.T.);
#3485=EDGE_CURVE('',#2807,#2805,#243,.T.);
#3486=EDGE_CURVE('',#2806,#2804,#244,.T.);
#3487=EDGE_CURVE('',#2808,#2809,#621,.T.);
#3488=EDGE_CURVE('',#2809,#2807,#245,.T.);
#3489=EDGE_CURVE('',#2808,#2806,#246,.T.);
#3490=EDGE_CURVE('',#2810,#2811,#622,.T.);
#3491=EDGE_CURVE('',#2811,#2809,#247,.T.);
#3492=EDGE_CURVE('',#2810,#2808,#248,.T.);
#3493=EDGE_CURVE('',#2812,#2813,#623,.T.);
#3494=EDGE_CURVE('',#2813,#2811,#249,.T.);
#3495=EDGE_CURVE('',#2812,#2810,#250,.T.);
#3496=EDGE_CURVE('',#2814,#2815,#624,.T.);
#3497=EDGE_CURVE('',#2816,#2814,#251,.T.);
#3498=EDGE_CURVE('',#2817,#2816,#2499,.T.);
#3499=EDGE_CURVE('',#2817,#2815,#252,.T.);
#3500=EDGE_CURVE('',#2748,#2785,#253,.T.);
#3501=EDGE_CURVE('',#2784,#2749,#254,.T.);
#3502=EDGE_CURVE('',#2815,#2813,#255,.T.);
#3503=EDGE_CURVE('',#2814,#2812,#256,.T.);
#3504=EDGE_CURVE('',#2780,#2817,#257,.T.);
#3505=EDGE_CURVE('',#2776,#2778,#258,.T.);
#3506=EDGE_CURVE('',#2779,#2777,#259,.T.);
#3507=EDGE_CURVE('',#2816,#2781,#260,.T.);
#3508=EDGE_CURVE('',#2676,#2713,#261,.T.);
#3509=EDGE_CURVE('',#2712,#2677,#262,.T.);
#3510=EDGE_CURVE('',#2743,#2741,#263,.T.);
#3511=EDGE_CURVE('',#2742,#2740,#264,.T.);
#3512=EDGE_CURVE('',#2708,#2745,#265,.T.);
#3513=EDGE_CURVE('',#2704,#2706,#266,.T.);
#3514=EDGE_CURVE('',#2707,#2705,#267,.T.);
#3515=EDGE_CURVE('',#2744,#2709,#268,.T.);
#3516=EDGE_CURVE('',#2818,#2818,#2500,.T.);
#3517=EDGE_CURVE('',#2818,#2819,#625,.T.);
#3518=EDGE_CURVE('',#2819,#2819,#2501,.T.);
#3519=EDGE_CURVE('',#2820,#2820,#2502,.T.);
#3520=EDGE_CURVE('',#2820,#2821,#626,.T.);
#3521=EDGE_CURVE('',#2821,#2821,#2503,.T.);
#3522=EDGE_CURVE('',#2822,#2822,#2504,.T.);
#3523=EDGE_CURVE('',#2822,#2823,#627,.T.);
#3524=EDGE_CURVE('',#2823,#2823,#2505,.T.);
#3525=EDGE_CURVE('',#2824,#2825,#628,.T.);
#3526=EDGE_CURVE('',#2826,#2824,#629,.T.);
#3527=EDGE_CURVE('',#2826,#2827,#630,.T.);
#3528=EDGE_CURVE('',#2827,#2825,#631,.T.);
#3529=EDGE_CURVE('',#2828,#2829,#632,.T.);
#3530=EDGE_CURVE('',#2830,#2828,#633,.T.);
#3531=EDGE_CURVE('',#2830,#2831,#634,.T.);
#3532=EDGE_CURVE('',#2831,#2829,#635,.T.);
#3533=EDGE_CURVE('',#2831,#2826,#636,.T.);
#3534=EDGE_CURVE('',#2827,#2830,#637,.T.);
#3535=EDGE_CURVE('',#2832,#2825,#638,.T.);
#3536=EDGE_CURVE('',#2833,#2832,#639,.T.);
#3537=EDGE_CURVE('',#2824,#2833,#640,.T.);
#3538=EDGE_CURVE('',#2834,#2829,#641,.T.);
#3539=EDGE_CURVE('',#2835,#2834,#642,.T.);
#3540=EDGE_CURVE('',#2828,#2835,#643,.T.);
#3541=EDGE_CURVE('',#2836,#2837,#644,.T.);
#3542=EDGE_CURVE('',#2838,#2836,#645,.T.);
#3543=EDGE_CURVE('',#2838,#2839,#646,.T.);
#3544=EDGE_CURVE('',#2839,#2837,#647,.T.);
#3545=EDGE_CURVE('',#2840,#2836,#648,.T.);
#3546=EDGE_CURVE('',#2841,#2840,#649,.T.);
#3547=EDGE_CURVE('',#2841,#2838,#650,.T.);
#3548=EDGE_CURVE('',#2837,#2842,#651,.T.);
#3549=EDGE_CURVE('',#2839,#2843,#652,.T.);
#3550=EDGE_CURVE('',#2843,#2842,#653,.T.);
#3551=EDGE_CURVE('',#2843,#2841,#654,.T.);
#3552=EDGE_CURVE('',#2844,#2842,#655,.T.);
#3553=EDGE_CURVE('',#2845,#2844,#656,.T.);
#3554=EDGE_CURVE('',#2846,#2845,#657,.T.);
#3555=EDGE_CURVE('',#2846,#2847,#658,.T.);
#3556=EDGE_CURVE('',#2847,#2848,#659,.T.);
#3557=EDGE_CURVE('',#2848,#2849,#660,.T.);
#3558=EDGE_CURVE('',#2850,#2849,#661,.T.);
#3559=EDGE_CURVE('',#2851,#2850,#662,.T.);
#3560=EDGE_CURVE('',#2840,#2851,#663,.T.);
#3561=EDGE_CURVE('',#2852,#2853,#664,.T.);
#3562=EDGE_CURVE('',#2853,#2854,#665,.T.);
#3563=EDGE_CURVE('',#2854,#2855,#666,.T.);
#3564=EDGE_CURVE('',#2855,#2852,#667,.T.);
#3565=EDGE_CURVE('',#2856,#2857,#668,.T.);
#3566=EDGE_CURVE('',#2857,#2858,#669,.T.);
#3567=EDGE_CURVE('',#2858,#2859,#670,.T.);
#3568=EDGE_CURVE('',#2859,#2856,#671,.T.);
#3569=EDGE_CURVE('',#2833,#2848,#672,.T.);
#3570=EDGE_CURVE('',#2834,#2847,#673,.T.);
#3571=EDGE_CURVE('',#2835,#2846,#674,.T.);
#3572=EDGE_CURVE('',#2832,#2849,#675,.T.);
#3573=EDGE_CURVE('',#2845,#2860,#676,.T.);
#3574=EDGE_CURVE('',#2861,#2860,#677,.T.);
#3575=EDGE_CURVE('',#2861,#2862,#678,.T.);
#3576=EDGE_CURVE('',#2862,#2863,#679,.T.);
#3577=EDGE_CURVE('',#2863,#2864,#680,.T.);
#3578=EDGE_CURVE('',#2865,#2864,#681,.T.);
#3579=EDGE_CURVE('',#2850,#2865,#682,.T.);
#3580=EDGE_CURVE('',#2866,#2867,#683,.T.);
#3581=EDGE_CURVE('',#2866,#2857,#684,.T.);
#3582=EDGE_CURVE('',#2867,#2856,#685,.T.);
#3583=EDGE_CURVE('',#2868,#2866,#686,.T.);
#3584=EDGE_CURVE('',#2868,#2858,#687,.T.);
#3585=EDGE_CURVE('',#2869,#2868,#688,.T.);
#3586=EDGE_CURVE('',#2869,#2859,#689,.T.);
#3587=EDGE_CURVE('',#2867,#2869,#690,.T.);
#3588=EDGE_CURVE('',#2870,#2871,#691,.T.);
#3589=EDGE_CURVE('',#2870,#2853,#692,.T.);
#3590=EDGE_CURVE('',#2871,#2852,#693,.T.);
#3591=EDGE_CURVE('',#2872,#2870,#694,.T.);
#3592=EDGE_CURVE('',#2872,#2854,#695,.T.);
#3593=EDGE_CURVE('',#2873,#2872,#696,.T.);
#3594=EDGE_CURVE('',#2873,#2855,#697,.T.);
#3595=EDGE_CURVE('',#2871,#2873,#698,.T.);
#3596=EDGE_CURVE('',#2874,#2875,#699,.T.);
#3597=EDGE_CURVE('',#2864,#2874,#700,.T.);
#3598=EDGE_CURVE('',#2863,#2876,#701,.T.);
#3599=EDGE_CURVE('',#2876,#2877,#702,.T.);
#3600=EDGE_CURVE('',#2878,#2877,#703,.T.);
#3601=EDGE_CURVE('',#2879,#2878,#704,.T.);
#3602=EDGE_CURVE('',#2879,#2875,#705,.T.);
#3603=EDGE_CURVE('',#2880,#2862,#706,.T.);
#3604=EDGE_CURVE('',#2876,#2880,#707,.T.);
#3605=EDGE_CURVE('',#2875,#2881,#708,.T.);
#3606=EDGE_CURVE('',#2882,#2879,#709,.T.);
#3607=EDGE_CURVE('',#2881,#2882,#710,.T.);
#3608=EDGE_CURVE('',#2883,#2878,#711,.T.);
#3609=EDGE_CURVE('',#2882,#2883,#712,.T.);
#3610=EDGE_CURVE('',#2881,#2884,#713,.T.);
#3611=EDGE_CURVE('',#2885,#2883,#714,.T.);
#3612=EDGE_CURVE('',#2880,#2885,#715,.T.);
#3613=EDGE_CURVE('',#2884,#2861,#716,.T.);
#3614=EDGE_CURVE('',#2877,#2885,#717,.T.);
#3615=EDGE_CURVE('',#2874,#2886,#718,.T.);
#3616=EDGE_CURVE('',#2886,#2865,#719,.T.);
#3617=EDGE_CURVE('',#2860,#2887,#720,.T.);
#3618=EDGE_CURVE('',#2887,#2884,#721,.T.);
#3619=EDGE_CURVE('',#2851,#2886,#722,.T.);
#3620=EDGE_CURVE('',#2844,#2887,#723,.T.);
#4283=ORIENTED_EDGE('',*,*,#3300,.T.);
#4284=ORIENTED_EDGE('',*,*,#3301,.T.);
#4285=ORIENTED_EDGE('',*,*,#3302,.T.);
#4286=ORIENTED_EDGE('',*,*,#3303,.T.);
#4287=ORIENTED_EDGE('',*,*,#3304,.T.);
#4288=ORIENTED_EDGE('',*,*,#3305,.T.);
#4289=ORIENTED_EDGE('',*,*,#3304,.F.);
#4290=ORIENTED_EDGE('',*,*,#3306,.T.);
#4291=ORIENTED_EDGE('',*,*,#3307,.T.);
#4292=ORIENTED_EDGE('',*,*,#3308,.T.);
#4293=ORIENTED_EDGE('',*,*,#3300,.F.);
#4294=ORIENTED_EDGE('',*,*,#3309,.T.);
#4295=ORIENTED_EDGE('',*,*,#3310,.T.);
#4296=ORIENTED_EDGE('',*,*,#3311,.T.);
#4297=ORIENTED_EDGE('',*,*,#3307,.F.);
#4298=ORIENTED_EDGE('',*,*,#3312,.T.);
#4299=ORIENTED_EDGE('',*,*,#3313,.T.);
#4300=ORIENTED_EDGE('',*,*,#3314,.T.);
#4301=ORIENTED_EDGE('',*,*,#3310,.F.);
#4302=ORIENTED_EDGE('',*,*,#3315,.T.);
#4303=ORIENTED_EDGE('',*,*,#3316,.T.);
#4304=ORIENTED_EDGE('',*,*,#3317,.T.);
#4305=ORIENTED_EDGE('',*,*,#3313,.F.);
#4306=ORIENTED_EDGE('',*,*,#3318,.T.);
#4307=ORIENTED_EDGE('',*,*,#3319,.T.);
#4308=ORIENTED_EDGE('',*,*,#3320,.T.);
#4309=ORIENTED_EDGE('',*,*,#3316,.F.);
#4310=ORIENTED_EDGE('',*,*,#3321,.T.);
#4311=ORIENTED_EDGE('',*,*,#3322,.T.);
#4312=ORIENTED_EDGE('',*,*,#3323,.T.);
#4313=ORIENTED_EDGE('',*,*,#3319,.F.);
#4314=ORIENTED_EDGE('',*,*,#3324,.T.);
#4315=ORIENTED_EDGE('',*,*,#3325,.T.);
#4316=ORIENTED_EDGE('',*,*,#3326,.T.);
#4317=ORIENTED_EDGE('',*,*,#3322,.F.);
#4318=ORIENTED_EDGE('',*,*,#3327,.T.);
#4319=ORIENTED_EDGE('',*,*,#3328,.T.);
#4320=ORIENTED_EDGE('',*,*,#3329,.T.);
#4321=ORIENTED_EDGE('',*,*,#3325,.F.);
#4322=ORIENTED_EDGE('',*,*,#3330,.T.);
#4323=ORIENTED_EDGE('',*,*,#3331,.T.);
#4324=ORIENTED_EDGE('',*,*,#3332,.T.);
#4325=ORIENTED_EDGE('',*,*,#3328,.F.);
#4326=ORIENTED_EDGE('',*,*,#3333,.T.);
#4327=ORIENTED_EDGE('',*,*,#3334,.T.);
#4328=ORIENTED_EDGE('',*,*,#3335,.T.);
#4329=ORIENTED_EDGE('',*,*,#3331,.F.);
#4330=ORIENTED_EDGE('',*,*,#3336,.T.);
#4331=ORIENTED_EDGE('',*,*,#3337,.T.);
#4332=ORIENTED_EDGE('',*,*,#3338,.T.);
#4333=ORIENTED_EDGE('',*,*,#3334,.F.);
#4334=ORIENTED_EDGE('',*,*,#3339,.T.);
#4335=ORIENTED_EDGE('',*,*,#3340,.T.);
#4336=ORIENTED_EDGE('',*,*,#3341,.T.);
#4337=ORIENTED_EDGE('',*,*,#3337,.F.);
#4338=ORIENTED_EDGE('',*,*,#3342,.T.);
#4339=ORIENTED_EDGE('',*,*,#3343,.T.);
#4340=ORIENTED_EDGE('',*,*,#3344,.T.);
#4341=ORIENTED_EDGE('',*,*,#3340,.F.);
#4342=ORIENTED_EDGE('',*,*,#3345,.T.);
#4343=ORIENTED_EDGE('',*,*,#3346,.F.);
#4344=ORIENTED_EDGE('',*,*,#3347,.T.);
#4345=ORIENTED_EDGE('',*,*,#3348,.F.);
#4346=ORIENTED_EDGE('',*,*,#3349,.T.);
#4347=ORIENTED_EDGE('',*,*,#3350,.T.);
#4348=ORIENTED_EDGE('',*,*,#3351,.T.);
#4349=ORIENTED_EDGE('',*,*,#3352,.F.);
#4350=ORIENTED_EDGE('',*,*,#3353,.F.);
#4351=ORIENTED_EDGE('',*,*,#3354,.T.);
#4352=ORIENTED_EDGE('',*,*,#3355,.T.);
#4353=ORIENTED_EDGE('',*,*,#3350,.F.);
#4354=ORIENTED_EDGE('',*,*,#3356,.F.);
#4355=ORIENTED_EDGE('',*,*,#3357,.T.);
#4356=ORIENTED_EDGE('',*,*,#3358,.T.);
#4357=ORIENTED_EDGE('',*,*,#3354,.F.);
#4358=ORIENTED_EDGE('',*,*,#3359,.F.);
#4359=ORIENTED_EDGE('',*,*,#3360,.T.);
#4360=ORIENTED_EDGE('',*,*,#3361,.T.);
#4361=ORIENTED_EDGE('',*,*,#3357,.F.);
#4362=ORIENTED_EDGE('',*,*,#3362,.F.);
#4363=ORIENTED_EDGE('',*,*,#3363,.T.);
#4364=ORIENTED_EDGE('',*,*,#3364,.T.);
#4365=ORIENTED_EDGE('',*,*,#3360,.F.);
#4366=ORIENTED_EDGE('',*,*,#3365,.F.);
#4367=ORIENTED_EDGE('',*,*,#3366,.T.);
#4368=ORIENTED_EDGE('',*,*,#3367,.T.);
#4369=ORIENTED_EDGE('',*,*,#3363,.F.);
#4370=ORIENTED_EDGE('',*,*,#3368,.F.);
#4371=ORIENTED_EDGE('',*,*,#3369,.T.);
#4372=ORIENTED_EDGE('',*,*,#3370,.T.);
#4373=ORIENTED_EDGE('',*,*,#3366,.F.);
#4374=ORIENTED_EDGE('',*,*,#3371,.F.);
#4375=ORIENTED_EDGE('',*,*,#3372,.T.);
#4376=ORIENTED_EDGE('',*,*,#3373,.T.);
#4377=ORIENTED_EDGE('',*,*,#3369,.F.);
#4378=ORIENTED_EDGE('',*,*,#3374,.F.);
#4379=ORIENTED_EDGE('',*,*,#3375,.T.);
#4380=ORIENTED_EDGE('',*,*,#3376,.T.);
#4381=ORIENTED_EDGE('',*,*,#3372,.F.);
#4382=ORIENTED_EDGE('',*,*,#3377,.F.);
#4383=ORIENTED_EDGE('',*,*,#3378,.T.);
#4384=ORIENTED_EDGE('',*,*,#3379,.T.);
#4385=ORIENTED_EDGE('',*,*,#3375,.F.);
#4386=ORIENTED_EDGE('',*,*,#3380,.F.);
#4387=ORIENTED_EDGE('',*,*,#3381,.T.);
#4388=ORIENTED_EDGE('',*,*,#3382,.T.);
#4389=ORIENTED_EDGE('',*,*,#3378,.F.);
#4390=ORIENTED_EDGE('',*,*,#3383,.F.);
#4391=ORIENTED_EDGE('',*,*,#3384,.T.);
#4392=ORIENTED_EDGE('',*,*,#3385,.T.);
#4393=ORIENTED_EDGE('',*,*,#3381,.F.);
#4394=ORIENTED_EDGE('',*,*,#3386,.F.);
#4395=ORIENTED_EDGE('',*,*,#3387,.T.);
#4396=ORIENTED_EDGE('',*,*,#3388,.T.);
#4397=ORIENTED_EDGE('',*,*,#3384,.F.);
#4398=ORIENTED_EDGE('',*,*,#3389,.F.);
#4399=ORIENTED_EDGE('',*,*,#3390,.T.);
#4400=ORIENTED_EDGE('',*,*,#3391,.T.);
#4401=ORIENTED_EDGE('',*,*,#3387,.F.);
#4402=ORIENTED_EDGE('',*,*,#3392,.F.);
#4403=ORIENTED_EDGE('',*,*,#3393,.T.);
#4404=ORIENTED_EDGE('',*,*,#3394,.T.);
#4405=ORIENTED_EDGE('',*,*,#3390,.F.);
#4406=ORIENTED_EDGE('',*,*,#3395,.F.);
#4407=ORIENTED_EDGE('',*,*,#3396,.F.);
#4408=ORIENTED_EDGE('',*,*,#3397,.F.);
#4409=ORIENTED_EDGE('',*,*,#3398,.F.);
#4410=ORIENTED_EDGE('',*,*,#3399,.T.);
#4411=ORIENTED_EDGE('',*,*,#3400,.T.);
#4412=ORIENTED_EDGE('',*,*,#3401,.T.);
#4413=ORIENTED_EDGE('',*,*,#3402,.T.);
#4414=ORIENTED_EDGE('',*,*,#3403,.T.);
#4415=ORIENTED_EDGE('',*,*,#3404,.T.);
#4416=ORIENTED_EDGE('',*,*,#3405,.T.);
#4417=ORIENTED_EDGE('',*,*,#3404,.F.);
#4418=ORIENTED_EDGE('',*,*,#3406,.T.);
#4419=ORIENTED_EDGE('',*,*,#3407,.T.);
#4420=ORIENTED_EDGE('',*,*,#3408,.T.);
#4421=ORIENTED_EDGE('',*,*,#3400,.F.);
#4422=ORIENTED_EDGE('',*,*,#3409,.T.);
#4423=ORIENTED_EDGE('',*,*,#3410,.T.);
#4424=ORIENTED_EDGE('',*,*,#3411,.T.);
#4425=ORIENTED_EDGE('',*,*,#3407,.F.);
#4426=ORIENTED_EDGE('',*,*,#3412,.T.);
#4427=ORIENTED_EDGE('',*,*,#3413,.T.);
#4428=ORIENTED_EDGE('',*,*,#3414,.T.);
#4429=ORIENTED_EDGE('',*,*,#3410,.F.);
#4430=ORIENTED_EDGE('',*,*,#3415,.T.);
#4431=ORIENTED_EDGE('',*,*,#3416,.T.);
#4432=ORIENTED_EDGE('',*,*,#3417,.T.);
#4433=ORIENTED_EDGE('',*,*,#3413,.F.);
#4434=ORIENTED_EDGE('',*,*,#3418,.T.);
#4435=ORIENTED_EDGE('',*,*,#3419,.T.);
#4436=ORIENTED_EDGE('',*,*,#3420,.T.);
#4437=ORIENTED_EDGE('',*,*,#3416,.F.);
#4438=ORIENTED_EDGE('',*,*,#3421,.T.);
#4439=ORIENTED_EDGE('',*,*,#3422,.T.);
#4440=ORIENTED_EDGE('',*,*,#3423,.T.);
#4441=ORIENTED_EDGE('',*,*,#3419,.F.);
#4442=ORIENTED_EDGE('',*,*,#3424,.T.);
#4443=ORIENTED_EDGE('',*,*,#3425,.T.);
#4444=ORIENTED_EDGE('',*,*,#3426,.T.);
#4445=ORIENTED_EDGE('',*,*,#3422,.F.);
#4446=ORIENTED_EDGE('',*,*,#3427,.T.);
#4447=ORIENTED_EDGE('',*,*,#3428,.T.);
#4448=ORIENTED_EDGE('',*,*,#3429,.T.);
#4449=ORIENTED_EDGE('',*,*,#3425,.F.);
#4450=ORIENTED_EDGE('',*,*,#3430,.T.);
#4451=ORIENTED_EDGE('',*,*,#3431,.T.);
#4452=ORIENTED_EDGE('',*,*,#3432,.T.);
#4453=ORIENTED_EDGE('',*,*,#3428,.F.);
#4454=ORIENTED_EDGE('',*,*,#3433,.T.);
#4455=ORIENTED_EDGE('',*,*,#3434,.T.);
#4456=ORIENTED_EDGE('',*,*,#3435,.T.);
#4457=ORIENTED_EDGE('',*,*,#3431,.F.);
#4458=ORIENTED_EDGE('',*,*,#3436,.T.);
#4459=ORIENTED_EDGE('',*,*,#3437,.T.);
#4460=ORIENTED_EDGE('',*,*,#3438,.T.);
#4461=ORIENTED_EDGE('',*,*,#3434,.F.);
#4462=ORIENTED_EDGE('',*,*,#3439,.T.);
#4463=ORIENTED_EDGE('',*,*,#3440,.T.);
#4464=ORIENTED_EDGE('',*,*,#3441,.T.);
#4465=ORIENTED_EDGE('',*,*,#3437,.F.);
#4466=ORIENTED_EDGE('',*,*,#3442,.T.);
#4467=ORIENTED_EDGE('',*,*,#3443,.T.);
#4468=ORIENTED_EDGE('',*,*,#3444,.T.);
#4469=ORIENTED_EDGE('',*,*,#3440,.F.);
#4470=ORIENTED_EDGE('',*,*,#3445,.T.);
#4471=ORIENTED_EDGE('',*,*,#3446,.F.);
#4472=ORIENTED_EDGE('',*,*,#3447,.T.);
#4473=ORIENTED_EDGE('',*,*,#3448,.F.);
#4474=ORIENTED_EDGE('',*,*,#3449,.T.);
#4475=ORIENTED_EDGE('',*,*,#3450,.T.);
#4476=ORIENTED_EDGE('',*,*,#3451,.T.);
#4477=ORIENTED_EDGE('',*,*,#3452,.F.);
#4478=ORIENTED_EDGE('',*,*,#3453,.F.);
#4479=ORIENTED_EDGE('',*,*,#3454,.T.);
#4480=ORIENTED_EDGE('',*,*,#3455,.T.);
#4481=ORIENTED_EDGE('',*,*,#3450,.F.);
#4482=ORIENTED_EDGE('',*,*,#3456,.F.);
#4483=ORIENTED_EDGE('',*,*,#3457,.T.);
#4484=ORIENTED_EDGE('',*,*,#3458,.T.);
#4485=ORIENTED_EDGE('',*,*,#3454,.F.);
#4486=ORIENTED_EDGE('',*,*,#3459,.F.);
#4487=ORIENTED_EDGE('',*,*,#3460,.T.);
#4488=ORIENTED_EDGE('',*,*,#3461,.T.);
#4489=ORIENTED_EDGE('',*,*,#3457,.F.);
#4490=ORIENTED_EDGE('',*,*,#3462,.F.);
#4491=ORIENTED_EDGE('',*,*,#3463,.T.);
#4492=ORIENTED_EDGE('',*,*,#3464,.T.);
#4493=ORIENTED_EDGE('',*,*,#3460,.F.);
#4494=ORIENTED_EDGE('',*,*,#3465,.F.);
#4495=ORIENTED_EDGE('',*,*,#3466,.T.);
#4496=ORIENTED_EDGE('',*,*,#3467,.T.);
#4497=ORIENTED_EDGE('',*,*,#3463,.F.);
#4498=ORIENTED_EDGE('',*,*,#3468,.F.);
#4499=ORIENTED_EDGE('',*,*,#3469,.T.);
#4500=ORIENTED_EDGE('',*,*,#3470,.T.);
#4501=ORIENTED_EDGE('',*,*,#3466,.F.);
#4502=ORIENTED_EDGE('',*,*,#3471,.F.);
#4503=ORIENTED_EDGE('',*,*,#3472,.T.);
#4504=ORIENTED_EDGE('',*,*,#3473,.T.);
#4505=ORIENTED_EDGE('',*,*,#3469,.F.);
#4506=ORIENTED_EDGE('',*,*,#3474,.F.);
#4507=ORIENTED_EDGE('',*,*,#3475,.T.);
#4508=ORIENTED_EDGE('',*,*,#3476,.T.);
#4509=ORIENTED_EDGE('',*,*,#3472,.F.);
#4510=ORIENTED_EDGE('',*,*,#3477,.F.);
#4511=ORIENTED_EDGE('',*,*,#3478,.T.);
#4512=ORIENTED_EDGE('',*,*,#3479,.T.);
#4513=ORIENTED_EDGE('',*,*,#3475,.F.);
#4514=ORIENTED_EDGE('',*,*,#3480,.F.);
#4515=ORIENTED_EDGE('',*,*,#3481,.T.);
#4516=ORIENTED_EDGE('',*,*,#3482,.T.);
#4517=ORIENTED_EDGE('',*,*,#3478,.F.);
#4518=ORIENTED_EDGE('',*,*,#3483,.F.);
#4519=ORIENTED_EDGE('',*,*,#3484,.T.);
#4520=ORIENTED_EDGE('',*,*,#3485,.T.);
#4521=ORIENTED_EDGE('',*,*,#3481,.F.);
#4522=ORIENTED_EDGE('',*,*,#3486,.F.);
#4523=ORIENTED_EDGE('',*,*,#3487,.T.);
#4524=ORIENTED_EDGE('',*,*,#3488,.T.);
#4525=ORIENTED_EDGE('',*,*,#3484,.F.);
#4526=ORIENTED_EDGE('',*,*,#3489,.F.);
#4527=ORIENTED_EDGE('',*,*,#3490,.T.);
#4528=ORIENTED_EDGE('',*,*,#3491,.T.);
#4529=ORIENTED_EDGE('',*,*,#3487,.F.);
#4530=ORIENTED_EDGE('',*,*,#3492,.F.);
#4531=ORIENTED_EDGE('',*,*,#3493,.T.);
#4532=ORIENTED_EDGE('',*,*,#3494,.T.);
#4533=ORIENTED_EDGE('',*,*,#3490,.F.);
#4534=ORIENTED_EDGE('',*,*,#3495,.F.);
#4535=ORIENTED_EDGE('',*,*,#3496,.F.);
#4536=ORIENTED_EDGE('',*,*,#3497,.F.);
#4537=ORIENTED_EDGE('',*,*,#3498,.F.);
#4538=ORIENTED_EDGE('',*,*,#3499,.T.);
#4539=ORIENTED_EDGE('',*,*,#3402,.F.);
#4540=ORIENTED_EDGE('',*,*,#3500,.T.);
#4541=ORIENTED_EDGE('',*,*,#3452,.T.);
#4542=ORIENTED_EDGE('',*,*,#3501,.T.);
#4543=ORIENTED_EDGE('',*,*,#3496,.T.);
#4544=ORIENTED_EDGE('',*,*,#3502,.T.);
#4545=ORIENTED_EDGE('',*,*,#3493,.F.);
#4546=ORIENTED_EDGE('',*,*,#3503,.F.);
#4547=ORIENTED_EDGE('',*,*,#3501,.F.);
#4548=ORIENTED_EDGE('',*,*,#3451,.F.);
#4549=ORIENTED_EDGE('',*,*,#3455,.F.);
#4550=ORIENTED_EDGE('',*,*,#3458,.F.);
#4551=ORIENTED_EDGE('',*,*,#3461,.F.);
#4552=ORIENTED_EDGE('',*,*,#3464,.F.);
#4553=ORIENTED_EDGE('',*,*,#3467,.F.);
#4554=ORIENTED_EDGE('',*,*,#3470,.F.);
#4555=ORIENTED_EDGE('',*,*,#3473,.F.);
#4556=ORIENTED_EDGE('',*,*,#3476,.F.);
#4557=ORIENTED_EDGE('',*,*,#3479,.F.);
#4558=ORIENTED_EDGE('',*,*,#3482,.F.);
#4559=ORIENTED_EDGE('',*,*,#3485,.F.);
#4560=ORIENTED_EDGE('',*,*,#3488,.F.);
#4561=ORIENTED_EDGE('',*,*,#3491,.F.);
#4562=ORIENTED_EDGE('',*,*,#3494,.F.);
#4563=ORIENTED_EDGE('',*,*,#3502,.F.);
#4564=ORIENTED_EDGE('',*,*,#3499,.F.);
#4565=ORIENTED_EDGE('',*,*,#3504,.F.);
#4566=ORIENTED_EDGE('',*,*,#3447,.F.);
#4567=ORIENTED_EDGE('',*,*,#3505,.F.);
#4568=ORIENTED_EDGE('',*,*,#3445,.F.);
#4569=ORIENTED_EDGE('',*,*,#3442,.F.);
#4570=ORIENTED_EDGE('',*,*,#3439,.F.);
#4571=ORIENTED_EDGE('',*,*,#3436,.F.);
#4572=ORIENTED_EDGE('',*,*,#3433,.F.);
#4573=ORIENTED_EDGE('',*,*,#3430,.F.);
#4574=ORIENTED_EDGE('',*,*,#3427,.F.);
#4575=ORIENTED_EDGE('',*,*,#3424,.F.);
#4576=ORIENTED_EDGE('',*,*,#3421,.F.);
#4577=ORIENTED_EDGE('',*,*,#3418,.F.);
#4578=ORIENTED_EDGE('',*,*,#3415,.F.);
#4579=ORIENTED_EDGE('',*,*,#3412,.F.);
#4580=ORIENTED_EDGE('',*,*,#3409,.F.);
#4581=ORIENTED_EDGE('',*,*,#3406,.F.);
#4582=ORIENTED_EDGE('',*,*,#3403,.F.);
#4583=ORIENTED_EDGE('',*,*,#3500,.F.);
#4584=ORIENTED_EDGE('',*,*,#3401,.F.);
#4585=ORIENTED_EDGE('',*,*,#3408,.F.);
#4586=ORIENTED_EDGE('',*,*,#3411,.F.);
#4587=ORIENTED_EDGE('',*,*,#3414,.F.);
#4588=ORIENTED_EDGE('',*,*,#3417,.F.);
#4589=ORIENTED_EDGE('',*,*,#3420,.F.);
#4590=ORIENTED_EDGE('',*,*,#3423,.F.);
#4591=ORIENTED_EDGE('',*,*,#3426,.F.);
#4592=ORIENTED_EDGE('',*,*,#3429,.F.);
#4593=ORIENTED_EDGE('',*,*,#3432,.F.);
#4594=ORIENTED_EDGE('',*,*,#3435,.F.);
#4595=ORIENTED_EDGE('',*,*,#3438,.F.);
#4596=ORIENTED_EDGE('',*,*,#3441,.F.);
#4597=ORIENTED_EDGE('',*,*,#3444,.F.);
#4598=ORIENTED_EDGE('',*,*,#3506,.F.);
#4599=ORIENTED_EDGE('',*,*,#3449,.F.);
#4600=ORIENTED_EDGE('',*,*,#3507,.F.);
#4601=ORIENTED_EDGE('',*,*,#3497,.T.);
#4602=ORIENTED_EDGE('',*,*,#3503,.T.);
#4603=ORIENTED_EDGE('',*,*,#3495,.T.);
#4604=ORIENTED_EDGE('',*,*,#3492,.T.);
#4605=ORIENTED_EDGE('',*,*,#3489,.T.);
#4606=ORIENTED_EDGE('',*,*,#3486,.T.);
#4607=ORIENTED_EDGE('',*,*,#3483,.T.);
#4608=ORIENTED_EDGE('',*,*,#3480,.T.);
#4609=ORIENTED_EDGE('',*,*,#3477,.T.);
#4610=ORIENTED_EDGE('',*,*,#3474,.T.);
#4611=ORIENTED_EDGE('',*,*,#3471,.T.);
#4612=ORIENTED_EDGE('',*,*,#3468,.T.);
#4613=ORIENTED_EDGE('',*,*,#3465,.T.);
#4614=ORIENTED_EDGE('',*,*,#3462,.T.);
#4615=ORIENTED_EDGE('',*,*,#3459,.T.);
#4616=ORIENTED_EDGE('',*,*,#3456,.T.);
#4617=ORIENTED_EDGE('',*,*,#3453,.T.);
#4618=ORIENTED_EDGE('',*,*,#3446,.T.);
#4619=ORIENTED_EDGE('',*,*,#3506,.T.);
#4620=ORIENTED_EDGE('',*,*,#3443,.F.);
#4621=ORIENTED_EDGE('',*,*,#3505,.T.);
#4622=ORIENTED_EDGE('',*,*,#3302,.F.);
#4623=ORIENTED_EDGE('',*,*,#3508,.T.);
#4624=ORIENTED_EDGE('',*,*,#3352,.T.);
#4625=ORIENTED_EDGE('',*,*,#3509,.T.);
#4626=ORIENTED_EDGE('',*,*,#3396,.T.);
#4627=ORIENTED_EDGE('',*,*,#3510,.T.);
#4628=ORIENTED_EDGE('',*,*,#3393,.F.);
#4629=ORIENTED_EDGE('',*,*,#3511,.F.);
#4630=ORIENTED_EDGE('',*,*,#3509,.F.);
#4631=ORIENTED_EDGE('',*,*,#3351,.F.);
#4632=ORIENTED_EDGE('',*,*,#3355,.F.);
#4633=ORIENTED_EDGE('',*,*,#3358,.F.);
#4634=ORIENTED_EDGE('',*,*,#3361,.F.);
#4635=ORIENTED_EDGE('',*,*,#3364,.F.);
#4636=ORIENTED_EDGE('',*,*,#3367,.F.);
#4637=ORIENTED_EDGE('',*,*,#3370,.F.);
#4638=ORIENTED_EDGE('',*,*,#3373,.F.);
#4639=ORIENTED_EDGE('',*,*,#3376,.F.);
#4640=ORIENTED_EDGE('',*,*,#3379,.F.);
#4641=ORIENTED_EDGE('',*,*,#3382,.F.);
#4642=ORIENTED_EDGE('',*,*,#3385,.F.);
#4643=ORIENTED_EDGE('',*,*,#3388,.F.);
#4644=ORIENTED_EDGE('',*,*,#3391,.F.);
#4645=ORIENTED_EDGE('',*,*,#3394,.F.);
#4646=ORIENTED_EDGE('',*,*,#3510,.F.);
#4647=ORIENTED_EDGE('',*,*,#3399,.F.);
#4648=ORIENTED_EDGE('',*,*,#3512,.F.);
#4649=ORIENTED_EDGE('',*,*,#3347,.F.);
#4650=ORIENTED_EDGE('',*,*,#3513,.F.);
#4651=ORIENTED_EDGE('',*,*,#3345,.F.);
#4652=ORIENTED_EDGE('',*,*,#3342,.F.);
#4653=ORIENTED_EDGE('',*,*,#3339,.F.);
#4654=ORIENTED_EDGE('',*,*,#3336,.F.);
#4655=ORIENTED_EDGE('',*,*,#3333,.F.);
#4656=ORIENTED_EDGE('',*,*,#3330,.F.);
#4657=ORIENTED_EDGE('',*,*,#3327,.F.);
#4658=ORIENTED_EDGE('',*,*,#3324,.F.);
#4659=ORIENTED_EDGE('',*,*,#3321,.F.);
#4660=ORIENTED_EDGE('',*,*,#3318,.F.);
#4661=ORIENTED_EDGE('',*,*,#3315,.F.);
#4662=ORIENTED_EDGE('',*,*,#3312,.F.);
#4663=ORIENTED_EDGE('',*,*,#3309,.F.);
#4664=ORIENTED_EDGE('',*,*,#3306,.F.);
#4665=ORIENTED_EDGE('',*,*,#3303,.F.);
#4666=ORIENTED_EDGE('',*,*,#3508,.F.);
#4667=ORIENTED_EDGE('',*,*,#3301,.F.);
#4668=ORIENTED_EDGE('',*,*,#3308,.F.);
#4669=ORIENTED_EDGE('',*,*,#3311,.F.);
#4670=ORIENTED_EDGE('',*,*,#3314,.F.);
#4671=ORIENTED_EDGE('',*,*,#3317,.F.);
#4672=ORIENTED_EDGE('',*,*,#3320,.F.);
#4673=ORIENTED_EDGE('',*,*,#3323,.F.);
#4674=ORIENTED_EDGE('',*,*,#3326,.F.);
#4675=ORIENTED_EDGE('',*,*,#3329,.F.);
#4676=ORIENTED_EDGE('',*,*,#3332,.F.);
#4677=ORIENTED_EDGE('',*,*,#3335,.F.);
#4678=ORIENTED_EDGE('',*,*,#3338,.F.);
#4679=ORIENTED_EDGE('',*,*,#3341,.F.);
#4680=ORIENTED_EDGE('',*,*,#3344,.F.);
#4681=ORIENTED_EDGE('',*,*,#3514,.F.);
#4682=ORIENTED_EDGE('',*,*,#3349,.F.);
#4683=ORIENTED_EDGE('',*,*,#3515,.F.);
#4684=ORIENTED_EDGE('',*,*,#3397,.T.);
#4685=ORIENTED_EDGE('',*,*,#3511,.T.);
#4686=ORIENTED_EDGE('',*,*,#3395,.T.);
#4687=ORIENTED_EDGE('',*,*,#3392,.T.);
#4688=ORIENTED_EDGE('',*,*,#3389,.T.);
#4689=ORIENTED_EDGE('',*,*,#3386,.T.);
#4690=ORIENTED_EDGE('',*,*,#3383,.T.);
#4691=ORIENTED_EDGE('',*,*,#3380,.T.);
#4692=ORIENTED_EDGE('',*,*,#3377,.T.);
#4693=ORIENTED_EDGE('',*,*,#3374,.T.);
#4694=ORIENTED_EDGE('',*,*,#3371,.T.);
#4695=ORIENTED_EDGE('',*,*,#3368,.T.);
#4696=ORIENTED_EDGE('',*,*,#3365,.T.);
#4697=ORIENTED_EDGE('',*,*,#3362,.T.);
#4698=ORIENTED_EDGE('',*,*,#3359,.T.);
#4699=ORIENTED_EDGE('',*,*,#3356,.T.);
#4700=ORIENTED_EDGE('',*,*,#3353,.T.);
#4701=ORIENTED_EDGE('',*,*,#3346,.T.);
#4702=ORIENTED_EDGE('',*,*,#3514,.T.);
#4703=ORIENTED_EDGE('',*,*,#3343,.F.);
#4704=ORIENTED_EDGE('',*,*,#3513,.T.);
#4705=ORIENTED_EDGE('',*,*,#3405,.F.);
#4706=ORIENTED_EDGE('',*,*,#3305,.F.);
#4707=ORIENTED_EDGE('',*,*,#3516,.F.);
#4708=ORIENTED_EDGE('',*,*,#3517,.T.);
#4709=ORIENTED_EDGE('',*,*,#3518,.F.);
#4710=ORIENTED_EDGE('',*,*,#3517,.F.);
#4711=ORIENTED_EDGE('',*,*,#3519,.F.);
#4712=ORIENTED_EDGE('',*,*,#3520,.T.);
#4713=ORIENTED_EDGE('',*,*,#3521,.F.);
#4714=ORIENTED_EDGE('',*,*,#3520,.F.);
#4715=ORIENTED_EDGE('',*,*,#3522,.F.);
#4716=ORIENTED_EDGE('',*,*,#3523,.T.);
#4717=ORIENTED_EDGE('',*,*,#3524,.F.);
#4718=ORIENTED_EDGE('',*,*,#3523,.F.);
#4719=ORIENTED_EDGE('',*,*,#3525,.F.);
#4720=ORIENTED_EDGE('',*,*,#3526,.F.);
#4721=ORIENTED_EDGE('',*,*,#3527,.T.);
#4722=ORIENTED_EDGE('',*,*,#3528,.T.);
#4723=ORIENTED_EDGE('',*,*,#3529,.F.);
#4724=ORIENTED_EDGE('',*,*,#3530,.F.);
#4725=ORIENTED_EDGE('',*,*,#3531,.T.);
#4726=ORIENTED_EDGE('',*,*,#3532,.T.);
#4727=ORIENTED_EDGE('',*,*,#3527,.F.);
#4728=ORIENTED_EDGE('',*,*,#3533,.F.);
#4729=ORIENTED_EDGE('',*,*,#3531,.F.);
#4730=ORIENTED_EDGE('',*,*,#3534,.F.);
#4731=ORIENTED_EDGE('',*,*,#3525,.T.);
#4732=ORIENTED_EDGE('',*,*,#3535,.F.);
#4733=ORIENTED_EDGE('',*,*,#3536,.F.);
#4734=ORIENTED_EDGE('',*,*,#3537,.F.);
#4735=ORIENTED_EDGE('',*,*,#3529,.T.);
#4736=ORIENTED_EDGE('',*,*,#3538,.F.);
#4737=ORIENTED_EDGE('',*,*,#3539,.F.);
#4738=ORIENTED_EDGE('',*,*,#3540,.F.);
#4739=ORIENTED_EDGE('',*,*,#3541,.F.);
#4740=ORIENTED_EDGE('',*,*,#3542,.F.);
#4741=ORIENTED_EDGE('',*,*,#3543,.T.);
#4742=ORIENTED_EDGE('',*,*,#3544,.T.);
#4743=ORIENTED_EDGE('',*,*,#3524,.T.);
#4744=ORIENTED_EDGE('',*,*,#3545,.F.);
#4745=ORIENTED_EDGE('',*,*,#3546,.F.);
#4746=ORIENTED_EDGE('',*,*,#3547,.T.);
#4747=ORIENTED_EDGE('',*,*,#3542,.T.);
#4748=ORIENTED_EDGE('',*,*,#3548,.F.);
#4749=ORIENTED_EDGE('',*,*,#3544,.F.);
#4750=ORIENTED_EDGE('',*,*,#3549,.T.);
#4751=ORIENTED_EDGE('',*,*,#3550,.T.);
#4752=ORIENTED_EDGE('',*,*,#3547,.F.);
#4753=ORIENTED_EDGE('',*,*,#3551,.F.);
#4754=ORIENTED_EDGE('',*,*,#3549,.F.);
#4755=ORIENTED_EDGE('',*,*,#3543,.F.);
#4756=ORIENTED_EDGE('',*,*,#3545,.T.);
#4757=ORIENTED_EDGE('',*,*,#3541,.T.);
#4758=ORIENTED_EDGE('',*,*,#3548,.T.);
#4759=ORIENTED_EDGE('',*,*,#3552,.F.);
#4760=ORIENTED_EDGE('',*,*,#3553,.F.);
#4761=ORIENTED_EDGE('',*,*,#3554,.F.);
#4762=ORIENTED_EDGE('',*,*,#3555,.T.);
#4763=ORIENTED_EDGE('',*,*,#3556,.T.);
#4764=ORIENTED_EDGE('',*,*,#3557,.T.);
#4765=ORIENTED_EDGE('',*,*,#3558,.F.);
#4766=ORIENTED_EDGE('',*,*,#3559,.F.);
#4767=ORIENTED_EDGE('',*,*,#3560,.F.);
#4768=ORIENTED_EDGE('',*,*,#3561,.T.);
#4769=ORIENTED_EDGE('',*,*,#3562,.T.);
#4770=ORIENTED_EDGE('',*,*,#3563,.T.);
#4771=ORIENTED_EDGE('',*,*,#3564,.T.);
#4772=ORIENTED_EDGE('',*,*,#3565,.T.);
#4773=ORIENTED_EDGE('',*,*,#3566,.T.);
#4774=ORIENTED_EDGE('',*,*,#3567,.T.);
#4775=ORIENTED_EDGE('',*,*,#3568,.T.);
#4776=ORIENTED_EDGE('',*,*,#3537,.T.);
#4777=ORIENTED_EDGE('',*,*,#3569,.T.);
#4778=ORIENTED_EDGE('',*,*,#3556,.F.);
#4779=ORIENTED_EDGE('',*,*,#3570,.F.);
#4780=ORIENTED_EDGE('',*,*,#3538,.T.);
#4781=ORIENTED_EDGE('',*,*,#3532,.F.);
#4782=ORIENTED_EDGE('',*,*,#3533,.T.);
#4783=ORIENTED_EDGE('',*,*,#3526,.T.);
#4784=ORIENTED_EDGE('',*,*,#3516,.T.);
#4785=ORIENTED_EDGE('',*,*,#3519,.T.);
#4786=ORIENTED_EDGE('',*,*,#3555,.F.);
#4787=ORIENTED_EDGE('',*,*,#3571,.F.);
#4788=ORIENTED_EDGE('',*,*,#3539,.T.);
#4789=ORIENTED_EDGE('',*,*,#3570,.T.);
#4790=ORIENTED_EDGE('',*,*,#3557,.F.);
#4791=ORIENTED_EDGE('',*,*,#3569,.F.);
#4792=ORIENTED_EDGE('',*,*,#3536,.T.);
#4793=ORIENTED_EDGE('',*,*,#3572,.T.);
#4794=ORIENTED_EDGE('',*,*,#3540,.T.);
#4795=ORIENTED_EDGE('',*,*,#3571,.T.);
#4796=ORIENTED_EDGE('',*,*,#3554,.T.);
#4797=ORIENTED_EDGE('',*,*,#3573,.T.);
#4798=ORIENTED_EDGE('',*,*,#3574,.F.);
#4799=ORIENTED_EDGE('',*,*,#3575,.T.);
#4800=ORIENTED_EDGE('',*,*,#3576,.T.);
#4801=ORIENTED_EDGE('',*,*,#3577,.T.);
#4802=ORIENTED_EDGE('',*,*,#3578,.F.);
#4803=ORIENTED_EDGE('',*,*,#3579,.F.);
#4804=ORIENTED_EDGE('',*,*,#3558,.T.);
#4805=ORIENTED_EDGE('',*,*,#3572,.F.);
#4806=ORIENTED_EDGE('',*,*,#3535,.T.);
#4807=ORIENTED_EDGE('',*,*,#3528,.F.);
#4808=ORIENTED_EDGE('',*,*,#3534,.T.);
#4809=ORIENTED_EDGE('',*,*,#3530,.T.);
#4810=ORIENTED_EDGE('',*,*,#3518,.T.);
#4811=ORIENTED_EDGE('',*,*,#3521,.T.);
#4812=ORIENTED_EDGE('',*,*,#3580,.F.);
#4813=ORIENTED_EDGE('',*,*,#3581,.T.);
#4814=ORIENTED_EDGE('',*,*,#3565,.F.);
#4815=ORIENTED_EDGE('',*,*,#3582,.F.);
#4816=ORIENTED_EDGE('',*,*,#3583,.F.);
#4817=ORIENTED_EDGE('',*,*,#3584,.T.);
#4818=ORIENTED_EDGE('',*,*,#3566,.F.);
#4819=ORIENTED_EDGE('',*,*,#3581,.F.);
#4820=ORIENTED_EDGE('',*,*,#3585,.F.);
#4821=ORIENTED_EDGE('',*,*,#3586,.T.);
#4822=ORIENTED_EDGE('',*,*,#3567,.F.);
#4823=ORIENTED_EDGE('',*,*,#3584,.F.);
#4824=ORIENTED_EDGE('',*,*,#3587,.F.);
#4825=ORIENTED_EDGE('',*,*,#3582,.T.);
#4826=ORIENTED_EDGE('',*,*,#3568,.F.);
#4827=ORIENTED_EDGE('',*,*,#3586,.F.);
#4828=ORIENTED_EDGE('',*,*,#3588,.F.);
#4829=ORIENTED_EDGE('',*,*,#3589,.T.);
#4830=ORIENTED_EDGE('',*,*,#3561,.F.);
#4831=ORIENTED_EDGE('',*,*,#3590,.F.);
#4832=ORIENTED_EDGE('',*,*,#3591,.F.);
#4833=ORIENTED_EDGE('',*,*,#3592,.T.);
#4834=ORIENTED_EDGE('',*,*,#3562,.F.);
#4835=ORIENTED_EDGE('',*,*,#3589,.F.);
#4836=ORIENTED_EDGE('',*,*,#3593,.F.);
#4837=ORIENTED_EDGE('',*,*,#3594,.T.);
#4838=ORIENTED_EDGE('',*,*,#3563,.F.);
#4839=ORIENTED_EDGE('',*,*,#3592,.F.);
#4840=ORIENTED_EDGE('',*,*,#3595,.F.);
#4841=ORIENTED_EDGE('',*,*,#3590,.T.);
#4842=ORIENTED_EDGE('',*,*,#3564,.F.);
#4843=ORIENTED_EDGE('',*,*,#3594,.F.);
#4844=ORIENTED_EDGE('',*,*,#3596,.F.);
#4845=ORIENTED_EDGE('',*,*,#3597,.F.);
#4846=ORIENTED_EDGE('',*,*,#3577,.F.);
#4847=ORIENTED_EDGE('',*,*,#3598,.T.);
#4848=ORIENTED_EDGE('',*,*,#3599,.T.);
#4849=ORIENTED_EDGE('',*,*,#3600,.F.);
#4850=ORIENTED_EDGE('',*,*,#3601,.F.);
#4851=ORIENTED_EDGE('',*,*,#3602,.T.);
#4852=ORIENTED_EDGE('',*,*,#3576,.F.);
#4853=ORIENTED_EDGE('',*,*,#3603,.F.);
#4854=ORIENTED_EDGE('',*,*,#3604,.F.);
#4855=ORIENTED_EDGE('',*,*,#3598,.F.);
#4856=ORIENTED_EDGE('',*,*,#3605,.F.);
#4857=ORIENTED_EDGE('',*,*,#3602,.F.);
#4858=ORIENTED_EDGE('',*,*,#3606,.F.);
#4859=ORIENTED_EDGE('',*,*,#3607,.F.);
#4860=ORIENTED_EDGE('',*,*,#3606,.T.);
#4861=ORIENTED_EDGE('',*,*,#3601,.T.);
#4862=ORIENTED_EDGE('',*,*,#3608,.F.);
#4863=ORIENTED_EDGE('',*,*,#3609,.F.);
#4864=ORIENTED_EDGE('',*,*,#3610,.F.);
#4865=ORIENTED_EDGE('',*,*,#3607,.T.);
#4866=ORIENTED_EDGE('',*,*,#3609,.T.);
#4867=ORIENTED_EDGE('',*,*,#3611,.F.);
#4868=ORIENTED_EDGE('',*,*,#3612,.F.);
#4869=ORIENTED_EDGE('',*,*,#3603,.T.);
#4870=ORIENTED_EDGE('',*,*,#3575,.F.);
#4871=ORIENTED_EDGE('',*,*,#3613,.F.);
#4872=ORIENTED_EDGE('',*,*,#3604,.T.);
#4873=ORIENTED_EDGE('',*,*,#3612,.T.);
#4874=ORIENTED_EDGE('',*,*,#3614,.F.);
#4875=ORIENTED_EDGE('',*,*,#3599,.F.);
#4876=ORIENTED_EDGE('',*,*,#3600,.T.);
#4877=ORIENTED_EDGE('',*,*,#3614,.T.);
#4878=ORIENTED_EDGE('',*,*,#3611,.T.);
#4879=ORIENTED_EDGE('',*,*,#3608,.T.);
#4880=ORIENTED_EDGE('',*,*,#3507,.T.);
#4881=ORIENTED_EDGE('',*,*,#3448,.T.);
#4882=ORIENTED_EDGE('',*,*,#3504,.T.);
#4883=ORIENTED_EDGE('',*,*,#3498,.T.);
#4884=ORIENTED_EDGE('',*,*,#3515,.T.);
#4885=ORIENTED_EDGE('',*,*,#3348,.T.);
#4886=ORIENTED_EDGE('',*,*,#3512,.T.);
#4887=ORIENTED_EDGE('',*,*,#3398,.T.);
#4888=ORIENTED_EDGE('',*,*,#3597,.T.);
#4889=ORIENTED_EDGE('',*,*,#3615,.T.);
#4890=ORIENTED_EDGE('',*,*,#3616,.T.);
#4891=ORIENTED_EDGE('',*,*,#3578,.T.);
#4892=ORIENTED_EDGE('',*,*,#3580,.T.);
#4893=ORIENTED_EDGE('',*,*,#3587,.T.);
#4894=ORIENTED_EDGE('',*,*,#3585,.T.);
#4895=ORIENTED_EDGE('',*,*,#3583,.T.);
#4896=ORIENTED_EDGE('',*,*,#3613,.T.);
#4897=ORIENTED_EDGE('',*,*,#3574,.T.);
#4898=ORIENTED_EDGE('',*,*,#3617,.T.);
#4899=ORIENTED_EDGE('',*,*,#3618,.T.);
#4900=ORIENTED_EDGE('',*,*,#3588,.T.);
#4901=ORIENTED_EDGE('',*,*,#3595,.T.);
#4902=ORIENTED_EDGE('',*,*,#3593,.T.);
#4903=ORIENTED_EDGE('',*,*,#3591,.T.);
#4904=ORIENTED_EDGE('',*,*,#3560,.T.);
#4905=ORIENTED_EDGE('',*,*,#3619,.T.);
#4906=ORIENTED_EDGE('',*,*,#3615,.F.);
#4907=ORIENTED_EDGE('',*,*,#3596,.T.);
#4908=ORIENTED_EDGE('',*,*,#3605,.T.);
#4909=ORIENTED_EDGE('',*,*,#3610,.T.);
#4910=ORIENTED_EDGE('',*,*,#3618,.F.);
#4911=ORIENTED_EDGE('',*,*,#3620,.F.);
#4912=ORIENTED_EDGE('',*,*,#3552,.T.);
#4913=ORIENTED_EDGE('',*,*,#3550,.F.);
#4914=ORIENTED_EDGE('',*,*,#3551,.T.);
#4915=ORIENTED_EDGE('',*,*,#3546,.T.);
#4916=ORIENTED_EDGE('',*,*,#3522,.T.);
#4917=ORIENTED_EDGE('',*,*,#3553,.T.);
#4918=ORIENTED_EDGE('',*,*,#3620,.T.);
#4919=ORIENTED_EDGE('',*,*,#3617,.F.);
#4920=ORIENTED_EDGE('',*,*,#3573,.F.);
#4921=ORIENTED_EDGE('',*,*,#3559,.T.);
#4922=ORIENTED_EDGE('',*,*,#3579,.T.);
#4923=ORIENTED_EDGE('',*,*,#3616,.F.);
#4924=ORIENTED_EDGE('',*,*,#3619,.F.);
#5937=PLANE('',#6776);
#5938=PLANE('',#6779);
#5939=PLANE('',#6782);
#5940=PLANE('',#6783);
#5941=PLANE('',#6793);
#5942=PLANE('',#6794);
#5943=PLANE('',#6795);
#5944=PLANE('',#6796);
#5945=PLANE('',#6797);
#5946=PLANE('',#6798);
#5947=PLANE('',#6799);
#5948=PLANE('',#6800);
#5949=PLANE('',#6801);
#5950=PLANE('',#6802);
#5951=PLANE('',#6803);
#5952=PLANE('',#6804);
#5953=PLANE('',#6805);
#5954=PLANE('',#6806);
#5955=PLANE('',#6807);
#5956=PLANE('',#6808);
#5957=PLANE('',#6809);
#5958=PLANE('',#6810);
#5959=PLANE('',#6811);
#5960=PLANE('',#6812);
#5961=PLANE('',#6813);
#5962=PLANE('',#6814);
#5963=PLANE('',#6815);
#5964=PLANE('',#6816);
#5965=PLANE('',#6817);
#5966=PLANE('',#6818);
#5967=PLANE('',#6819);
#5968=PLANE('',#6820);
#5969=PLANE('',#6821);
#5970=PLANE('',#6822);
#5971=PLANE('',#6823);
#5972=PLANE('',#6824);
#5973=PLANE('',#6825);
#5974=PLANE('',#6826);
#6098=ADVANCED_FACE('',(#1719),#1431,.F.);
#6099=ADVANCED_FACE('',(#1720),#1432,.F.);
#6100=ADVANCED_FACE('',(#1721),#1433,.F.);
#6101=ADVANCED_FACE('',(#1722),#1434,.F.);
#6102=ADVANCED_FACE('',(#1723),#1435,.F.);
#6103=ADVANCED_FACE('',(#1724),#1436,.F.);
#6104=ADVANCED_FACE('',(#1725),#1437,.F.);
#6105=ADVANCED_FACE('',(#1726),#1438,.F.);
#6106=ADVANCED_FACE('',(#1727),#1439,.F.);
#6107=ADVANCED_FACE('',(#1728),#1440,.F.);
#6108=ADVANCED_FACE('',(#1729),#1441,.F.);
#6109=ADVANCED_FACE('',(#1730),#1442,.F.);
#6110=ADVANCED_FACE('',(#1731),#1443,.F.);
#6111=ADVANCED_FACE('',(#1732),#1444,.F.);
#6112=ADVANCED_FACE('',(#1733),#1445,.F.);
#6113=ADVANCED_FACE('',(#1734),#1446,.F.);
#6114=ADVANCED_FACE('',(#1735),#1447,.F.);
#6115=ADVANCED_FACE('',(#1736),#1448,.F.);
#6116=ADVANCED_FACE('',(#1737),#1449,.F.);
#6117=ADVANCED_FACE('',(#1738),#1450,.F.);
#6118=ADVANCED_FACE('',(#1739),#1451,.F.);
#6119=ADVANCED_FACE('',(#1740),#1452,.F.);
#6120=ADVANCED_FACE('',(#1741),#1453,.F.);
#6121=ADVANCED_FACE('',(#1742),#1454,.F.);
#6122=ADVANCED_FACE('',(#1743),#1455,.F.);
#6123=ADVANCED_FACE('',(#1744),#1456,.F.);
#6124=ADVANCED_FACE('',(#1745),#1457,.F.);
#6125=ADVANCED_FACE('',(#1746),#1458,.F.);
#6126=ADVANCED_FACE('',(#1747),#1459,.F.);
#6127=ADVANCED_FACE('',(#1748),#1460,.F.);
#6128=ADVANCED_FACE('',(#1749),#1461,.F.);
#6129=ADVANCED_FACE('',(#1750),#1462,.F.);
#6130=ADVANCED_FACE('',(#1751),#1463,.F.);
#6131=ADVANCED_FACE('',(#1752),#1464,.F.);
#6132=ADVANCED_FACE('',(#1753),#1465,.F.);
#6133=ADVANCED_FACE('',(#1754),#1466,.F.);
#6134=ADVANCED_FACE('',(#1755),#1467,.F.);
#6135=ADVANCED_FACE('',(#1756),#1468,.F.);
#6136=ADVANCED_FACE('',(#1757),#1469,.F.);
#6137=ADVANCED_FACE('',(#1758),#1470,.F.);
#6138=ADVANCED_FACE('',(#1759),#1471,.F.);
#6139=ADVANCED_FACE('',(#1760),#1472,.F.);
#6140=ADVANCED_FACE('',(#1761),#1473,.F.);
#6141=ADVANCED_FACE('',(#1762),#1474,.F.);
#6142=ADVANCED_FACE('',(#1763),#1475,.F.);
#6143=ADVANCED_FACE('',(#1764),#1476,.F.);
#6144=ADVANCED_FACE('',(#1765),#1477,.F.);
#6145=ADVANCED_FACE('',(#1766),#1478,.F.);
#6146=ADVANCED_FACE('',(#1767),#1479,.F.);
#6147=ADVANCED_FACE('',(#1768),#1480,.F.);
#6148=ADVANCED_FACE('',(#1769),#1481,.F.);
#6149=ADVANCED_FACE('',(#1770),#1482,.F.);
#6150=ADVANCED_FACE('',(#1771),#1483,.F.);
#6151=ADVANCED_FACE('',(#1772),#1484,.F.);
#6152=ADVANCED_FACE('',(#1773),#1485,.F.);
#6153=ADVANCED_FACE('',(#1774),#1486,.F.);
#6154=ADVANCED_FACE('',(#1775),#1487,.F.);
#6155=ADVANCED_FACE('',(#1776),#1488,.F.);
#6156=ADVANCED_FACE('',(#1777),#1489,.F.);
#6157=ADVANCED_FACE('',(#1778),#1490,.F.);
#6158=ADVANCED_FACE('',(#1779),#1491,.F.);
#6159=ADVANCED_FACE('',(#1780),#1492,.F.);
#6160=ADVANCED_FACE('',(#1781),#5937,.T.);
#6161=ADVANCED_FACE('',(#1782),#1493,.F.);
#6162=ADVANCED_FACE('',(#1783),#117,.F.);
#6163=ADVANCED_FACE('',(#1784),#118,.F.);
#6164=ADVANCED_FACE('',(#1785),#1494,.F.);
#6165=ADVANCED_FACE('',(#1786),#5938,.T.);
#6166=ADVANCED_FACE('',(#1787),#1495,.F.);
#6167=ADVANCED_FACE('',(#1788),#119,.F.);
#6168=ADVANCED_FACE('',(#1789),#120,.F.);
#6169=ADVANCED_FACE('',(#1790),#1496,.F.);
#6170=ADVANCED_FACE('',(#1791),#5939,.F.);
#6171=ADVANCED_FACE('',(#1792),#5940,.F.);
#6172=ADVANCED_FACE('',(#1793),#1497,.F.);
#6173=ADVANCED_FACE('',(#1794),#1498,.F.);
#6174=ADVANCED_FACE('',(#1795),#1499,.F.);
#6175=ADVANCED_FACE('',(#1796),#5941,.T.);
#6176=ADVANCED_FACE('',(#1797),#5942,.T.);
#6177=ADVANCED_FACE('',(#1798),#5943,.F.);
#6178=ADVANCED_FACE('',(#1799),#5944,.F.);
#6179=ADVANCED_FACE('',(#1800),#5945,.F.);
#6180=ADVANCED_FACE('',(#1801,#1634),#5946,.T.);
#6181=ADVANCED_FACE('',(#1802),#5947,.T.);
#6182=ADVANCED_FACE('',(#1803),#5948,.T.);
#6183=ADVANCED_FACE('',(#1804),#5949,.F.);
#6184=ADVANCED_FACE('',(#1805,#1635,#1636),#5950,.F.);
#6185=ADVANCED_FACE('',(#1806,#1637,#1638),#5951,.T.);
#6186=ADVANCED_FACE('',(#1807),#5952,.T.);
#6187=ADVANCED_FACE('',(#1808),#5953,.T.);
#6188=ADVANCED_FACE('',(#1809,#1639,#1640),#5954,.T.);
#6189=ADVANCED_FACE('',(#1810),#5955,.F.);
#6190=ADVANCED_FACE('',(#1811),#5956,.F.);
#6191=ADVANCED_FACE('',(#1812),#5957,.F.);
#6192=ADVANCED_FACE('',(#1813),#5958,.F.);
#6193=ADVANCED_FACE('',(#1814),#5959,.F.);
#6194=ADVANCED_FACE('',(#1815),#5960,.F.);
#6195=ADVANCED_FACE('',(#1816),#5961,.F.);
#6196=ADVANCED_FACE('',(#1817),#5962,.F.);
#6197=ADVANCED_FACE('',(#1818),#5963,.T.);
#6198=ADVANCED_FACE('',(#1819),#5964,.F.);
#6199=ADVANCED_FACE('',(#1820),#5965,.F.);
#6200=ADVANCED_FACE('',(#1821),#5966,.T.);
#6201=ADVANCED_FACE('',(#1822),#5967,.T.);
#6202=ADVANCED_FACE('',(#1823),#5968,.T.);
#6203=ADVANCED_FACE('',(#1824,#1641,#1642),#5969,.T.);
#6204=ADVANCED_FACE('',(#1825,#1643),#5970,.T.);
#6205=ADVANCED_FACE('',(#1826,#1644),#5971,.T.);
#6206=ADVANCED_FACE('',(#1827,#1645),#5972,.T.);
#6207=ADVANCED_FACE('',(#1828),#5973,.T.);
#6208=ADVANCED_FACE('',(#1829),#5974,.T.);
#6425=CLOSED_SHELL('',(#6098,#6099,#6100,#6101,#6102,#6103,#6104,#6105,
#6106,#6107,#6108,#6109,#6110,#6111,#6112,#6113,#6114,#6115,#6116,#6117,
#6118,#6119,#6120,#6121,#6122,#6123,#6124,#6125,#6126,#6127,#6128,#6129,
#6130,#6131,#6132,#6133,#6134,#6135,#6136,#6137,#6138,#6139,#6140,#6141,
#6142,#6143,#6144,#6145,#6146,#6147,#6148,#6149,#6150,#6151,#6152,#6153,
#6154,#6155,#6156,#6157,#6158,#6159,#6160,#6161,#6162,#6163,#6164,#6165,
#6166,#6167,#6168,#6169,#6170,#6171,#6172,#6173,#6174,#6175,#6176,#6177,
#6178,#6179,#6180,#6181,#6182,#6183,#6184,#6185,#6186,#6187,#6188,#6189,
#6190,#6191,#6192,#6193,#6194,#6195,#6196,#6197,#6198,#6199,#6200,#6201,
#6202,#6203,#6204,#6205,#6206,#6207,#6208));
#6703=AXIS2_PLACEMENT_3D('',#8906,#7359,#7360);
#6704=AXIS2_PLACEMENT_3D('',#8907,#7361,#7362);
#6705=AXIS2_PLACEMENT_3D('',#8932,#7364,#7365);
#6706=AXIS2_PLACEMENT_3D('',#8940,#7367,#7368);
#6707=AXIS2_PLACEMENT_3D('',#8963,#7369,#7370);
#6708=AXIS2_PLACEMENT_3D('',#9014,#7372,#7373);
#6709=AXIS2_PLACEMENT_3D('',#9062,#7375,#7376);
#6710=AXIS2_PLACEMENT_3D('',#9113,#7378,#7379);
#6711=AXIS2_PLACEMENT_3D('',#9164,#7381,#7382);
#6712=AXIS2_PLACEMENT_3D('',#9212,#7384,#7385);
#6713=AXIS2_PLACEMENT_3D('',#9260,#7387,#7388);
#6714=AXIS2_PLACEMENT_3D('',#9311,#7390,#7391);
#6715=AXIS2_PLACEMENT_3D('',#9359,#7393,#7394);
#6716=AXIS2_PLACEMENT_3D('',#9407,#7396,#7397);
#6717=AXIS2_PLACEMENT_3D('',#9458,#7399,#7400);
#6718=AXIS2_PLACEMENT_3D('',#9509,#7402,#7403);
#6719=AXIS2_PLACEMENT_3D('',#9557,#7405,#7406);
#6720=AXIS2_PLACEMENT_3D('',#9608,#7408,#7409);
#6721=AXIS2_PLACEMENT_3D('',#9627,#7411,#7412);
#6722=AXIS2_PLACEMENT_3D('',#9647,#7413,#7414);
#6723=AXIS2_PLACEMENT_3D('',#9659,#7416,#7417);
#6724=AXIS2_PLACEMENT_3D('',#9667,#7418,#7419);
#6725=AXIS2_PLACEMENT_3D('',#9691,#7421,#7422);
#6726=AXIS2_PLACEMENT_3D('',#9716,#7424,#7425);
#6727=AXIS2_PLACEMENT_3D('',#9741,#7427,#7428);
#6728=AXIS2_PLACEMENT_3D('',#9765,#7430,#7431);
#6729=AXIS2_PLACEMENT_3D('',#9790,#7433,#7434);
#6730=AXIS2_PLACEMENT_3D('',#9814,#7436,#7437);
#6731=AXIS2_PLACEMENT_3D('',#9839,#7439,#7440);
#6732=AXIS2_PLACEMENT_3D('',#9864,#7442,#7443);
#6733=AXIS2_PLACEMENT_3D('',#9888,#7445,#7446);
#6734=AXIS2_PLACEMENT_3D('',#9913,#7448,#7449);
#6735=AXIS2_PLACEMENT_3D('',#9937,#7451,#7452);
#6736=AXIS2_PLACEMENT_3D('',#9962,#7454,#7455);
#6737=AXIS2_PLACEMENT_3D('',#9987,#7457,#7458);
#6738=AXIS2_PLACEMENT_3D('',#10011,#7460,#7461);
#6739=AXIS2_PLACEMENT_3D('',#10022,#7463,#7464);
#6740=AXIS2_PLACEMENT_3D('',#10028,#7465,#7466);
#6741=AXIS2_PLACEMENT_3D('',#10053,#7468,#7469);
#6742=AXIS2_PLACEMENT_3D('',#10061,#7471,#7472);
#6743=AXIS2_PLACEMENT_3D('',#10084,#7473,#7474);
#6744=AXIS2_PLACEMENT_3D('',#10135,#7476,#7477);
#6745=AXIS2_PLACEMENT_3D('',#10183,#7479,#7480);
#6746=AXIS2_PLACEMENT_3D('',#10234,#7482,#7483);
#6747=AXIS2_PLACEMENT_3D('',#10285,#7485,#7486);
#6748=AXIS2_PLACEMENT_3D('',#10333,#7488,#7489);
#6749=AXIS2_PLACEMENT_3D('',#10381,#7491,#7492);
#6750=AXIS2_PLACEMENT_3D('',#10432,#7494,#7495);
#6751=AXIS2_PLACEMENT_3D('',#10480,#7497,#7498);
#6752=AXIS2_PLACEMENT_3D('',#10528,#7500,#7501);
#6753=AXIS2_PLACEMENT_3D('',#10579,#7503,#7504);
#6754=AXIS2_PLACEMENT_3D('',#10630,#7506,#7507);
#6755=AXIS2_PLACEMENT_3D('',#10678,#7509,#7510);
#6756=AXIS2_PLACEMENT_3D('',#10729,#7512,#7513);
#6757=AXIS2_PLACEMENT_3D('',#10748,#7515,#7516);
#6758=AXIS2_PLACEMENT_3D('',#10768,#7517,#7518);
#6759=AXIS2_PLACEMENT_3D('',#10780,#7520,#7521);
#6760=AXIS2_PLACEMENT_3D('',#10788,#7522,#7523);
#6761=AXIS2_PLACEMENT_3D('',#10812,#7525,#7526);
#6762=AXIS2_PLACEMENT_3D('',#10837,#7528,#7529);
#6763=AXIS2_PLACEMENT_3D('',#10862,#7531,#7532);
#6764=AXIS2_PLACEMENT_3D('',#10886,#7534,#7535);
#6765=AXIS2_PLACEMENT_3D('',#10911,#7537,#7538);
#6766=AXIS2_PLACEMENT_3D('',#10935,#7540,#7541);
#6767=AXIS2_PLACEMENT_3D('',#10960,#7543,#7544);
#6768=AXIS2_PLACEMENT_3D('',#10985,#7546,#7547);
#6769=AXIS2_PLACEMENT_3D('',#11009,#7549,#7550);
#6770=AXIS2_PLACEMENT_3D('',#11034,#7552,#7553);
#6771=AXIS2_PLACEMENT_3D('',#11058,#7555,#7556);
#6772=AXIS2_PLACEMENT_3D('',#11083,#7558,#7559);
#6773=AXIS2_PLACEMENT_3D('',#11108,#7561,#7562);
#6774=AXIS2_PLACEMENT_3D('',#11132,#7564,#7565);
#6775=AXIS2_PLACEMENT_3D('',#11143,#7567,#7568);
#6776=AXIS2_PLACEMENT_3D('',#11149,#7569,#7570);
#6777=AXIS2_PLACEMENT_3D('',#11323,#7571,#7572);
#6778=AXIS2_PLACEMENT_3D('',#12391,#7573,#7574);
#6779=AXIS2_PLACEMENT_3D('',#12392,#7575,#7576);
#6780=AXIS2_PLACEMENT_3D('',#12566,#7577,#7578);
#6781=AXIS2_PLACEMENT_3D('',#13634,#7579,#7580);
#6782=AXIS2_PLACEMENT_3D('',#13635,#7581,#7582);
#6783=AXIS2_PLACEMENT_3D('',#13636,#7583,#7584);
#6784=AXIS2_PLACEMENT_3D('',#13637,#7585,#7586);
#6785=AXIS2_PLACEMENT_3D('',#13639,#7587,#7588);
#6786=AXIS2_PLACEMENT_3D('',#13642,#7590,#7591);
#6787=AXIS2_PLACEMENT_3D('',#13643,#7592,#7593);
#6788=AXIS2_PLACEMENT_3D('',#13645,#7594,#7595);
#6789=AXIS2_PLACEMENT_3D('',#13648,#7597,#7598);
#6790=AXIS2_PLACEMENT_3D('',#13649,#7599,#7600);
#6791=AXIS2_PLACEMENT_3D('',#13651,#7601,#7602);
#6792=AXIS2_PLACEMENT_3D('',#13654,#7604,#7605);
#6793=AXIS2_PLACEMENT_3D('',#13655,#7606,#7607);
#6794=AXIS2_PLACEMENT_3D('',#13664,#7612,#7613);
#6795=AXIS2_PLACEMENT_3D('',#13673,#7618,#7619);
#6796=AXIS2_PLACEMENT_3D('',#13676,#7622,#7623);
#6797=AXIS2_PLACEMENT_3D('',#13682,#7627,#7628);
#6798=AXIS2_PLACEMENT_3D('',#13688,#7632,#7633);
#6799=AXIS2_PLACEMENT_3D('',#13697,#7638,#7639);
#6800=AXIS2_PLACEMENT_3D('',#13703,#7643,#7644);
#6801=AXIS2_PLACEMENT_3D('',#13709,#7648,#7649);
#6802=AXIS2_PLACEMENT_3D('',#13711,#7651,#7652);
#6803=AXIS2_PLACEMENT_3D('',#13745,#7670,#7671);
#6804=AXIS2_PLACEMENT_3D('',#13748,#7674,#7675);
#6805=AXIS2_PLACEMENT_3D('',#13750,#7677,#7678);
#6806=AXIS2_PLACEMENT_3D('',#13752,#7680,#7681);
#6807=AXIS2_PLACEMENT_3D('',#13766,#7689,#7690);
#6808=AXIS2_PLACEMENT_3D('',#13772,#7694,#7695);
#6809=AXIS2_PLACEMENT_3D('',#13776,#7698,#7699);
#6810=AXIS2_PLACEMENT_3D('',#13780,#7702,#7703);
#6811=AXIS2_PLACEMENT_3D('',#13782,#7705,#7706);
#6812=AXIS2_PLACEMENT_3D('',#13788,#7710,#7711);
#6813=AXIS2_PLACEMENT_3D('',#13792,#7714,#7715);
#6814=AXIS2_PLACEMENT_3D('',#13796,#7718,#7719);
#6815=AXIS2_PLACEMENT_3D('',#13798,#7721,#7722);
#6816=AXIS2_PLACEMENT_3D('',#13812,#7730,#7731);
#6817=AXIS2_PLACEMENT_3D('',#13816,#7734,#7735);
#6818=AXIS2_PLACEMENT_3D('',#13822,#7739,#7740);
#6819=AXIS2_PLACEMENT_3D('',#13826,#7743,#7744);
#6820=AXIS2_PLACEMENT_3D('',#13833,#7749,#7750);
#6821=AXIS2_PLACEMENT_3D('',#13835,#7752,#7753);
#6822=AXIS2_PLACEMENT_3D('',#13836,#7754,#7755);
#6823=AXIS2_PLACEMENT_3D('',#13840,#7758,#7759);
#6824=AXIS2_PLACEMENT_3D('',#13844,#7762,#7763);
#6825=AXIS2_PLACEMENT_3D('',#13847,#7766,#7767);
#6826=AXIS2_PLACEMENT_3D('',#13848,#7768,#7769);
#7359=DIRECTION('axis',(0.,0.,1.));
#7360=DIRECTION('refdir',(1.,0.,0.));
#7361=DIRECTION('center_axis',(0.,0.,-1.));
#7362=DIRECTION('ref_axis',(1.,0.,0.));
#7363=DIRECTION('',(0.,0.,-1.));
#7364=DIRECTION('center_axis',(0.,0.,1.));
#7365=DIRECTION('ref_axis',(1.,0.,0.));
#7366=DIRECTION('',(0.,0.,-1.));
#7367=DIRECTION('center_axis',(0.,0.,1.));
#7368=DIRECTION('ref_axis',(1.,0.,0.));
#7369=DIRECTION('center_axis',(0.,0.,-1.));
#7370=DIRECTION('ref_axis',(1.,0.,0.));
#7371=DIRECTION('',(0.,0.,-1.));
#7372=DIRECTION('center_axis',(0.,0.,-1.));
#7373=DIRECTION('ref_axis',(1.,0.,0.));
#7374=DIRECTION('',(0.,0.,-1.));
#7375=DIRECTION('center_axis',(0.,0.,-1.));
#7376=DIRECTION('ref_axis',(1.,0.,0.));
#7377=DIRECTION('',(0.,0.,-1.));
#7378=DIRECTION('center_axis',(0.,0.,-1.));
#7379=DIRECTION('ref_axis',(1.,0.,0.));
#7380=DIRECTION('',(0.,0.,-1.));
#7381=DIRECTION('center_axis',(0.,0.,-1.));
#7382=DIRECTION('ref_axis',(1.,0.,0.));
#7383=DIRECTION('',(0.,0.,-1.));
#7384=DIRECTION('center_axis',(0.,0.,-1.));
#7385=DIRECTION('ref_axis',(1.,0.,0.));
#7386=DIRECTION('',(0.,0.,-1.));
#7387=DIRECTION('center_axis',(0.,0.,-1.));
#7388=DIRECTION('ref_axis',(1.,0.,0.));
#7389=DIRECTION('',(0.,0.,-1.));
#7390=DIRECTION('center_axis',(0.,0.,-1.));
#7391=DIRECTION('ref_axis',(1.,0.,0.));
#7392=DIRECTION('',(0.,0.,-1.));
#7393=DIRECTION('center_axis',(0.,0.,-1.));
#7394=DIRECTION('ref_axis',(1.,0.,0.));
#7395=DIRECTION('',(0.,0.,-1.));
#7396=DIRECTION('center_axis',(0.,0.,-1.));
#7397=DIRECTION('ref_axis',(1.,0.,0.));
#7398=DIRECTION('',(0.,0.,-1.));
#7399=DIRECTION('center_axis',(0.,0.,-1.));
#7400=DIRECTION('ref_axis',(1.,0.,0.));
#7401=DIRECTION('',(0.,0.,-1.));
#7402=DIRECTION('center_axis',(0.,0.,-1.));
#7403=DIRECTION('ref_axis',(1.,0.,0.));
#7404=DIRECTION('',(0.,0.,-1.));
#7405=DIRECTION('center_axis',(0.,0.,-1.));
#7406=DIRECTION('ref_axis',(1.,0.,0.));
#7407=DIRECTION('',(0.,0.,-1.));
#7408=DIRECTION('center_axis',(0.,0.,-1.));
#7409=DIRECTION('ref_axis',(0.938438541741608,-0.345446238036955,0.));
#7410=DIRECTION('',(0.,0.,-1.));
#7411=DIRECTION('center_axis',(0.,0.,-1.));
#7412=DIRECTION('ref_axis',(1.,0.,0.));
#7413=DIRECTION('center_axis',(0.,0.,-1.));
#7414=DIRECTION('ref_axis',(0.0179644034331435,0.999838627084037,0.));
#7415=DIRECTION('',(1.22464679914735E-16,-8.74945686026681E-30,-1.));
#7416=DIRECTION('center_axis',(0.,0.,1.));
#7417=DIRECTION('ref_axis',(1.,-7.13222724178225E-14,0.));
#7418=DIRECTION('center_axis',(0.,0.,-1.));
#7419=DIRECTION('ref_axis',(1.,-7.13222724178225E-14,0.));
#7420=DIRECTION('',(1.22464679914735E-16,-8.74945686026681E-30,-1.));
#7421=DIRECTION('center_axis',(0.,0.,-1.));
#7422=DIRECTION('ref_axis',(1.,-7.13222724178225E-14,0.));
#7423=DIRECTION('',(1.22464679914735E-16,-8.74945686026681E-30,-1.));
#7424=DIRECTION('center_axis',(0.,0.,-1.));
#7425=DIRECTION('ref_axis',(1.,-7.13222724178225E-14,0.));
#7426=DIRECTION('',(1.22464679914735E-16,-8.74945686026681E-30,-1.));
#7427=DIRECTION('center_axis',(0.,0.,-1.));
#7428=DIRECTION('ref_axis',(1.,-7.13222724178225E-14,0.));
#7429=DIRECTION('',(1.22464679914735E-16,-8.74945686026681E-30,-1.));
#7430=DIRECTION('center_axis',(0.,0.,-1.));
#7431=DIRECTION('ref_axis',(1.,-7.13222724178225E-14,0.));
#7432=DIRECTION('',(1.22464679914735E-16,-8.74945686026681E-30,-1.));
#7433=DIRECTION('center_axis',(0.,0.,-1.));
#7434=DIRECTION('ref_axis',(1.,-7.13222724178225E-14,0.));
#7435=DIRECTION('',(1.22464679914735E-16,-8.74945686026681E-30,-1.));
#7436=DIRECTION('center_axis',(0.,0.,-1.));
#7437=DIRECTION('ref_axis',(1.,-7.13222724178225E-14,0.));
#7438=DIRECTION('',(1.22464679914735E-16,-8.74945686026681E-30,-1.));
#7439=DIRECTION('center_axis',(0.,0.,-1.));
#7440=DIRECTION('ref_axis',(1.,-7.13222724178225E-14,0.));
#7441=DIRECTION('',(1.22464679914735E-16,-8.74945686026681E-30,-1.));
#7442=DIRECTION('center_axis',(0.,0.,-1.));
#7443=DIRECTION('ref_axis',(1.,-7.13222724178225E-14,0.));
#7444=DIRECTION('',(1.22464679914735E-16,-8.74945686026681E-30,-1.));
#7445=DIRECTION('center_axis',(0.,0.,-1.));
#7446=DIRECTION('ref_axis',(1.,-7.13222724178225E-14,0.));
#7447=DIRECTION('',(1.22464679914735E-16,-8.74945686026681E-30,-1.));
#7448=DIRECTION('center_axis',(0.,0.,-1.));
#7449=DIRECTION('ref_axis',(1.,-7.13222724178225E-14,0.));
#7450=DIRECTION('',(1.22464679914735E-16,-8.74945686026681E-30,-1.));
#7451=DIRECTION('center_axis',(0.,0.,-1.));
#7452=DIRECTION('ref_axis',(1.,-7.13222724178225E-14,0.));
#7453=DIRECTION('',(1.22464679914735E-16,-8.74945686026681E-30,-1.));
#7454=DIRECTION('center_axis',(0.,0.,-1.));
#7455=DIRECTION('ref_axis',(1.,-7.13222724178225E-14,0.));
#7456=DIRECTION('',(1.22464679914735E-16,-8.74945686026681E-30,-1.));
#7457=DIRECTION('center_axis',(0.,0.,-1.));
#7458=DIRECTION('ref_axis',(1.,-7.13222724178225E-14,0.));
#7459=DIRECTION('',(1.22464679914735E-16,-8.74945686026681E-30,-1.));
#7460=DIRECTION('center_axis',(0.,0.,-1.));
#7461=DIRECTION('ref_axis',(-0.609341687186091,-0.792907755200571,0.));
#7462=DIRECTION('',(1.22464679914735E-16,-8.74945686026681E-30,-1.));
#7463=DIRECTION('center_axis',(0.,0.,-1.));
#7464=DIRECTION('ref_axis',(1.,-7.13222724178225E-14,0.));
#7465=DIRECTION('center_axis',(0.,0.,-1.));
#7466=DIRECTION('ref_axis',(1.,0.,0.));
#7467=DIRECTION('',(0.,0.,-1.));
#7468=DIRECTION('center_axis',(0.,0.,1.));
#7469=DIRECTION('ref_axis',(1.,0.,0.));
#7470=DIRECTION('',(0.,0.,-1.));
#7471=DIRECTION('center_axis',(0.,0.,1.));
#7472=DIRECTION('ref_axis',(1.,0.,0.));
#7473=DIRECTION('center_axis',(0.,0.,-1.));
#7474=DIRECTION('ref_axis',(1.,0.,0.));
#7475=DIRECTION('',(0.,0.,-1.));
#7476=DIRECTION('center_axis',(0.,0.,-1.));
#7477=DIRECTION('ref_axis',(1.,0.,0.));
#7478=DIRECTION('',(0.,0.,-1.));
#7479=DIRECTION('center_axis',(0.,0.,-1.));
#7480=DIRECTION('ref_axis',(1.,0.,0.));
#7481=DIRECTION('',(0.,0.,-1.));
#7482=DIRECTION('center_axis',(0.,0.,-1.));
#7483=DIRECTION('ref_axis',(1.,0.,0.));
#7484=DIRECTION('',(0.,0.,-1.));
#7485=DIRECTION('center_axis',(0.,0.,-1.));
#7486=DIRECTION('ref_axis',(1.,0.,0.));
#7487=DIRECTION('',(0.,0.,-1.));
#7488=DIRECTION('center_axis',(0.,0.,-1.));
#7489=DIRECTION('ref_axis',(1.,0.,0.));
#7490=DIRECTION('',(0.,0.,-1.));
#7491=DIRECTION('center_axis',(0.,0.,-1.));
#7492=DIRECTION('ref_axis',(1.,0.,0.));
#7493=DIRECTION('',(0.,0.,-1.));
#7494=DIRECTION('center_axis',(0.,0.,-1.));
#7495=DIRECTION('ref_axis',(1.,0.,0.));
#7496=DIRECTION('',(0.,0.,-1.));
#7497=DIRECTION('center_axis',(0.,0.,-1.));
#7498=DIRECTION('ref_axis',(1.,0.,0.));
#7499=DIRECTION('',(0.,0.,-1.));
#7500=DIRECTION('center_axis',(0.,0.,-1.));
#7501=DIRECTION('ref_axis',(1.,0.,0.));
#7502=DIRECTION('',(0.,0.,-1.));
#7503=DIRECTION('center_axis',(0.,0.,-1.));
#7504=DIRECTION('ref_axis',(1.,0.,0.));
#7505=DIRECTION('',(0.,0.,-1.));
#7506=DIRECTION('center_axis',(0.,0.,-1.));
#7507=DIRECTION('ref_axis',(1.,0.,0.));
#7508=DIRECTION('',(0.,0.,-1.));
#7509=DIRECTION('center_axis',(0.,0.,-1.));
#7510=DIRECTION('ref_axis',(1.,0.,0.));
#7511=DIRECTION('',(0.,0.,-1.));
#7512=DIRECTION('center_axis',(0.,0.,-1.));
#7513=DIRECTION('ref_axis',(0.93843855055824,-0.345446214085711,0.));
#7514=DIRECTION('',(0.,0.,-1.));
#7515=DIRECTION('center_axis',(0.,0.,-1.));
#7516=DIRECTION('ref_axis',(1.,0.,0.));
#7517=DIRECTION('center_axis',(0.,0.,-1.));
#7518=DIRECTION('ref_axis',(0.0179644055674462,0.999838627045689,0.));
#7519=DIRECTION('',(1.22464679914735E-16,-8.74945686026681E-30,-1.));
#7520=DIRECTION('center_axis',(0.,0.,1.));
#7521=DIRECTION('ref_axis',(1.,-7.13222724178225E-14,0.));
#7522=DIRECTION('center_axis',(0.,0.,-1.));
#7523=DIRECTION('ref_axis',(1.,-7.13222724178225E-14,0.));
#7524=DIRECTION('',(1.22464679914735E-16,-8.74945686026681E-30,-1.));
#7525=DIRECTION('center_axis',(0.,0.,-1.));
#7526=DIRECTION('ref_axis',(1.,-7.13222724178225E-14,0.));
#7527=DIRECTION('',(1.22464679914735E-16,-8.74945686026681E-30,-1.));
#7528=DIRECTION('center_axis',(0.,0.,-1.));
#7529=DIRECTION('ref_axis',(1.,-7.13222724178225E-14,0.));
#7530=DIRECTION('',(1.22464679914735E-16,-8.74945686026681E-30,-1.));
#7531=DIRECTION('center_axis',(0.,0.,-1.));
#7532=DIRECTION('ref_axis',(1.,-7.13222724178225E-14,0.));
#7533=DIRECTION('',(1.22464679914735E-16,-8.74945686026681E-30,-1.));
#7534=DIRECTION('center_axis',(0.,0.,-1.));
#7535=DIRECTION('ref_axis',(1.,-7.13222724178225E-14,0.));
#7536=DIRECTION('',(1.22464679914735E-16,-8.74945686026681E-30,-1.));
#7537=DIRECTION('center_axis',(0.,0.,-1.));
#7538=DIRECTION('ref_axis',(1.,-7.13222724178225E-14,0.));
#7539=DIRECTION('',(1.22464679914735E-16,-8.74945686026681E-30,-1.));
#7540=DIRECTION('center_axis',(0.,0.,-1.));
#7541=DIRECTION('ref_axis',(1.,-7.13222724178225E-14,0.));
#7542=DIRECTION('',(1.22464679914735E-16,-8.74945686026681E-30,-1.));
#7543=DIRECTION('center_axis',(0.,0.,-1.));
#7544=DIRECTION('ref_axis',(1.,-7.13222724178225E-14,0.));
#7545=DIRECTION('',(1.22464679914735E-16,-8.74945686026681E-30,-1.));
#7546=DIRECTION('center_axis',(0.,0.,-1.));
#7547=DIRECTION('ref_axis',(1.,-7.13222724178225E-14,0.));
#7548=DIRECTION('',(1.22464679914735E-16,-8.74945686026681E-30,-1.));
#7549=DIRECTION('center_axis',(0.,0.,-1.));
#7550=DIRECTION('ref_axis',(1.,-7.13222724178225E-14,0.));
#7551=DIRECTION('',(1.22464679914735E-16,-8.74945686026681E-30,-1.));
#7552=DIRECTION('center_axis',(0.,0.,-1.));
#7553=DIRECTION('ref_axis',(1.,-7.13222724178225E-14,0.));
#7554=DIRECTION('',(1.22464679914735E-16,-8.74945686026681E-30,-1.));
#7555=DIRECTION('center_axis',(0.,0.,-1.));
#7556=DIRECTION('ref_axis',(1.,-7.13222724178225E-14,0.));
#7557=DIRECTION('',(1.22464679914735E-16,-8.74945686026681E-30,-1.));
#7558=DIRECTION('center_axis',(0.,0.,-1.));
#7559=DIRECTION('ref_axis',(1.,-7.13222724178225E-14,0.));
#7560=DIRECTION('',(1.22464679914735E-16,-8.74945686026681E-30,-1.));
#7561=DIRECTION('center_axis',(0.,0.,-1.));
#7562=DIRECTION('ref_axis',(1.,-7.13222724178225E-14,0.));
#7563=DIRECTION('',(1.22464679914735E-16,-8.74945686026681E-30,-1.));
#7564=DIRECTION('center_axis',(0.,0.,-1.));
#7565=DIRECTION('ref_axis',(-0.609341710614343,-0.792907737196193,0.));
#7566=DIRECTION('',(1.22464679914735E-16,-8.74945686026681E-30,-1.));
#7567=DIRECTION('center_axis',(0.,0.,-1.));
#7568=DIRECTION('ref_axis',(1.,-7.13222724178225E-14,0.));
#7569=DIRECTION('center_axis',(0.,0.,1.));
#7570=DIRECTION('ref_axis',(1.,0.,0.));
#7571=DIRECTION('center_axis',(0.,0.,-1.));
#7572=DIRECTION('ref_axis',(1.,-7.13222724178225E-14,0.));
#7573=DIRECTION('center_axis',(0.,0.,-1.));
#7574=DIRECTION('ref_axis',(1.,0.,0.));
#7575=DIRECTION('center_axis',(0.,0.,1.));
#7576=DIRECTION('ref_axis',(1.,0.,0.));
#7577=DIRECTION('center_axis',(0.,0.,-1.));
#7578=DIRECTION('ref_axis',(1.,-7.13222724178225E-14,0.));
#7579=DIRECTION('center_axis',(0.,0.,-1.));
#7580=DIRECTION('ref_axis',(1.,0.,0.));
#7581=DIRECTION('center_axis',(0.,0.,-1.));
#7582=DIRECTION('ref_axis',(1.,0.,0.));
#7583=DIRECTION('center_axis',(0.,0.,-1.));
#7584=DIRECTION('ref_axis',(1.,0.,0.));
#7585=DIRECTION('center_axis',(0.,-1.,0.));
#7586=DIRECTION('ref_axis',(0.,0.,1.));
#7587=DIRECTION('center_axis',(0.,-1.,0.));
#7588=DIRECTION('ref_axis',(0.,0.,1.));
#7589=DIRECTION('',(0.,-1.,0.));
#7590=DIRECTION('center_axis',(0.,1.,0.));
#7591=DIRECTION('ref_axis',(0.,0.,1.));
#7592=DIRECTION('center_axis',(0.,-1.,0.));
#7593=DIRECTION('ref_axis',(0.,0.,1.));
#7594=DIRECTION('center_axis',(0.,-1.,0.));
#7595=DIRECTION('ref_axis',(0.,0.,1.));
#7596=DIRECTION('',(0.,-1.,0.));
#7597=DIRECTION('center_axis',(0.,1.,0.));
#7598=DIRECTION('ref_axis',(0.,0.,1.));
#7599=DIRECTION('center_axis',(0.,-1.,0.));
#7600=DIRECTION('ref_axis',(0.,0.,1.));
#7601=DIRECTION('center_axis',(0.,-1.,0.));
#7602=DIRECTION('ref_axis',(0.,0.,1.));
#7603=DIRECTION('',(0.,-1.,0.));
#7604=DIRECTION('center_axis',(0.,1.,0.));
#7605=DIRECTION('ref_axis',(0.,0.,1.));
#7606=DIRECTION('center_axis',(-1.,0.,0.));
#7607=DIRECTION('ref_axis',(0.,-1.,0.));
#7608=DIRECTION('',(0.,-1.,0.));
#7609=DIRECTION('',(0.,0.,1.));
#7610=DIRECTION('',(0.,-1.,0.));
#7611=DIRECTION('',(0.,0.,1.));
#7612=DIRECTION('center_axis',(1.,0.,0.));
#7613=DIRECTION('ref_axis',(0.,1.,0.));
#7614=DIRECTION('',(0.,1.,0.));
#7615=DIRECTION('',(0.,0.,1.));
#7616=DIRECTION('',(0.,1.,0.));
#7617=DIRECTION('',(0.,0.,1.));
#7618=DIRECTION('center_axis',(0.,0.,1.));
#7619=DIRECTION('ref_axis',(1.,0.,0.));
#7620=DIRECTION('',(-1.,0.,0.));
#7621=DIRECTION('',(1.,0.,0.));
#7622=DIRECTION('center_axis',(0.,0.,1.));
#7623=DIRECTION('ref_axis',(1.,0.,0.));
#7624=DIRECTION('',(1.,0.,0.));
#7625=DIRECTION('',(0.,-1.,0.));
#7626=DIRECTION('',(-1.,0.,0.));
#7627=DIRECTION('center_axis',(0.,0.,1.));
#7628=DIRECTION('ref_axis',(1.,0.,0.));
#7629=DIRECTION('',(-1.,0.,0.));
#7630=DIRECTION('',(0.,1.,0.));
#7631=DIRECTION('',(1.,0.,0.));
#7632=DIRECTION('center_axis',(0.,-1.,0.));
#7633=DIRECTION('ref_axis',(1.,0.,0.));
#7634=DIRECTION('',(1.,0.,0.));
#7635=DIRECTION('',(0.,0.,1.));
#7636=DIRECTION('',(1.,0.,0.));
#7637=DIRECTION('',(0.,0.,1.));
#7638=DIRECTION('center_axis',(-1.,0.,0.));
#7639=DIRECTION('ref_axis',(0.,-1.,0.));
#7640=DIRECTION('',(0.,-1.,0.));
#7641=DIRECTION('',(0.,0.,1.));
#7642=DIRECTION('',(0.,-1.,0.));
#7643=DIRECTION('center_axis',(1.,0.,0.));
#7644=DIRECTION('ref_axis',(0.,1.,0.));
#7645=DIRECTION('',(0.,1.,0.));
#7646=DIRECTION('',(0.,1.,0.));
#7647=DIRECTION('',(0.,0.,1.));
#7648=DIRECTION('center_axis',(0.,0.,1.));
#7649=DIRECTION('ref_axis',(1.,0.,0.));
#7650=DIRECTION('',(-1.,0.,0.));
#7651=DIRECTION('center_axis',(0.,0.,1.));
#7652=DIRECTION('ref_axis',(1.,0.,0.));
#7653=DIRECTION('',(-1.,0.,0.));
#7654=DIRECTION('',(0.,1.,0.));
#7655=DIRECTION('',(1.,0.,0.));
#7656=DIRECTION('',(0.,1.,0.));
#7657=DIRECTION('',(-1.,0.,0.));
#7658=DIRECTION('',(0.,-1.,0.));
#7659=DIRECTION('',(1.,0.,0.));
#7660=DIRECTION('',(0.,-1.,0.));
#7661=DIRECTION('',(-1.,0.,0.));
#7662=DIRECTION('',(1.,0.,0.));
#7663=DIRECTION('',(0.,1.,0.));
#7664=DIRECTION('',(-1.,0.,0.));
#7665=DIRECTION('',(0.,-1.,0.));
#7666=DIRECTION('',(1.,0.,0.));
#7667=DIRECTION('',(0.,1.,0.));
#7668=DIRECTION('',(-1.,0.,0.));
#7669=DIRECTION('',(0.,-1.,0.));
#7670=DIRECTION('center_axis',(0.,1.,0.));
#7671=DIRECTION('ref_axis',(-1.,0.,0.));
#7672=DIRECTION('',(0.,0.,1.));
#7673=DIRECTION('',(0.,0.,1.));
#7674=DIRECTION('center_axis',(1.,0.,0.));
#7675=DIRECTION('ref_axis',(0.,1.,0.));
#7676=DIRECTION('',(0.,0.,1.));
#7677=DIRECTION('center_axis',(-1.,0.,0.));
#7678=DIRECTION('ref_axis',(0.,-1.,0.));
#7679=DIRECTION('',(0.,0.,1.));
#7680=DIRECTION('center_axis',(0.,-1.,0.));
#7681=DIRECTION('ref_axis',(1.,0.,0.));
#7682=DIRECTION('',(0.,0.,1.));
#7683=DIRECTION('',(1.,0.,0.));
#7684=DIRECTION('',(0.,0.,-1.));
#7685=DIRECTION('',(-1.,0.,0.));
#7686=DIRECTION('',(0.,0.,1.));
#7687=DIRECTION('',(1.,0.,0.));
#7688=DIRECTION('',(0.,0.,1.));
#7689=DIRECTION('center_axis',(0.,-1.,0.));
#7690=DIRECTION('ref_axis',(-1.,0.,0.));
#7691=DIRECTION('',(-1.,0.,0.));
#7692=DIRECTION('',(0.,0.,-1.));
#7693=DIRECTION('',(0.,0.,-1.));
#7694=DIRECTION('center_axis',(1.,0.,0.));
#7695=DIRECTION('ref_axis',(0.,-1.,0.));
#7696=DIRECTION('',(0.,-1.,0.));
#7697=DIRECTION('',(0.,0.,-1.));
#7698=DIRECTION('center_axis',(0.,1.,0.));
#7699=DIRECTION('ref_axis',(1.,0.,0.));
#7700=DIRECTION('',(1.,0.,0.));
#7701=DIRECTION('',(0.,0.,-1.));
#7702=DIRECTION('center_axis',(-1.,0.,0.));
#7703=DIRECTION('ref_axis',(0.,1.,0.));
#7704=DIRECTION('',(0.,1.,0.));
#7705=DIRECTION('center_axis',(0.,-1.,0.));
#7706=DIRECTION('ref_axis',(-1.,0.,0.));
#7707=DIRECTION('',(-1.,0.,0.));
#7708=DIRECTION('',(0.,0.,-1.));
#7709=DIRECTION('',(0.,0.,-1.));
#7710=DIRECTION('center_axis',(1.,0.,0.));
#7711=DIRECTION('ref_axis',(0.,-1.,0.));
#7712=DIRECTION('',(0.,-1.,0.));
#7713=DIRECTION('',(0.,0.,-1.));
#7714=DIRECTION('center_axis',(0.,1.,0.));
#7715=DIRECTION('ref_axis',(1.,0.,0.));
#7716=DIRECTION('',(1.,0.,0.));
#7717=DIRECTION('',(0.,0.,-1.));
#7718=DIRECTION('center_axis',(-1.,0.,0.));
#7719=DIRECTION('ref_axis',(0.,1.,0.));
#7720=DIRECTION('',(0.,1.,0.));
#7721=DIRECTION('center_axis',(-1.,0.,0.));
#7722=DIRECTION('ref_axis',(0.,-1.,0.));
#7723=DIRECTION('',(0.,0.,-1.));
#7724=DIRECTION('',(0.,1.,0.));
#7725=DIRECTION('',(0.,-1.,0.));
#7726=DIRECTION('',(0.,0.,1.));
#7727=DIRECTION('',(0.,-1.,0.));
#7728=DIRECTION('',(0.,0.,1.));
#7729=DIRECTION('',(0.,-1.,0.));
#7730=DIRECTION('center_axis',(0.,0.,1.));
#7731=DIRECTION('ref_axis',(1.,0.,0.));
#7732=DIRECTION('',(0.,1.,0.));
#7733=DIRECTION('',(1.,0.,0.));
#7734=DIRECTION('center_axis',(0.,0.,1.));
#7735=DIRECTION('ref_axis',(1.,0.,0.));
#7736=DIRECTION('',(1.,0.,0.));
#7737=DIRECTION('',(-1.,0.,0.));
#7738=DIRECTION('',(0.,1.,0.));
#7739=DIRECTION('center_axis',(0.,1.,0.));
#7740=DIRECTION('ref_axis',(-1.,0.,0.));
#7741=DIRECTION('',(-1.,0.,0.));
#7742=DIRECTION('',(0.,0.,1.));
#7743=DIRECTION('center_axis',(1.,0.,0.));
#7744=DIRECTION('ref_axis',(0.,1.,0.));
#7745=DIRECTION('',(0.,0.,1.));
#7746=DIRECTION('',(0.,1.,0.));
#7747=DIRECTION('',(0.,0.,1.));
#7748=DIRECTION('',(0.,-1.,0.));
#7749=DIRECTION('center_axis',(0.,-1.,0.));
#7750=DIRECTION('ref_axis',(1.,0.,0.));
#7751=DIRECTION('',(1.,0.,0.));
#7752=DIRECTION('center_axis',(0.,0.,1.));
#7753=DIRECTION('ref_axis',(1.,0.,0.));
#7754=DIRECTION('center_axis',(0.,0.,1.));
#7755=DIRECTION('ref_axis',(1.,0.,0.));
#7756=DIRECTION('',(-1.,0.,0.));
#7757=DIRECTION('',(0.,-1.,0.));
#7758=DIRECTION('center_axis',(0.,0.,1.));
#7759=DIRECTION('ref_axis',(1.,0.,0.));
#7760=DIRECTION('',(0.,1.,0.));
#7761=DIRECTION('',(-1.,0.,0.));
#7762=DIRECTION('center_axis',(0.,1.,0.));
#7763=DIRECTION('ref_axis',(-1.,0.,0.));
#7764=DIRECTION('',(0.,0.,1.));
#7765=DIRECTION('',(0.,0.,1.));
#7766=DIRECTION('center_axis',(1.,0.,0.));
#7767=DIRECTION('ref_axis',(0.,1.,0.));
#7768=DIRECTION('center_axis',(-1.,0.,0.));
#7769=DIRECTION('ref_axis',(0.,-1.,0.));
#8906=CARTESIAN_POINT('',(0.,0.,0.));
#8907=CARTESIAN_POINT('Origin',(83.,23.,-12.));
#8908=CARTESIAN_POINT('',(81.3313534283113,22.999608308332,-16.2285196366098));
#8909=CARTESIAN_POINT('',(81.3334663741701,23.0014782390593,-16.4214803633902));
#8910=CARTESIAN_POINT('',(81.334,23.,-12.));
#8911=CARTESIAN_POINT('',(82.2300979593295,21.5225674811446,-17.));
#8912=CARTESIAN_POINT('Ctrl Pts',(81.3334663741701,23.0014782390593,-16.4214803633902));
#8913=CARTESIAN_POINT('Ctrl Pts',(81.3324167265455,23.1152856061038,-16.4290983789409));
#8914=CARTESIAN_POINT('Ctrl Pts',(81.3430834208759,23.2288980499925,-16.4367163944915));
#8915=CARTESIAN_POINT('Ctrl Pts',(81.366191211586,23.3399236516146,-16.4443344100422));
#8916=CARTESIAN_POINT('Ctrl Pts',(81.4785582190846,23.8798114654899,-16.4813787827061));
#8917=CARTESIAN_POINT('Ctrl Pts',(81.8851094874654,24.3585303713383,-16.5184231553699));
#8918=CARTESIAN_POINT('Ctrl Pts',(82.3995343180334,24.5569680544574,-16.5554675280338));
#8919=CARTESIAN_POINT('Ctrl Pts',(82.9139591486014,24.7554057375764,-16.5925119006976));
#8920=CARTESIAN_POINT('Ctrl Pts',(83.5362575413566,24.6735621979661,-16.6295562733615));
#8921=CARTESIAN_POINT('Ctrl Pts',(83.9821832750364,24.348973723947,-16.6666006460253));
#8922=CARTESIAN_POINT('Ctrl Pts',(84.4281090087162,24.0243852499279,-16.7036450186892));
#8923=CARTESIAN_POINT('Ctrl Pts',(84.6976620833208,23.4570518415,-16.740689391353));
#8924=CARTESIAN_POINT('Ctrl Pts',(84.6664136128519,22.9064184197971,-16.7777337640169));
#8925=CARTESIAN_POINT('Ctrl Pts',(84.635165142383,22.3557849980942,-16.8147781366807));
#8926=CARTESIAN_POINT('Ctrl Pts',(84.3031151268407,21.8218515631163,-16.8518225093446));
#8927=CARTESIAN_POINT('Ctrl Pts',(83.8246634223492,21.5495472460214,-16.8888668820084));
#8928=CARTESIAN_POINT('Ctrl Pts',(83.3462117178578,21.2772429289266,-16.9259112546723));
#8929=CARTESIAN_POINT('Ctrl Pts',(82.7213583244172,21.2665677297147,-16.9629556273362));
#8930=CARTESIAN_POINT('Ctrl Pts',(82.2300979593296,21.5225674811446,-17.));
#8931=CARTESIAN_POINT('',(81.6629741098033,23.9990032536159,-17.));
#8932=CARTESIAN_POINT('Origin',(83.,23.,-17.));
#8933=CARTESIAN_POINT('',(81.3354782356987,22.9987789599865,-16.9285196366098));
#8934=CARTESIAN_POINT('Ctrl Pts',(81.6629726863575,23.9990044309052,-17.));
#8935=CARTESIAN_POINT('Ctrl Pts',(81.4510076185789,23.7145503593587,-16.9761732122033));
#8936=CARTESIAN_POINT('Ctrl Pts',(81.3378311765629,23.3559374868803,-16.9523464244065));
#8937=CARTESIAN_POINT('Ctrl Pts',(81.3354782356987,22.9987789599865,-16.9285196366098));
#8938=CARTESIAN_POINT('',(81.334,23.,-18.));
#8939=CARTESIAN_POINT('',(81.334,23.,-12.));
#8940=CARTESIAN_POINT('Origin',(83.,23.,-18.));
#8941=CARTESIAN_POINT('Ctrl Pts',(81.3354782356987,22.9987789599865,-16.9285196366098));
#8942=CARTESIAN_POINT('Ctrl Pts',(81.3342446902247,22.8115361392917,-16.9160282787975));
#8943=CARTESIAN_POINT('Ctrl Pts',(81.3634704623982,22.6246930386351,-16.9035369209851));
#8944=CARTESIAN_POINT('Ctrl Pts',(81.4248896518804,22.4491447215318,-16.8910455631728));
#8945=CARTESIAN_POINT('Ctrl Pts',(81.6070344097262,21.9285386051282,-16.8540011905089));
#8946=CARTESIAN_POINT('Ctrl Pts',(82.0723133280082,21.5072676735534,-16.8169568178451));
#8947=CARTESIAN_POINT('Ctrl Pts',(82.6082885703566,21.3778807889459,-16.7799124451812));
#8948=CARTESIAN_POINT('Ctrl Pts',(83.144263812705,21.2484939043384,-16.7428680725174));
#8949=CARTESIAN_POINT('Ctrl Pts',(83.7509353791199,21.4109910666983,-16.7058236998535));
#8950=CARTESIAN_POINT('Ctrl Pts',(84.1504372220724,21.7911271928933,-16.6687793271897));
#8951=CARTESIAN_POINT('Ctrl Pts',(84.549939065025,22.1712633190883,-16.6317349545258));
#8952=CARTESIAN_POINT('Ctrl Pts',(84.7422711845153,22.7690384091184,-16.594690581862));
#8953=CARTESIAN_POINT('Ctrl Pts',(84.639539482518,23.3108402472818,-16.5576462091981));
#8954=CARTESIAN_POINT('Ctrl Pts',(84.5368077805207,23.8526420854451,-16.5206018365343));
#8955=CARTESIAN_POINT('Ctrl Pts',(84.1390122570358,24.3384706717417,-16.4835574638704));
#8956=CARTESIAN_POINT('Ctrl Pts',(83.6281313759476,24.5460306512639,-16.4465130912066));
#8957=CARTESIAN_POINT('Ctrl Pts',(83.1172504948595,24.7535906307861,-16.4094687185427));
#8958=CARTESIAN_POINT('Ctrl Pts',(82.493284256168,24.6828820035339,-16.3724243458788));
#8959=CARTESIAN_POINT('Ctrl Pts',(82.0418022728353,24.3662477041162,-16.335379973215));
#8960=CARTESIAN_POINT('Ctrl Pts',(81.607678605813,24.0617871758054,-16.2997598610132));
#8961=CARTESIAN_POINT('Ctrl Pts',(81.3330310126921,23.5299478610255,-16.2641397488115));
#8962=CARTESIAN_POINT('Ctrl Pts',(81.3313534283113,22.999608308332,-16.2285196366098));
#8963=CARTESIAN_POINT('Origin',(83.,23.,-12.));
#8964=CARTESIAN_POINT('',(81.3344264707835,23.0015125425552,-15.5285196366098));
#8965=CARTESIAN_POINT('',(81.3367022839223,22.9999597918218,-15.7214803633902));
#8966=CARTESIAN_POINT('',(81.334,23.,-12.));
#8967=CARTESIAN_POINT('Ctrl Pts',(81.3367022839223,22.9999597918218,-15.7214803633902));
#8968=CARTESIAN_POINT('Ctrl Pts',(81.3367622982155,23.2804572295637,-15.7401654762911));
#8969=CARTESIAN_POINT('Ctrl Pts',(81.4039329804852,23.5609817981292,-15.758850589192));
#8970=CARTESIAN_POINT('Ctrl Pts',(81.5380528850521,23.8046577193695,-15.7775357020929));
#8971=CARTESIAN_POINT('Ctrl Pts',(81.8039537523775,24.2877600524149,-15.8145800747567));
#8972=CARTESIAN_POINT('Ctrl Pts',(82.3330017103809,24.6260270310476,-15.8516244474206));
#8973=CARTESIAN_POINT('Ctrl Pts',(82.8830897957813,24.6646603768711,-15.8886688200844));
#8974=CARTESIAN_POINT('Ctrl Pts',(83.4331778811817,24.7032937226946,-15.9257131927483));
#8975=CARTESIAN_POINT('Ctrl Pts',(84.0043060939791,24.442293435709,-15.9627575654121));
#8976=CARTESIAN_POINT('Ctrl Pts',(84.33512331298,24.001099683907,-15.999801938076));
#8977=CARTESIAN_POINT('Ctrl Pts',(84.6659405319808,23.559905932105,-16.0368463107398));
#8978=CARTESIAN_POINT('Ctrl Pts',(84.7564467571851,22.9385187154866,-16.0738906834037));
#8979=CARTESIAN_POINT('Ctrl Pts',(84.5652078284987,22.4212944599841,-16.1109350560675));
#8980=CARTESIAN_POINT('Ctrl Pts',(84.3739688998123,21.9040702044815,-16.1479794287314));
#8981=CARTESIAN_POINT('Ctrl Pts',(83.9009848172353,21.4910089100948,-16.1850238013952));
#8982=CARTESIAN_POINT('Ctrl Pts',(83.3627357719796,21.3711407259392,-16.2220681740591));
#8983=CARTESIAN_POINT('Ctrl Pts',(82.8244867267238,21.2512725417836,-16.2591125467229));
#8984=CARTESIAN_POINT('Ctrl Pts',(82.2209727187894,21.4245974678592,-16.2961569193868));
#8985=CARTESIAN_POINT('Ctrl Pts',(81.8283070881303,21.8117882918482,-16.3332012920507));
#8986=CARTESIAN_POINT('Ctrl Pts',(81.5163914517474,22.1193549919522,-16.3626276491638));
#8987=CARTESIAN_POINT('Ctrl Pts',(81.3375208822818,22.5618708107873,-16.392054006277));
#8988=CARTESIAN_POINT('Ctrl Pts',(81.3334663741701,23.0014782390593,-16.4214803633902));
#8989=CARTESIAN_POINT('Ctrl Pts',(81.3313534283113,22.999608308332,-16.2285196366098));
#8990=CARTESIAN_POINT('Ctrl Pts',(81.3312863505578,22.9784028260999,-16.2270953761477));
#8991=CARTESIAN_POINT('Ctrl Pts',(81.3316556913563,22.957199741655,-16.2256711156856));
#8992=CARTESIAN_POINT('Ctrl Pts',(81.3324687060016,22.9360136864517,-16.2242468552234));
#8993=CARTESIAN_POINT('Ctrl Pts',(81.3536148504745,22.3849739397882,-16.1872024825596));
#8994=CARTESIAN_POINT('Ctrl Pts',(81.6749048673942,21.8454544180445,-16.1501581098957));
#8995=CARTESIAN_POINT('Ctrl Pts',(82.1493177603708,21.564346170154,-16.1131137372319));
#8996=CARTESIAN_POINT('Ctrl Pts',(82.6237306533474,21.2832379222636,-16.076069364568));
#8997=CARTESIAN_POINT('Ctrl Pts',(83.2512664223808,21.2605409482263,-16.0390249919042));
#8998=CARTESIAN_POINT('Ctrl Pts',(83.744748519932,21.5066436861515,-16.0019806192403));
#8999=CARTESIAN_POINT('Ctrl Pts',(84.2382306174832,21.7527464240767,-15.9649362465765));
#9000=CARTESIAN_POINT('Ctrl Pts',(84.5976590435522,22.2676488739642,-15.9278918739126));
#9001=CARTESIAN_POINT('Ctrl Pts',(84.6585541971785,22.8157206109035,-15.8908475012488));
#9002=CARTESIAN_POINT('Ctrl Pts',(84.7194493508049,23.3637923478428,-15.8538031285849));
#9003=CARTESIAN_POINT('Ctrl Pts',(84.4818112319886,23.945033371834,-15.816758755921));
#9004=CARTESIAN_POINT('Ctrl Pts',(84.0543867577353,24.2934568182214,-15.7797143832572));
#9005=CARTESIAN_POINT('Ctrl Pts',(83.626962283482,24.6418802646089,-15.7426700105933));
#9006=CARTESIAN_POINT('Ctrl Pts',(83.0097514537917,24.7574861333928,-15.7056256379295));
#9007=CARTESIAN_POINT('Ctrl Pts',(82.4852025736897,24.5873706699448,-15.6685812652656));
#9008=CARTESIAN_POINT('Ctrl Pts',(81.9606536935877,24.4172552064967,-15.6315368926018));
#9009=CARTESIAN_POINT('Ctrl Pts',(81.528766763074,23.9614184108167,-15.5944925199379));
#9010=CARTESIAN_POINT('Ctrl Pts',(81.3871814989429,23.4284602887024,-15.5574481472741));
#9011=CARTESIAN_POINT('Ctrl Pts',(81.350326141176,23.289728603694,-15.547805310386));
#9012=CARTESIAN_POINT('Ctrl Pts',(81.3331412508702,23.1457712768177,-15.5381624734979));
#9013=CARTESIAN_POINT('Ctrl Pts',(81.3344264707835,23.0015125425552,-15.5285196366098));
#9014=CARTESIAN_POINT('Origin',(83.,23.,-12.));
#9015=CARTESIAN_POINT('',(81.3365468042549,22.999471848124,-14.8285196366098));
#9016=CARTESIAN_POINT('',(81.333366306688,22.9985354187012,-15.0214803633902));
#9017=CARTESIAN_POINT('',(81.334,23.,-12.));
#9018=CARTESIAN_POINT('Ctrl Pts',(81.333366306688,22.9985354187012,-15.0214803633902));
#9019=CARTESIAN_POINT('Ctrl Pts',(81.3374449915474,23.4429099901808,-15.0512325736413));
#9020=CARTESIAN_POINT('Ctrl Pts',(81.5206881913661,23.8902541505524,-15.0809847838924));
#9021=CARTESIAN_POINT('Ctrl Pts',(81.8387594834446,24.1984499635096,-15.1107369941435));
#9022=CARTESIAN_POINT('Ctrl Pts',(82.2347889339624,24.5821834895996,-15.1477813668074));
#9023=CARTESIAN_POINT('Ctrl Pts',(82.8398376944982,24.7502001641106,-15.1848257394712));
#9024=CARTESIAN_POINT('Ctrl Pts',(83.3770234781491,24.6256122398906,-15.2218701121351));
#9025=CARTESIAN_POINT('Ctrl Pts',(83.9142092618,24.5010243156706,-15.2589144847989));
#9026=CARTESIAN_POINT('Ctrl Pts',(84.3835320685661,24.0838317927196,-15.2959588574628));
#9027=CARTESIAN_POINT('Ctrl Pts',(84.5702206791894,23.5649502004703,-15.3330032301266));
#9028=CARTESIAN_POINT('Ctrl Pts',(84.7569092898127,23.0460686082211,-15.3700476027905));
#9029=CARTESIAN_POINT('Ctrl Pts',(84.6609637042931,22.4254979466735,-15.4070919754543));
#9030=CARTESIAN_POINT('Ctrl Pts',(84.3262902449012,21.9872235220564,-15.4441363481182));
#9031=CARTESIAN_POINT('Ctrl Pts',(83.9916167855093,21.5489490974392,-15.481180720782));
#9032=CARTESIAN_POINT('Ctrl Pts',(83.418215452245,21.2929709097526,-15.5182250934459));
#9033=CARTESIAN_POINT('Ctrl Pts',(82.8684865098548,21.3364296974664,-15.5552694661097));
#9034=CARTESIAN_POINT('Ctrl Pts',(82.3187575674646,21.3798884851801,-15.5923138387736));
#9035=CARTESIAN_POINT('Ctrl Pts',(81.7927010159485,21.722784248294,-15.6293582114374));
#9036=CARTESIAN_POINT('Ctrl Pts',(81.531049628514,22.20820097358,-15.6664025841013));
#9037=CARTESIAN_POINT('Ctrl Pts',(81.401374715867,22.4487744024699,-15.6847618438643));
#9038=CARTESIAN_POINT('Ctrl Pts',(81.3366433162294,22.7243540007479,-15.7031211036272));
#9039=CARTESIAN_POINT('Ctrl Pts',(81.3367022839223,22.9999597918218,-15.7214803633902));
#9040=CARTESIAN_POINT('Ctrl Pts',(81.3344264707835,23.0015125425552,-15.5285196366098));
#9041=CARTESIAN_POINT('Ctrl Pts',(81.3380786117293,22.5915801840872,-15.501118100834));
#9042=CARTESIAN_POINT('Ctrl Pts',(81.4908760810882,22.1792139742199,-15.4737165650583));
#9043=CARTESIAN_POINT('Ctrl Pts',(81.765275274686,21.8774062461374,-15.4463150292825));
#9044=CARTESIAN_POINT('Ctrl Pts',(82.1362379123091,21.4693897742355,-15.4092706566187));
#9045=CARTESIAN_POINT('Ctrl Pts',(82.7294467853039,21.2634362789804,-15.3722262839548));
#9046=CARTESIAN_POINT('Ctrl Pts',(83.2734377782961,21.3537941624193,-15.335181911291));
#9047=CARTESIAN_POINT('Ctrl Pts',(83.8174287712884,21.4441520458581,-15.2981375386271));
#9048=CARTESIAN_POINT('Ctrl Pts',(84.3122018842782,21.8308213079908,-15.2610931659633));
#9049=CARTESIAN_POINT('Ctrl Pts',(84.5313392342341,22.3368544701007,-15.2240487932994));
#9050=CARTESIAN_POINT('Ctrl Pts',(84.7504765841901,22.8428876322106,-15.1870044206355));
#9051=CARTESIAN_POINT('Ctrl Pts',(84.6939781711122,23.4682846942976,-15.1499600479717));
#9052=CARTESIAN_POINT('Ctrl Pts',(84.3876987654037,23.9268516604712,-15.1129156753078));
#9053=CARTESIAN_POINT('Ctrl Pts',(84.0814193596952,24.3854186266448,-15.075871302644));
#9054=CARTESIAN_POINT('Ctrl Pts',(83.5253589613561,24.677155496905,-15.0388269299801));
#9055=CARTESIAN_POINT('Ctrl Pts',(82.9739817594994,24.6685577343773,-15.0017825573163));
#9056=CARTESIAN_POINT('Ctrl Pts',(82.4226045576427,24.6599599718496,-14.9647381846524));
#9057=CARTESIAN_POINT('Ctrl Pts',(81.8759105522683,24.3510275765339,-14.9276938119886));
#9058=CARTESIAN_POINT('Ctrl Pts',(81.5840776752226,23.8831340941212,-14.8906494393247));
#9059=CARTESIAN_POINT('Ctrl Pts',(81.4209263176052,23.6215547352472,-14.8699395050864));
#9060=CARTESIAN_POINT('Ctrl Pts',(81.3374306038022,23.3102928382113,-14.8492295708481));
#9061=CARTESIAN_POINT('Ctrl Pts',(81.3365468042549,22.999471848124,-14.8285196366098));
#9062=CARTESIAN_POINT('Origin',(83.,23.,-12.));
#9063=CARTESIAN_POINT('',(81.3324917645664,22.9987669698696,-14.1285196366098));
#9064=CARTESIAN_POINT('',(81.3319380765938,23.0009590763004,-14.3214803633902));
#9065=CARTESIAN_POINT('',(81.334,23.,-12.));
#9066=CARTESIAN_POINT('Ctrl Pts',(81.3319380765938,23.0009590763004,-14.3214803633902));
#9067=CARTESIAN_POINT('Ctrl Pts',(81.3315519766315,23.0572154733417,-14.3252552983277));
#9068=CARTESIAN_POINT('Ctrl Pts',(81.3341512946454,23.1134357699009,-14.3290302332651));
#9069=CARTESIAN_POINT('Ctrl Pts',(81.3398536357379,23.1693395494696,-14.3328051682026));
#9070=CARTESIAN_POINT('Ctrl Pts',(81.3958121229659,23.7179372016065,-14.3698495408664));
#9071=CARTESIAN_POINT('Ctrl Pts',(81.7505912237274,24.2360543194683,-14.4068939135303));
#9072=CARTESIAN_POINT('Ctrl Pts',(82.2418370400616,24.4865903135586,-14.4439382861942));
#9073=CARTESIAN_POINT('Ctrl Pts',(82.7330828563959,24.7371263076488,-14.480982658858));
#9074=CARTESIAN_POINT('Ctrl Pts',(83.3607953883029,24.7200811779674,-14.5180270315219));
#9075=CARTESIAN_POINT('Ctrl Pts',(83.8377210268577,24.4432551111368,-14.5550714041857));
#9076=CARTESIAN_POINT('Ctrl Pts',(84.3146466654126,24.1664290443063,-14.5921157768496));
#9077=CARTESIAN_POINT('Ctrl Pts',(84.6407854106153,23.6298220403266,-14.6291601495134));
#9078=CARTESIAN_POINT('Ctrl Pts',(84.6668897564314,23.0789960248702,-14.6662045221773));
#9079=CARTESIAN_POINT('Ctrl Pts',(84.6929941022474,22.5281700094137,-14.7032488948411));
#9080=CARTESIAN_POINT('Ctrl Pts',(84.4190640486767,21.9631249824804,-14.740293267505));
#9081=CARTESIAN_POINT('Ctrl Pts',(83.9704553748996,21.642436667718,-14.7773376401688));
#9082=CARTESIAN_POINT('Ctrl Pts',(83.5218467011226,21.3217483529555,-14.8143820128327));
#9083=CARTESIAN_POINT('Ctrl Pts',(82.8985594071392,21.245416750364,-14.8514263854965));
#9084=CARTESIAN_POINT('Ctrl Pts',(82.385822033276,21.4483727047864,-14.8884707581604));
#9085=CARTESIAN_POINT('Ctrl Pts',(81.8730846594129,21.6513286592087,-14.9255151308242));
#9086=CARTESIAN_POINT('Ctrl Pts',(81.47089720567,22.1335721706451,-14.9625595034881));
#9087=CARTESIAN_POINT('Ctrl Pts',(81.3633085490485,22.6744191151978,-14.9996038761519));
#9088=CARTESIAN_POINT('Ctrl Pts',(81.3421297868928,22.7808845099802,-15.0068960385647));
#9089=CARTESIAN_POINT('Ctrl Pts',(81.33236663533,22.8896207693363,-15.0141882009774));
#9090=CARTESIAN_POINT('Ctrl Pts',(81.333366306688,22.9985354187012,-15.0214803633902));
#9091=CARTESIAN_POINT('Ctrl Pts',(81.3365468042549,22.999471848124,-14.8285196366098));
#9092=CARTESIAN_POINT('Ctrl Pts',(81.3358497296471,22.754319629603,-14.8121851981843));
#9093=CARTESIAN_POINT('Ctrl Pts',(81.3865444352782,22.5094416934687,-14.7958507597587));
#9094=CARTESIAN_POINT('Ctrl Pts',(81.4900814308096,22.2894313720426,-14.7795163213332));
#9095=CARTESIAN_POINT('Ctrl Pts',(81.7248898121595,21.7904767018865,-14.7424719486693));
#9096=CARTESIAN_POINT('Ctrl Pts',(82.2314783235764,21.419421931084,-14.7054275760055));
#9097=CARTESIAN_POINT('Ctrl Pts',(82.7780220917042,21.3460690255097,-14.6683832033416));
#9098=CARTESIAN_POINT('Ctrl Pts',(83.324565859832,21.2727161199355,-14.6313388306778));
#9099=CARTESIAN_POINT('Ctrl Pts',(83.9110648846709,21.4970650795895,-14.5942944580139));
#9100=CARTESIAN_POINT('Ctrl Pts',(84.2691256707508,21.9164494051546,-14.5572500853501));
#9101=CARTESIAN_POINT('Ctrl Pts',(84.6271864568307,22.3358337307197,-14.5202057126862));
#9102=CARTESIAN_POINT('Ctrl Pts',(84.7568090041518,22.9502534221959,-14.4831613400223));
#9103=CARTESIAN_POINT('Ctrl Pts',(84.59867548387,23.4785379372198,-14.4461169673585));
#9104=CARTESIAN_POINT('Ctrl Pts',(84.4405419635882,24.0068224522436,-14.4090725946946));
#9105=CARTESIAN_POINT('Ctrl Pts',(83.9946523757037,24.4489717908152,-14.3720282220308));
#9106=CARTESIAN_POINT('Ctrl Pts',(83.4650545707756,24.6026497141309,-14.3349838493669));
#9107=CARTESIAN_POINT('Ctrl Pts',(82.9354567658475,24.7563276374466,-14.2979394767031));
#9108=CARTESIAN_POINT('Ctrl Pts',(82.3221507438759,24.6215341455064,-14.2608951040392));
#9109=CARTESIAN_POINT('Ctrl Pts',(81.9057974101989,24.2599533929618,-14.2238507313754));
#9110=CARTESIAN_POINT('Ctrl Pts',(81.5486453764393,23.949785824471,-14.1920736997868));
#9111=CARTESIAN_POINT('Ctrl Pts',(81.3364185984152,23.4727395907271,-14.1602966681983));
#9112=CARTESIAN_POINT('Ctrl Pts',(81.3324917645664,22.9987669698696,-14.1285196366098));
#9113=CARTESIAN_POINT('Origin',(83.,23.,-12.));
#9114=CARTESIAN_POINT('',(81.3327117051948,23.0013103746205,-13.4285196366098));
#9115=CARTESIAN_POINT('',(81.3362661788622,23.0008554997906,-13.6214803633902));
#9116=CARTESIAN_POINT('',(81.334,23.,-12.));
#9117=CARTESIAN_POINT('Ctrl Pts',(81.3362661788622,23.0008554997906,-13.6214803633902));
#9118=CARTESIAN_POINT('Ctrl Pts',(81.335230124389,23.2235153031014,-13.6363223956779));
#9119=CARTESIAN_POINT('Ctrl Pts',(81.376782669324,23.4458042723491,-13.6511644279656));
#9120=CARTESIAN_POINT('Ctrl Pts',(81.4627523219824,23.6493315104454,-13.6660064602532));
#9121=CARTESIAN_POINT('Ctrl Pts',(81.6773248137497,24.157317122466,-13.7030508329171));
#9122=CARTESIAN_POINT('Ctrl Pts',(82.1685965800531,24.5484253044889,-13.740095205581));
#9123=CARTESIAN_POINT('Ctrl Pts',(82.7117519925065,24.6436772554877,-13.7771395782448));
#9124=CARTESIAN_POINT('Ctrl Pts',(83.2549074049598,24.7389292064865,-13.8141839509087));
#9125=CARTESIAN_POINT('Ctrl Pts',(83.8499464635632,24.5383249264613,-13.8512283235725));
#9126=CARTESIAN_POINT('Ctrl Pts',(84.2245675848282,24.1336648818027,-13.8882726962364));
#9127=CARTESIAN_POINT('Ctrl Pts',(84.5991887060932,23.729004837144,-13.9253170689002));
#9128=CARTESIAN_POINT('Ctrl Pts',(84.7533918900198,23.120289027852,-13.9623614415641));
#9129=CARTESIAN_POINT('Ctrl Pts',(84.6166107249878,22.5860777876742,-13.9994058142279));
#9130=CARTESIAN_POINT('Ctrl Pts',(84.4798295599558,22.0518665474965,-14.0364501868918));
#9131=CARTESIAN_POINT('Ctrl Pts',(84.0520640459651,21.592159876433,-14.0734945595556));
#9132=CARTESIAN_POINT('Ctrl Pts',(83.5290681004942,21.4173285940911,-14.1105389322195));
#9133=CARTESIAN_POINT('Ctrl Pts',(83.0060721550232,21.2424973117493,-14.1475833048833));
#9134=CARTESIAN_POINT('Ctrl Pts',(82.3878457780718,21.352541418129,-14.1846276775472));
#9135=CARTESIAN_POINT('Ctrl Pts',(81.9573015264435,21.6971025645249,-14.221672050211));
#9136=CARTESIAN_POINT('Ctrl Pts',(81.5706310516055,22.0065518756786,-14.2549414879374));
#9137=CARTESIAN_POINT('Ctrl Pts',(81.3353408713083,22.5051574985021,-14.2882109256638));
#9138=CARTESIAN_POINT('Ctrl Pts',(81.3319380765938,23.0009590763004,-14.3214803633902));
#9139=CARTESIAN_POINT('Ctrl Pts',(81.3324917645664,22.9987669698696,-14.1285196366098));
#9140=CARTESIAN_POINT('Ctrl Pts',(81.3318408550197,22.9202015617864,-14.1232522955345));
#9141=CARTESIAN_POINT('Ctrl Pts',(81.3369132306244,22.8417206048205,-14.1179849544591));
#9142=CARTESIAN_POINT('Ctrl Pts',(81.3479975271719,22.7640981352866,-14.1127176133838));
#9143=CARTESIAN_POINT('Ctrl Pts',(81.4259516232043,22.218191643305,-14.07567324072));
#9144=CARTESIAN_POINT('Ctrl Pts',(81.8012604606514,21.7147466724909,-14.0386288680561));
#9145=CARTESIAN_POINT('Ctrl Pts',(82.3021753294762,21.4841495491966,-14.0015844953923));
#9146=CARTESIAN_POINT('Ctrl Pts',(82.803090198301,21.2535524259023,-13.9645401227284));
#9147=CARTESIAN_POINT('Ctrl Pts',(83.4296110985035,21.295803150128,-13.9274957500645));
#9148=CARTESIAN_POINT('Ctrl Pts',(83.8950297363476,21.5915669589779,-13.8904513774007));
#9149=CARTESIAN_POINT('Ctrl Pts',(84.3604483741916,21.887330767828,-13.8534070047368));
#9150=CARTESIAN_POINT('Ctrl Pts',(84.6647647496773,22.4366076613023,-13.816362632073));
#9151=CARTESIAN_POINT('Ctrl Pts',(84.6687177004905,22.9880377232852,-13.7793182594091));
#9152=CARTESIAN_POINT('Ctrl Pts',(84.6726706513036,23.539467785268,-13.7422738867453));
#9153=CARTESIAN_POINT('Ctrl Pts',(84.3762601774443,24.0930510157592,-13.7052295140814));
#9154=CARTESIAN_POINT('Ctrl Pts',(83.9151295450538,24.3954568340733,-13.6681851414176));
#9155=CARTESIAN_POINT('Ctrl Pts',(83.4539989126633,24.6978626523874,-13.6311407687537));
#9156=CARTESIAN_POINT('Ctrl Pts',(82.8281481217416,24.7490910585245,-13.5940963960899));
#9157=CARTESIAN_POINT('Ctrl Pts',(82.323978810837,24.5256989256713,-13.557052023426));
#9158=CARTESIAN_POINT('Ctrl Pts',(81.8198094999325,24.3023067928182,-13.5200076507622));
#9159=CARTESIAN_POINT('Ctrl Pts',(81.437321669045,23.804294120975,-13.4829632780983));
#9160=CARTESIAN_POINT('Ctrl Pts',(81.3515492768764,23.2595613095707,-13.4459189054345));
#9161=CARTESIAN_POINT('Ctrl Pts',(81.3381205444153,23.1742766276097,-13.4401191491596));
#9162=CARTESIAN_POINT('Ctrl Pts',(81.3319648379856,23.0878467514766,-13.4343193928847));
#9163=CARTESIAN_POINT('Ctrl Pts',(81.3327117051948,23.0013103746205,-13.4285196366098));
#9164=CARTESIAN_POINT('Origin',(83.,23.,-12.));
#9165=CARTESIAN_POINT('',(81.3366135456033,23.0004031163987,-12.7285196366098));
#9166=CARTESIAN_POINT('',(81.3350588241434,22.9985780810801,-12.9214803633902));
#9167=CARTESIAN_POINT('',(81.334,23.,-12.));
#9168=CARTESIAN_POINT('Ctrl Pts',(81.3350588241434,22.9985780810801,-12.9214803633902));
#9169=CARTESIAN_POINT('Ctrl Pts',(81.338211023598,23.3865574103556,-12.9473894930281));
#9170=CARTESIAN_POINT('Ctrl Pts',(81.4733906618918,23.7765167665672,-12.973298622666));
#9171=CARTESIAN_POINT('Ctrl Pts',(81.7211702184837,24.0720803253201,-12.9992077523039));
#9172=CARTESIAN_POINT('Ctrl Pts',(82.0754406382609,24.4946713875952,-13.0362521249677));
#9173=CARTESIAN_POINT('Ctrl Pts',(82.6598960034212,24.7242916927789,-13.0732964976316));
#9174=CARTESIAN_POINT('Ctrl Pts',(83.2070780368979,24.6558624703356,-13.1103408702954));
#9175=CARTESIAN_POINT('Ctrl Pts',(83.7542600703746,24.5874332478923,-13.1473852429593));
#9176=CARTESIAN_POINT('Ctrl Pts',(84.2641687721677,24.2209544978219,-13.1844296156232));
#9177=CARTESIAN_POINT('Ctrl Pts',(84.503459885431,23.7241341083882,-13.221473988287));
#9178=CARTESIAN_POINT('Ctrl Pts',(84.7427509986944,23.2273137189545,-13.2585183609509));
#9179=CARTESIAN_POINT('Ctrl Pts',(84.7114245234279,22.6001516901575,-13.2955627336147));
#9180=CARTESIAN_POINT('Ctrl Pts',(84.4238160712131,22.1296497088031,-13.3326071062786));
#9181=CARTESIAN_POINT('Ctrl Pts',(84.1362076189983,21.6591477274488,-13.3696514789424));
#9182=CARTESIAN_POINT('Ctrl Pts',(83.5923171898351,21.3453057935372,-13.4066958516063));
#9183=CARTESIAN_POINT('Ctrl Pts',(83.0410397477669,21.3317441523751,-13.4437402242701));
#9184=CARTESIAN_POINT('Ctrl Pts',(82.4897623056988,21.3181825112131,-13.480784596934));
#9185=CARTESIAN_POINT('Ctrl Pts',(81.9310978507256,21.6049011628006,-13.5178289695978));
#9186=CARTESIAN_POINT('Ctrl Pts',(81.6207022318547,22.0606920096035,-13.5548733422617));
#9187=CARTESIAN_POINT('Ctrl Pts',(81.4346683301881,22.3338677389618,-13.5770756826379));
#9188=CARTESIAN_POINT('Ctrl Pts',(81.3378160228199,22.6677765355771,-13.599278023014));
#9189=CARTESIAN_POINT('Ctrl Pts',(81.3362661788622,23.0008554997906,-13.6214803633902));
#9190=CARTESIAN_POINT('Ctrl Pts',(81.3327117051948,23.0013103746205,-13.4285196366098));
#9191=CARTESIAN_POINT('Ctrl Pts',(81.3367352500372,22.5351190778817,-13.3972750202208));
#9192=CARTESIAN_POINT('Ctrl Pts',(81.5410869333838,22.0658368917593,-13.3660304038319));
#9193=CARTESIAN_POINT('Ctrl Pts',(81.8878467271069,21.7558629667172,-13.3347857874429));
#9194=CARTESIAN_POINT('Ctrl Pts',(82.2989735229558,21.3883503862333,-13.297741414779));
#9195=CARTESIAN_POINT('Ctrl Pts',(82.9102840681031,21.244778176231,-13.2606970421152));
#9196=CARTESIAN_POINT('Ctrl Pts',(83.4420306266154,21.3908478054807,-13.2236526694514));
#9197=CARTESIAN_POINT('Ctrl Pts',(83.9737771851276,21.5369174347303,-13.1866082967875));
#9198=CARTESIAN_POINT('Ctrl Pts',(84.4259597570048,21.9726289032321,-13.1495639241236));
#9199=CARTESIAN_POINT('Ctrl Pts',(84.5916506984895,22.4985920682814,-13.1125195514598));
#9200=CARTESIAN_POINT('Ctrl Pts',(84.7573416399743,23.0245552333307,-13.0754751787959));
#9201=CARTESIAN_POINT('Ctrl Pts',(84.6365409510666,23.6407700949276,-13.0384308061321));
#9202=CARTESIAN_POINT('Ctrl Pts',(84.284529404345,24.0652446054149,-13.0013864334682));
#9203=CARTESIAN_POINT('Ctrl Pts',(83.9325178576235,24.4897191159023,-12.9643420608044));
#9204=CARTESIAN_POINT('Ctrl Pts',(83.349295453088,24.7224532752801,-12.9272976881405));
#9205=CARTESIAN_POINT('Ctrl Pts',(82.8017562407592,24.6569433520536,-12.8902533154767));
#9206=CARTESIAN_POINT('Ctrl Pts',(82.2542170284304,24.591433428827,-12.8532089428128));
#9207=CARTESIAN_POINT('Ctrl Pts',(81.7423610083083,24.2276794229961,-12.8161645701489));
#9208=CARTESIAN_POINT('Ctrl Pts',(81.500423568429,23.732142326238,-12.7791201974851));
#9209=CARTESIAN_POINT('Ctrl Pts',(81.390265855086,23.506516918766,-12.76225334386));
#9210=CARTESIAN_POINT('Ctrl Pts',(81.3360654021539,23.2535713441157,-12.7453864902349));
#9211=CARTESIAN_POINT('Ctrl Pts',(81.3366135456033,23.0004031163987,-12.7285196366098));
#9212=CARTESIAN_POINT('Origin',(83.,23.,-12.));
#9213=CARTESIAN_POINT('',(81.3341896407369,22.9984774011262,-12.0285196366098));
#9214=CARTESIAN_POINT('',(81.3312396011681,22.9999810457179,-12.2214803633902));
#9215=CARTESIAN_POINT('',(81.334,23.,-12.));
#9216=CARTESIAN_POINT('Ctrl Pts',(81.3312397054754,22.9999810464341,-12.2214803633902));
#9217=CARTESIAN_POINT('Ctrl Pts',(81.3313322642857,23.5504110986567,-12.2584565903783));
#9218=CARTESIAN_POINT('Ctrl Pts',(81.6304402888706,24.100927338771,-12.2954328173664));
#9219=CARTESIAN_POINT('Ctrl Pts',(82.0923259674676,24.4003177084854,-12.3324090443545));
#9220=CARTESIAN_POINT('Ctrl Pts',(82.5550628825009,24.7002598424202,-12.3694534170184));
#9221=CARTESIAN_POINT('Ctrl Pts',(83.1811779895532,24.7481496235668,-12.4064977896822));
#9222=CARTESIAN_POINT('Ctrl Pts',(83.6841486938121,24.5220717456108,-12.4435421623461));
#9223=CARTESIAN_POINT('Ctrl Pts',(84.1871193980711,24.2959938676547,-12.4805865350099));
#9224=CARTESIAN_POINT('Ctrl Pts',(84.5669456995367,23.795948330596,-12.5176309076738));
#9225=CARTESIAN_POINT('Ctrl Pts',(84.6498116077496,23.250765812993,-12.5546752803376));
#9226=CARTESIAN_POINT('Ctrl Pts',(84.7326775159625,22.70558329539,-12.5917196530015));
#9227=CARTESIAN_POINT('Ctrl Pts',(84.5185830309226,22.1152637972427,-12.6287640256654));
#9228=CARTESIAN_POINT('Ctrl Pts',(84.1055020023226,21.7499491382778,-12.6658083983292));
#9229=CARTESIAN_POINT('Ctrl Pts',(83.6924209737225,21.384634479313,-12.7028527709931));
#9230=CARTESIAN_POINT('Ctrl Pts',(83.0803534015624,21.2443246595305,-12.7398971436569));
#9231=CARTESIAN_POINT('Ctrl Pts',(82.5493934522351,21.3932282137333,-12.7769415163208));
#9232=CARTESIAN_POINT('Ctrl Pts',(82.0184335029077,21.542131767936,-12.8139858889846));
#9233=CARTESIAN_POINT('Ctrl Pts',(81.5685811764133,21.980248696124,-12.8510302616485));
#9234=CARTESIAN_POINT('Ctrl Pts',(81.405697750363,22.5070880699012,-12.8880746343123));
#9235=CARTESIAN_POINT('Ctrl Pts',(81.3567362913465,22.6654517845709,-12.8992098773383));
#9236=CARTESIAN_POINT('Ctrl Pts',(81.3337040697582,22.83183206603,-12.9103451203643));
#9237=CARTESIAN_POINT('Ctrl Pts',(81.3350588241434,22.9985780810801,-12.9214803633902));
#9238=CARTESIAN_POINT('Ctrl Pts',(81.3366135456033,23.0004031163987,-12.7285196366098));
#9239=CARTESIAN_POINT('Ctrl Pts',(81.3372692799288,22.6975424377975,-12.708342117571));
#9240=CARTESIAN_POINT('Ctrl Pts',(81.4162752610685,22.3943631223019,-12.6881645985323));
#9241=CARTESIAN_POINT('Ctrl Pts',(81.5715622690257,22.1372558266083,-12.6679870794936));
#9242=CARTESIAN_POINT('Ctrl Pts',(81.8566572691383,21.6652266114217,-12.6309427068297));
#9243=CARTESIAN_POINT('Ctrl Pts',(82.3988661289997,21.3484883687338,-12.5938983341658));
#9244=CARTESIAN_POINT('Ctrl Pts',(82.9500634037713,21.3319867517464,-12.556853961502));
#9245=CARTESIAN_POINT('Ctrl Pts',(83.5012606785428,21.315485134759,-12.5198095888381));
#9246=CARTESIAN_POINT('Ctrl Pts',(84.0614463682244,21.599220143472,-12.4827652161743));
#9247=CARTESIAN_POINT('Ctrl Pts',(84.3742684768708,22.0533490540479,-12.4457208435104));
#9248=CARTESIAN_POINT('Ctrl Pts',(84.687090585517,22.5074779646238,-12.4086764708466));
#9249=CARTESIAN_POINT('Ctrl Pts',(84.7525491131281,23.1320007770625,-12.3716320981827));
#9250=CARTESIAN_POINT('Ctrl Pts',(84.5406889492579,23.6411235619029,-12.3345877255189));
#9251=CARTESIAN_POINT('Ctrl Pts',(84.3288287853876,24.1502463467433,-12.297543352855));
#9252=CARTESIAN_POINT('Ctrl Pts',(83.8396499300361,24.5439691039855,-12.2604989801912));
#9253=CARTESIAN_POINT('Ctrl Pts',(83.2970102543581,24.6421165515269,-12.2234546075273));
#9254=CARTESIAN_POINT('Ctrl Pts',(82.7543705786802,24.7402639990683,-12.1864102348635));
#9255=CARTESIAN_POINT('Ctrl Pts',(82.1582700826758,24.5428361369091,-12.1493658621996));
#9256=CARTESIAN_POINT('Ctrl Pts',(81.7814960844601,24.1401798401158,-12.1123214895357));
#9257=CARTESIAN_POINT('Ctrl Pts',(81.4973831237566,23.8365498837768,-12.0843875385604));
#9258=CARTESIAN_POINT('Ctrl Pts',(81.3379830543993,23.4162234419347,-12.0564535875851));
#9259=CARTESIAN_POINT('Ctrl Pts',(81.3341896407369,22.9984774011262,-12.0285196366098));
#9260=CARTESIAN_POINT('Origin',(83.,23.,-12.));
#9261=CARTESIAN_POINT('',(81.3314456081428,23.0005306221462,-11.3285196366098));
#9262=CARTESIAN_POINT('',(81.335003566498,23.0014338851118,-11.5214803633902));
#9263=CARTESIAN_POINT('',(81.334,23.,-12.));
#9264=CARTESIAN_POINT('Ctrl Pts',(81.335003566498,23.0014338851118,-11.5214803633902));
#9265=CARTESIAN_POINT('Ctrl Pts',(81.3336508586925,23.1661251583794,-11.5324793150647));
#9266=CARTESIAN_POINT('Ctrl Pts',(81.3561117067033,23.3304556252146,-11.5434782667392));
#9267=CARTESIAN_POINT('Ctrl Pts',(81.4038994824931,23.4870574627757,-11.5544772184136));
#9268=CARTESIAN_POINT('Ctrl Pts',(81.5648482917547,24.0144910766468,-11.5915215910775));
#9269=CARTESIAN_POINT('Ctrl Pts',(82.0130896834685,24.4542560288336,-11.6285659637413));
#9270=CARTESIAN_POINT('Ctrl Pts',(82.5434995754815,24.6051072227256,-11.6656103364052));
#9271=CARTESIAN_POINT('Ctrl Pts',(83.0739094674945,24.7559584166175,-11.702654709069));
#9272=CARTESIAN_POINT('Ctrl Pts',(83.6864878598067,24.6178958522146,-11.7396990817329));
#9273=CARTESIAN_POINT('Ctrl Pts',(84.1009068246708,24.2540996760324,-11.7767434543967));
#9274=CARTESIAN_POINT('Ctrl Pts',(84.515325789535,23.8903034998501,-11.8137878270606));
#9275=CARTESIAN_POINT('Ctrl Pts',(84.731585326951,23.3007737118886,-11.8508321997244));
#9276=CARTESIAN_POINT('Ctrl Pts',(84.6507208166511,22.7552907449521,-11.8878765723883));
#9277=CARTESIAN_POINT('Ctrl Pts',(84.5698563063513,22.2098077780156,-11.9249209450521));
#9278=CARTESIAN_POINT('Ctrl Pts',(84.1918677483354,21.7083716321042,-11.961965317716));
#9279=CARTESIAN_POINT('Ctrl Pts',(83.689730145494,21.4804493557541,-11.9990096903798));
#9280=CARTESIAN_POINT('Ctrl Pts',(83.1875925426527,21.2525270794039,-12.0360540630437));
#9281=CARTESIAN_POINT('Ctrl Pts',(82.5613058949858,21.2981186726152,-12.0730984357076));
#9282=CARTESIAN_POINT('Ctrl Pts',(82.0974712976668,21.5963605251005,-12.1101428083714));
#9283=CARTESIAN_POINT('Ctrl Pts',(81.6327834446495,21.8951510140213,-12.147255326711));
#9284=CARTESIAN_POINT('Ctrl Pts',(81.3311468055007,22.4475221540126,-12.1843678450506));
#9285=CARTESIAN_POINT('Ctrl Pts',(81.3312397054754,22.9999810464341,-12.2214803633902));
#9286=CARTESIAN_POINT('Ctrl Pts',(81.3341896407369,22.9984774011262,-12.0285196366098));
#9287=CARTESIAN_POINT('Ctrl Pts',(81.3329524509769,22.8622330655561,-12.0194092149213));
#9288=CARTESIAN_POINT('Ctrl Pts',(81.3482668769255,22.7262632028618,-12.0102987932327));
#9289=CARTESIAN_POINT('Ctrl Pts',(81.381204657911,22.5947056619895,-12.0011883715442));
#9290=CARTESIAN_POINT('Ctrl Pts',(81.5151347300046,22.0597725120841,-11.9641439988803));
#9291=CARTESIAN_POINT('Ctrl Pts',(81.9404423746189,21.5977909437006,-11.9270996262165));
#9292=CARTESIAN_POINT('Ctrl Pts',(82.4624984436055,21.4201728142401,-11.8900552535526));
#9293=CARTESIAN_POINT('Ctrl Pts',(82.9845545125921,21.2425546847796,-11.8530108808888));
#9294=CARTESIAN_POINT('Ctrl Pts',(83.603359005951,21.3492999942421,-11.8159665082249));
#9295=CARTESIAN_POINT('Ctrl Pts',(84.0357348095674,21.6915599882903,-11.7789221355611));
#9296=CARTESIAN_POINT('Ctrl Pts',(84.4681106131838,22.0338199823385,-11.7418777628972));
#9297=CARTESIAN_POINT('Ctrl Pts',(84.7140577270577,22.6115946609723,-11.7048333902334));
#9298=CARTESIAN_POINT('Ctrl Pts',(84.6610259116884,23.1604829607542,-11.6677890175695));
#9299=CARTESIAN_POINT('Ctrl Pts',(84.607994096319,23.709371260536,-11.6307446449057));
#9300=CARTESIAN_POINT('Ctrl Pts',(84.2559833517065,24.2293731814658,-11.5937002722418));
#9301=CARTESIAN_POINT('Ctrl Pts',(83.7660807220893,24.4825256109881,-11.5566558995779));
#9302=CARTESIAN_POINT('Ctrl Pts',(83.2761780924722,24.7356780405103,-11.5196115269141));
#9303=CARTESIAN_POINT('Ctrl Pts',(82.6483835778505,24.7219809786249,-11.4825671542502));
#9304=CARTESIAN_POINT('Ctrl Pts',(82.1699883029908,24.4477024704062,-11.4455227815864));
#9305=CARTESIAN_POINT('Ctrl Pts',(81.6915930281311,24.1734239621876,-11.4084784089225));
#9306=CARTESIAN_POINT('Ctrl Pts',(81.3625969930333,23.6385640076356,-11.3714340362587));
#9307=CARTESIAN_POINT('Ctrl Pts',(81.3335552579371,23.0878850478946,-11.3343896635948));
#9308=CARTESIAN_POINT('Ctrl Pts',(81.3320212798414,23.0587983056868,-11.3324329879332));
#9309=CARTESIAN_POINT('Ctrl Pts',(81.3313241530342,23.029667429573,-11.3304763122715));
#9310=CARTESIAN_POINT('Ctrl Pts',(81.3314456081428,23.0005306221462,-11.3285196366098));
#9311=CARTESIAN_POINT('Origin',(83.,23.,-12.));
#9312=CARTESIAN_POINT('',(81.3357537722937,23.0011866319928,-10.6285196366098));
#9313=CARTESIAN_POINT('',(81.3362973248117,22.9991726428529,-10.8214803633902));
#9314=CARTESIAN_POINT('',(81.334,23.,-12.));
#9315=CARTESIAN_POINT('Ctrl Pts',(81.3362973248117,22.9991726428529,-10.8214803633902));
#9316=CARTESIAN_POINT('Ctrl Pts',(81.3377853361398,23.3302224779932,-10.8435464124149));
#9317=CARTESIAN_POINT('Ctrl Pts',(81.4333699684559,23.6620640474109,-10.8656124614396));
#9318=CARTESIAN_POINT('Ctrl Pts',(81.6172642260941,23.9342395911072,-10.8876785104643));
#9319=CARTESIAN_POINT('Ctrl Pts',(81.9259849854412,24.391166531648,-10.9247228831281));
#9320=CARTESIAN_POINT('Ctrl Pts',(82.4835934100557,24.6799335713466,-10.961767255792));
#9321=CARTESIAN_POINT('Ctrl Pts',(83.0349169112071,24.668395229957,-10.9988116284558));
#9322=CARTESIAN_POINT('Ctrl Pts',(83.5862404123585,24.6568568885673,-11.0358560011197));
#9323=CARTESIAN_POINT('Ctrl Pts',(84.1312789900469,24.3450131660894,-11.0729003737835));
#9324=CARTESIAN_POINT('Ctrl Pts',(84.4206122648672,23.8755698869538,-11.1099447464474));
#9325=CARTESIAN_POINT('Ctrl Pts',(84.7099455396876,23.4061266078182,-11.1469891191112));
#9326=CARTESIAN_POINT('Ctrl Pts',(84.74357351164,22.7790837720248,-11.1840334917751));
#9327=CARTESIAN_POINT('Ctrl Pts',(84.5061073589669,22.2813885213156,-11.2210778644389));
#9328=CARTESIAN_POINT('Ctrl Pts',(84.2686412062939,21.7836932706063,-11.2581222371028));
#9329=CARTESIAN_POINT('Ctrl Pts',(83.7600809289955,21.4153456049811,-11.2951666097666));
#9330=CARTESIAN_POINT('Ctrl Pts',(83.2131537183322,21.3449086652415,-11.3322109824305));
#9331=CARTESIAN_POINT('Ctrl Pts',(82.6662265076688,21.2744717255019,-11.3692553550943));
#9332=CARTESIAN_POINT('Ctrl Pts',(82.0809323636405,21.5019455116479,-11.4062997277582));
#9333=CARTESIAN_POINT('Ctrl Pts',(81.7251134050312,21.9232335424986,-11.4433441004221));
#9334=CARTESIAN_POINT('Ctrl Pts',(81.4749416810535,22.2194357273989,-11.4693895214114));
#9335=CARTESIAN_POINT('Ctrl Pts',(81.3382067667041,22.6114463960778,-11.4954349424008));
#9336=CARTESIAN_POINT('Ctrl Pts',(81.335003566498,23.0014338851118,-11.5214803633902));
#9337=CARTESIAN_POINT('Ctrl Pts',(81.3314456081428,23.0005306221462,-11.3285196366098));
#9338=CARTESIAN_POINT('Ctrl Pts',(81.3336235777125,22.4780406200363,-11.2934319396076));
#9339=CARTESIAN_POINT('Ctrl Pts',(81.5990308224674,21.953643300933,-11.2583442426054));
#9340=CARTESIAN_POINT('Ctrl Pts',(82.0223180314453,21.6476317704281,-11.2232565456033));
#9341=CARTESIAN_POINT('Ctrl Pts',(82.4692099751442,21.3245554176324,-11.1862121729394));
#9342=CARTESIAN_POINT('Ctrl Pts',(83.0920812976368,21.244900676971,-11.1491678002756));
#9343=CARTESIAN_POINT('Ctrl Pts',(83.605893823762,21.4451191253606,-11.1121234276117));
#9344=CARTESIAN_POINT('Ctrl Pts',(84.1197063498873,21.6453375737501,-11.0750790549479));
#9345=CARTESIAN_POINT('Ctrl Pts',(84.5244600796454,22.1254292111906,-11.038034682284));
#9346=CARTESIAN_POINT('Ctrl Pts',(84.6349317408232,22.6656946562779,-11.0009903096202));
#9347=CARTESIAN_POINT('Ctrl Pts',(84.745403402001,23.2059601013652,-10.9639459369563));
#9348=CARTESIAN_POINT('Ctrl Pts',(84.5615929945986,23.8063993540994,-10.9269015642925));
#9349=CARTESIAN_POINT('Ctrl Pts',(84.1676157783968,24.1922395958998,-10.8898571916286));
#9350=CARTESIAN_POINT('Ctrl Pts',(83.7736385621949,24.5780798377003,-10.8528128189648));
#9351=CARTESIAN_POINT('Ctrl Pts',(83.1694945371938,24.7493210685671,-10.8157684463009));
#9352=CARTESIAN_POINT('Ctrl Pts',(82.6316518986724,24.627599931261,-10.778724073637));
#9353=CARTESIAN_POINT('Ctrl Pts',(82.093809260151,24.5058787939549,-10.7416797009732));
#9354=CARTESIAN_POINT('Ctrl Pts',(81.6222680081092,24.0911952884759,-10.7046353283093));
#9355=CARTESIAN_POINT('Ctrl Pts',(81.432814699323,23.573316747823,-10.6675909556455));
#9356=CARTESIAN_POINT('Ctrl Pts',(81.3662081755097,23.3912450301455,-10.6545671826336));
#9357=CARTESIAN_POINT('Ctrl Pts',(81.3344685786651,23.1964180925411,-10.6415434096217));
#9358=CARTESIAN_POINT('Ctrl Pts',(81.3357537722937,23.0011866319928,-10.6285196366098));
#9359=CARTESIAN_POINT('Origin',(83.,23.,-12.));
#9360=CARTESIAN_POINT('',(81.3357306082006,22.9988024506805,-9.92851963660979));
#9361=CARTESIAN_POINT('',(81.3319839553715,22.9990126570311,-10.1214803633902));
#9362=CARTESIAN_POINT('',(81.334,23.,-12.));
#9363=CARTESIAN_POINT('Ctrl Pts',(81.3319839553715,22.9990126570311,-10.1214803633902));
#9364=CARTESIAN_POINT('Ctrl Pts',(81.3354513145775,23.4928188600527,-10.1546135097651));
#9365=CARTESIAN_POINT('Ctrl Pts',(81.568574055279,23.9894690902029,-10.18774665614));
#9366=CARTESIAN_POINT('Ctrl Pts',(81.9525268672513,24.2990619193099,-10.2208798025149));
#9367=CARTESIAN_POINT('Ctrl Pts',(82.3818036673203,24.6452008584172,-10.2579241751788));
#9368=CARTESIAN_POINT('Ctrl Pts',(82.9996220147768,24.757513137192,-10.2949685478426));
#9369=CARTESIAN_POINT('Ctrl Pts',(83.5232560752779,24.5846024465828,-10.3320129205065));
#9370=CARTESIAN_POINT('Ctrl Pts',(84.0468901357791,24.4116917559736,-10.3690572931703));
#9371=CARTESIAN_POINT('Ctrl Pts',(84.476339909325,23.9535580959804,-10.4061016658342));
#9372=CARTESIAN_POINT('Ctrl Pts',(84.6150807280518,23.4198524453986,-10.443146038498));
#9373=CARTESIAN_POINT('Ctrl Pts',(84.7538215467786,22.8861467948169,-10.4801904111619));
#9374=CARTESIAN_POINT('Ctrl Pts',(84.6018534106864,22.2768691536466,-10.5172347838257));
#9375=CARTESIAN_POINT('Ctrl Pts',(84.2287199295546,21.8708369609544,-10.5542791564896));
#9376=CARTESIAN_POINT('Ctrl Pts',(83.8555864484229,21.4648047682622,-10.5913235291534));
#9377=CARTESIAN_POINT('Ctrl Pts',(83.2612876222518,21.2620180240482,-10.6283679018173));
#9378=CARTESIAN_POINT('Ctrl Pts',(82.717786289584,21.3552759332688,-10.6654122744811));
#9379=CARTESIAN_POINT('Ctrl Pts',(82.1742849569162,21.4485338424895,-10.702456647145));
#9380=CARTESIAN_POINT('Ctrl Pts',(81.6815811177517,21.8378364051449,-10.7395010198088));
#9381=CARTESIAN_POINT('Ctrl Pts',(81.4651457452094,22.3450311071641,-10.7765453924727));
#9382=CARTESIAN_POINT('Ctrl Pts',(81.3776334235319,22.5501075020015,-10.7915237161119));
#9383=CARTESIAN_POINT('Ctrl Pts',(81.3352872701694,22.7744576716372,-10.806502039751));
#9384=CARTESIAN_POINT('Ctrl Pts',(81.3362973248117,22.9991726428529,-10.8214803633902));
#9385=CARTESIAN_POINT('Ctrl Pts',(81.3357537722937,23.0011866319928,-10.6285196366098));
#9386=CARTESIAN_POINT('Ctrl Pts',(81.3381241392834,22.6411084312276,-10.6044990369578));
#9387=CARTESIAN_POINT('Ctrl Pts',(81.4528344298303,22.2796541709646,-10.5804784373059));
#9388=CARTESIAN_POINT('Ctrl Pts',(81.6683271709657,21.9943115112502,-10.5564578376539));
#9389=CARTESIAN_POINT('Ctrl Pts',(82.0006583169253,21.5542583911568,-10.5194134649901));
#9390=CARTESIAN_POINT('Ctrl Pts',(82.5726859743754,21.2952257267967,-10.4823690923262));
#9391=CARTESIAN_POINT('Ctrl Pts',(83.1226390298723,21.3357519630943,-10.4453247196624));
#9392=CARTESIAN_POINT('Ctrl Pts',(83.6725920853691,21.3762781993919,-10.4082803469985));
#9393=CARTESIAN_POINT('Ctrl Pts',(84.2004705389127,21.7163633363471,-10.3712359743347));
#9394=CARTESIAN_POINT('Ctrl Pts',(84.4647068216147,22.200377722479,-10.3341916016708));
#9395=CARTESIAN_POINT('Ctrl Pts',(84.7289431043167,22.6843921086108,-10.297147229007));
#9396=CARTESIAN_POINT('Ctrl Pts',(84.7295372161771,23.3123357439193,-10.2601028563431));
#9397=CARTESIAN_POINT('Ctrl Pts',(84.4662172799166,23.796849263077,-10.2230584836792));
#9398=CARTESIAN_POINT('Ctrl Pts',(84.2028973436561,24.2813627822347,-10.1860141110154));
#9399=CARTESIAN_POINT('Ctrl Pts',(83.6756633592748,24.6224461852415,-10.1489697383515));
#9400=CARTESIAN_POINT('Ctrl Pts',(83.1257879738892,24.6640129944256,-10.1119253656877));
#9401=CARTESIAN_POINT('Ctrl Pts',(82.5759125885035,24.7055798036097,-10.0748809930238));
#9402=CARTESIAN_POINT('Ctrl Pts',(82.0033958021135,24.4476300189711,-10.03783662036));
#9403=CARTESIAN_POINT('Ctrl Pts',(81.6702325631919,24.0082065383626,-10.0007922476961));
#9404=CARTESIAN_POINT('Ctrl Pts',(81.4535682813828,23.7224385972649,-9.97670137733401));
#9405=CARTESIAN_POINT('Ctrl Pts',(81.3381319306509,23.3599213997545,-9.9526105069719));
#9406=CARTESIAN_POINT('Ctrl Pts',(81.3357306082006,22.9988024506805,-9.92851963660979));
#9407=CARTESIAN_POINT('Origin',(83.,23.,-12.));
#9408=CARTESIAN_POINT('',(81.3314317338341,22.9994875421002,-9.22851963660979));
#9409=CARTESIAN_POINT('',(81.3333049749392,23.0014544405517,-9.42148036339021));
#9410=CARTESIAN_POINT('',(81.334,23.,-12.));
#9411=CARTESIAN_POINT('Ctrl Pts',(81.3333049749392,23.0014544405517,-9.42148036339021));
#9412=CARTESIAN_POINT('Ctrl Pts',(81.3323267877789,23.1083233317145,-9.42863623445147));
#9413=CARTESIAN_POINT('Ctrl Pts',(81.34172531431,23.2150208601815,-9.43579210551273));
#9414=CARTESIAN_POINT('Ctrl Pts',(81.362124673025,23.3195719751752,-9.44294797657399));
#9415=CARTESIAN_POINT('Ctrl Pts',(81.4677276722785,23.8608101323596,-9.47999234923784));
#9416=CARTESIAN_POINT('Ctrl Pts',(81.8681425754562,24.3445264373676,-9.5170367219017));
#9417=CARTESIAN_POINT('Ctrl Pts',(82.380131642776,24.5493627895829,-9.55408109456555));
#9418=CARTESIAN_POINT('Ctrl Pts',(82.8921207100958,24.7541991417982,-9.5911254672294));
#9419=CARTESIAN_POINT('Ctrl Pts',(83.5156839415576,24.6801555412208,-9.62816983989325));
#9420=CARTESIAN_POINT('Ctrl Pts',(83.9654665308395,24.361115796639,-9.66521421255711));
#9421=CARTESIAN_POINT('Ctrl Pts',(84.4152491201214,24.0420760520572,-9.70225858522096));
#9422=CARTESIAN_POINT('Ctrl Pts',(84.6912510672232,23.478040163471,-9.73930295788482));
#9423=CARTESIAN_POINT('Ctrl Pts',(84.6671684494862,22.9271220536155,-9.77634733054867));
#9424=CARTESIAN_POINT('Ctrl Pts',(84.643085831749,22.37620394376,-9.81339170321253));
#9425=CARTESIAN_POINT('Ctrl Pts',(84.318918649173,21.8384036126351,-9.85043607587637));
#9426=CARTESIAN_POINT('Ctrl Pts',(83.8430121840525,21.559829075571,-9.88748044854023));
#9427=CARTESIAN_POINT('Ctrl Pts',(83.3671057189321,21.281254538507,-9.92452482120408));
#9428=CARTESIAN_POINT('Ctrl Pts',(82.7394599712673,21.2619057955038,-9.96156919386793));
#9429=CARTESIAN_POINT('Ctrl Pts',(82.2472979871377,21.5106372121392,-9.99861356653178));
#9430=CARTESIAN_POINT('Ctrl Pts',(81.755136003008,21.7593686287746,-10.0356579391956));
#9431=CARTESIAN_POINT('Ctrl Pts',(81.3984577824135,22.2761802050487,-10.0727023118595));
#9432=CARTESIAN_POINT('Ctrl Pts',(81.3404862984571,22.8245687929057,-10.1097466845233));
#9433=CARTESIAN_POINT('Ctrl Pts',(81.3343655417603,22.8824688653634,-10.1136579108123));
#9434=CARTESIAN_POINT('Ctrl Pts',(81.3315746484398,22.9407209457323,-10.1175691371013));
#9435=CARTESIAN_POINT('Ctrl Pts',(81.3319839553715,22.9990126570311,-10.1214803633902));
#9436=CARTESIAN_POINT('Ctrl Pts',(81.3357306082006,22.9988024506805,-9.92851963660979));
#9437=CARTESIAN_POINT('Ctrl Pts',(81.3344394329371,22.8046311705349,-9.91556613430805));
#9438=CARTESIAN_POINT('Ctrl Pts',(81.3658282901416,22.610864143876,-9.90261263200631));
#9439=CARTESIAN_POINT('Ctrl Pts',(81.4317326497978,22.4296497757676,-9.88965912970457));
#9440=CARTESIAN_POINT('Ctrl Pts',(81.6202056667786,21.9114136703591,-9.85261475704072));
#9441=CARTESIAN_POINT('Ctrl Pts',(82.0909613921934,21.4958386361202,-9.81557038437687));
#9442=CARTESIAN_POINT('Ctrl Pts',(82.6285727417101,21.373099987156,-9.77852601171301));
#9443=CARTESIAN_POINT('Ctrl Pts',(83.1661840912268,21.2503613381917,-9.74148163904916));
#9444=CARTESIAN_POINT('Ctrl Pts',(83.7706510648454,21.420459074502,-9.7044372663853));
#9445=CARTESIAN_POINT('Ctrl Pts',(84.1653576796438,21.80555312446,-9.66739289372145));
#9446=CARTESIAN_POINT('Ctrl Pts',(84.5600642944423,22.1906471744179,-9.6303485210576));
#9447=CARTESIAN_POINT('Ctrl Pts',(84.7450105504205,22.7907375380235,-9.59330414839374));
#9448=CARTESIAN_POINT('Ctrl Pts',(84.6355614011362,23.3312110552286,-9.55625977572989));
#9449=CARTESIAN_POINT('Ctrl Pts',(84.5261122518518,23.8716845724337,-9.51921540306604));
#9450=CARTESIAN_POINT('Ctrl Pts',(84.1222676973048,24.3525412432383,-9.48217103040219));
#9451=CARTESIAN_POINT('Ctrl Pts',(83.6088349532393,24.553731591913,-9.44512665773834));
#9452=CARTESIAN_POINT('Ctrl Pts',(83.0954022091738,24.7549219405877,-9.40808228507448));
#9453=CARTESIAN_POINT('Ctrl Pts',(82.4723812755898,24.6764459671325,-9.37103791241063));
#9454=CARTESIAN_POINT('Ctrl Pts',(82.0248787926276,24.3542158213969,-9.33399353974677));
#9455=CARTESIAN_POINT('Ctrl Pts',(81.6001644105017,24.0483945523337,-9.29883557203444));
#9456=CARTESIAN_POINT('Ctrl Pts',(81.3335478235868,23.5230123364042,-9.26367760432212));
#9457=CARTESIAN_POINT('Ctrl Pts',(81.3314317338341,22.9994875421002,-9.22851963660979));
#9458=CARTESIAN_POINT('Origin',(83.,23.,-12.));
#9459=CARTESIAN_POINT('',(81.3342211202573,23.0015219661406,-8.52851963660979));
#9460=CARTESIAN_POINT('',(81.3367006745913,23.0000736897444,-8.72148036339021));
#9461=CARTESIAN_POINT('',(81.334,23.,-12.));
#9462=CARTESIAN_POINT('Ctrl Pts',(81.3367006745913,23.0000736897444,-8.72148036339021));
#9463=CARTESIAN_POINT('Ctrl Pts',(81.3365927347494,23.2736326870282,-8.73970333180169));
#9464=CARTESIAN_POINT('Ctrl Pts',(81.4003184029638,23.5471443306604,-8.75792630021316));
#9465=CARTESIAN_POINT('Ctrl Pts',(81.5281532937941,23.7864026369698,-8.77614926862464));
#9466=CARTESIAN_POINT('Ctrl Pts',(81.7880211280806,24.2727764077912,-8.81319364128849));
#9467=CARTESIAN_POINT('Ctrl Pts',(82.3128162877671,24.6176004191139,-8.85023801395234));
#9468=CARTESIAN_POINT('Ctrl Pts',(82.8623821799344,24.6630764172596,-8.8872823866162));
#9469=CARTESIAN_POINT('Ctrl Pts',(83.4119480721017,24.7085524154054,-8.92432675928005));
#9470=CARTESIAN_POINT('Ctrl Pts',(83.9862846967497,24.4546804003742,-8.9613711319439));
#9471=CARTESIAN_POINT('Ctrl Pts',(84.3225643115941,24.0176372024102,-8.99841550460776));
#9472=CARTESIAN_POINT('Ctrl Pts',(84.6588439264386,23.5805940044462,-9.03545987727161));
#9473=CARTESIAN_POINT('Ctrl Pts',(84.7570665314794,22.9603796235494,-9.07250424993546));
#9474=CARTESIAN_POINT('Ctrl Pts',(84.5722835296534,22.4408163661117,-9.10954862259932));
#9475=CARTESIAN_POINT('Ctrl Pts',(84.3875005278274,21.9212531086739,-9.14659299526317));
#9476=CARTESIAN_POINT('Ctrl Pts',(83.9197119191345,21.5023409746951,-9.18363736792702));
#9477=CARTESIAN_POINT('Ctrl Pts',(83.3829869769,21.3757824007978,-9.22068174059087));
#9478=CARTESIAN_POINT('Ctrl Pts',(82.8462620346654,21.2492238269004,-9.25772611325473));
#9479=CARTESIAN_POINT('Ctrl Pts',(82.2406007588892,21.4150188130846,-9.29477048591858));
#9480=CARTESIAN_POINT('Ctrl Pts',(81.8431656686657,21.7972963108572,-9.33181485858244));
#9481=CARTESIAN_POINT('Ctrl Pts',(81.5225032177487,22.1057291653825,-9.36170336018503));
#9482=CARTESIAN_POINT('Ctrl Pts',(81.3373906478447,22.5550865564124,-9.39159186178762));
#9483=CARTESIAN_POINT('Ctrl Pts',(81.3333049749392,23.0014544405517,-9.42148036339021));
#9484=CARTESIAN_POINT('Ctrl Pts',(81.3314317338341,22.9994875421002,-9.22851963660979));
#9485=CARTESIAN_POINT('Ctrl Pts',(81.331318194786,22.9713977568116,-9.22663323165826));
#9486=CARTESIAN_POINT('Ctrl Pts',(81.3319661187671,22.9433133188019,-9.22474682670673));
#9487=CARTESIAN_POINT('Ctrl Pts',(81.3333919413996,22.9152684297273,-9.22286042175521));
#9488=CARTESIAN_POINT('Ctrl Pts',(81.3613916054742,22.3645355018094,-9.18581604909136));
#9489=CARTESIAN_POINT('Ctrl Pts',(81.6893749659637,21.8290539639894,-9.14877167642751));
#9490=CARTESIAN_POINT('Ctrl Pts',(82.1672503824573,21.5538707061649,-9.11172730376366));
#9491=CARTESIAN_POINT('Ctrl Pts',(82.6451257989509,21.2786874483404,-9.0746829310998));
#9492=CARTESIAN_POINT('Ctrl Pts',(83.2728932714485,21.2638024705112,-9.03763855843595));
#9493=CARTESIAN_POINT('Ctrl Pts',(83.7632740501943,21.5160274314317,-9.00059418577209));
#9494=CARTESIAN_POINT('Ctrl Pts',(84.2536548289401,21.7682523923522,-8.96354981310824));
#9495=CARTESIAN_POINT('Ctrl Pts',(84.606648913934,22.2875872920222,-8.92650544044439));
#9496=CARTESIAN_POINT('Ctrl Pts',(84.6607192650221,22.8363742600094,-8.88946106778053));
#9497=CARTESIAN_POINT('Ctrl Pts',(84.7147896161103,23.3851612279965,-8.85241669511668));
#9498=CARTESIAN_POINT('Ctrl Pts',(84.4699362332925,23.9634002643006,-8.81537232245283));
#9499=CARTESIAN_POINT('Ctrl Pts',(84.0382088432236,24.3064778061407,-8.77832794978898));
#9500=CARTESIAN_POINT('Ctrl Pts',(83.6064814531546,24.6495553479807,-8.74128357712513));
#9501=CARTESIAN_POINT('Ctrl Pts',(82.9878800558344,24.7574713953565,-8.70423920446127));
#9502=CARTESIAN_POINT('Ctrl Pts',(82.4654888246145,24.5808414414913,-8.66719483179742));
#9503=CARTESIAN_POINT('Ctrl Pts',(81.9430975933946,24.4042114876261,-8.63015045913357));
#9504=CARTESIAN_POINT('Ctrl Pts',(81.5169165282749,23.9430355325199,-8.59310608646971));
#9505=CARTESIAN_POINT('Ctrl Pts',(81.381974471854,23.4083567685463,-8.55606171380586));
#9506=CARTESIAN_POINT('Ctrl Pts',(81.3485318347526,23.275847539447,-8.54688102140717));
#9507=CARTESIAN_POINT('Ctrl Pts',(81.3329769563652,23.1388238034631,-8.53770032900848));
#9508=CARTESIAN_POINT('Ctrl Pts',(81.3342211202573,23.0015219661406,-8.52851963660979));
#9509=CARTESIAN_POINT('Origin',(83.,23.,-12.));
#9510=CARTESIAN_POINT('',(81.3366057744099,22.9995801773856,-7.82851963660979));
#9511=CARTESIAN_POINT('',(81.3335754310806,22.9985070363431,-8.02148036339021));
#9512=CARTESIAN_POINT('',(81.334,23.,-12.));
#9513=CARTESIAN_POINT('Ctrl Pts',(81.3335754310806,22.9985070363431,-8.02148036339021));
#9514=CARTESIAN_POINT('Ctrl Pts',(81.3376142783493,23.4361202976576,-8.05077042915191));
#9515=CARTESIAN_POINT('Ctrl Pts',(81.5146048683971,23.8766246058543,-8.08006049491359));
#9516=CARTESIAN_POINT('Ctrl Pts',(81.8239355688047,24.1839063669557,-8.10935056067528));
#9517=CARTESIAN_POINT('Ctrl Pts',(82.2151590585539,24.5725384773669,-8.14639493333913));
#9518=CARTESIAN_POINT('Ctrl Pts',(82.8180700843827,24.7480715305975,-8.18343930600298));
#9519=CARTESIAN_POINT('Ctrl Pts',(83.3567646970391,24.6301781453598,-8.22048367866684));
#9520=CARTESIAN_POINT('Ctrl Pts',(83.8954593096956,24.5122847601222,-8.2575280513307));
#9521=CARTESIAN_POINT('Ctrl Pts',(84.3699375091796,24.1009649364163,-8.29457242399455));
#9522=CARTESIAN_POINT('Ctrl Pts',(84.5630687330952,23.5844467211039,-8.33161679665841));
#9523=CARTESIAN_POINT('Ctrl Pts',(84.7561999570107,23.0679285057914,-8.36866116932226));
#9524=CARTESIAN_POINT('Ctrl Pts',(84.6679842053578,22.4462118988724,-8.4057055419861));
#9525=CARTESIAN_POINT('Ctrl Pts',(84.3387907424989,22.0038066545161,-8.44274991464995));
#9526=CARTESIAN_POINT('Ctrl Pts',(84.0095972796401,21.5614014101598,-8.47979428731381));
#9527=CARTESIAN_POINT('Ctrl Pts',(83.4394261055753,21.2983075283662,-8.51683865997767));
#9528=CARTESIAN_POINT('Ctrl Pts',(82.8891987702469,21.334921947292,-8.55388303264152));
#9529=CARTESIAN_POINT('Ctrl Pts',(82.3389714349186,21.3715363662178,-8.59092740530538));
#9530=CARTESIAN_POINT('Ctrl Pts',(81.8086879383266,21.707859085863,-8.62797177796922));
#9531=CARTESIAN_POINT('Ctrl Pts',(81.5410164444739,22.1899822108456,-8.66501615063307));
#9532=CARTESIAN_POINT('Ctrl Pts',(81.4050186388596,22.4349380187644,-8.68383755488545));
#9533=CARTESIAN_POINT('Ctrl Pts',(81.3368121591394,22.7175311116915,-8.70265895913783));
#9534=CARTESIAN_POINT('Ctrl Pts',(81.3367006745913,23.0000736897444,-8.72148036339021));
#9535=CARTESIAN_POINT('Ctrl Pts',(81.3342211202573,23.0015219661406,-8.52851963660979));
#9536=CARTESIAN_POINT('Ctrl Pts',(81.3379971954574,22.5848067197478,-8.50065595634463));
#9537=CARTESIAN_POINT('Ctrl Pts',(81.4965161259226,22.1655297680809,-8.47279227607946));
#9538=CARTESIAN_POINT('Ctrl Pts',(81.779340767355,21.8621279077235,-8.4449285958143));
#9539=CARTESIAN_POINT('Ctrl Pts',(82.1553521669993,21.4587593837155,-8.40788422315045));
#9540=CARTESIAN_POINT('Ctrl Pts',(82.7510780140101,21.2602039085407,-8.37083985048659));
#9541=CARTESIAN_POINT('Ctrl Pts',(83.293902437176,21.3573243730351,-8.33379547782274));
#9542=CARTESIAN_POINT('Ctrl Pts',(83.836726860342,21.4544448375295,-8.29675110515889));
#9543=CARTESIAN_POINT('Ctrl Pts',(84.3266498596631,21.847241241693,-8.25970673249503));
#9544=CARTESIAN_POINT('Ctrl Pts',(84.5394730287578,22.355962225086,-8.22266235983118));
#9545=CARTESIAN_POINT('Ctrl Pts',(84.7522961978524,22.864683208479,-8.18561798716733));
#9546=CARTESIAN_POINT('Ctrl Pts',(84.6880195367206,23.4893287711015,-8.14857361450347));
#9547=CARTESIAN_POINT('Ctrl Pts',(84.3760573110503,23.9440488020894,-8.11152924183962));
#9548=CARTESIAN_POINT('Ctrl Pts',(84.06409508538,24.3987688330773,-8.07448486917577));
#9549=CARTESIAN_POINT('Ctrl Pts',(83.5044472951711,24.6835633324306,-8.03744049651192));
#9550=CARTESIAN_POINT('Ctrl Pts',(82.9532197817844,24.6681047495028,-8.00039612384807));
#9551=CARTESIAN_POINT('Ctrl Pts',(82.4019922683977,24.6526461665751,-7.96335175118421));
#9552=CARTESIAN_POINT('Ctrl Pts',(81.859185031833,24.3369345013664,-7.92630737852035));
#9553=CARTESIAN_POINT('Ctrl Pts',(81.5731973482785,23.8654455911985,-7.8892630058565));
#9554=CARTESIAN_POINT('Ctrl Pts',(81.416881609315,23.6077382085239,-7.8690152161076));
#9555=CARTESIAN_POINT('Ctrl Pts',(81.3372912138979,23.3034920693719,-7.84876742635869));
#9556=CARTESIAN_POINT('Ctrl Pts',(81.3366057744099,22.9995801773856,-7.82851963660979));
#9557=CARTESIAN_POINT('Origin',(83.,23.,-12.));
#9558=CARTESIAN_POINT('',(81.3326822579993,22.9986976815004,-7.12851963660979));
#9559=CARTESIAN_POINT('',(81.3317908287134,23.0008588708997,-7.32148036339021));
#9560=CARTESIAN_POINT('',(81.334,23.,-12.));
#9561=CARTESIAN_POINT('Ctrl Pts',(81.3317908287134,23.0008588708997,-7.32148036339021));
#9562=CARTESIAN_POINT('Ctrl Pts',(81.3314807791329,23.0502166331272,-7.32479315383826));
#9563=CARTESIAN_POINT('Ctrl Pts',(81.333481500878,23.099548907092,-7.32810594428632));
#9564=CARTESIAN_POINT('Ctrl Pts',(81.3378748305336,23.1486671753356,-7.33141873473437));
#9565=CARTESIAN_POINT('Ctrl Pts',(81.3870020372038,23.6979187691063,-7.36846310739822));
#9566=CARTESIAN_POINT('Ctrl Pts',(81.7353061679567,24.2204106196216,-7.40550748006207));
#9567=CARTESIAN_POINT('Ctrl Pts',(82.2233962297481,24.4770403834683,-7.44255185272593));
#9568=CARTESIAN_POINT('Ctrl Pts',(82.7114862915396,24.733670147315,-7.47959622538978));
#9569=CARTESIAN_POINT('Ctrl Pts',(83.3393622843697,24.7244378244931,-7.51664059805363));
#9570=CARTESIAN_POINT('Ctrl Pts',(83.8196958818033,24.4535682023601,-7.55368497071749));
#9571=CARTESIAN_POINT('Ctrl Pts',(84.300029479237,24.182698580227,-7.59072934338134));
#9572=CARTESIAN_POINT('Ctrl Pts',(84.6328206812744,23.6501916587828,-7.62777371604519));
#9573=CARTESIAN_POINT('Ctrl Pts',(84.6657776422957,23.0997331376905,-7.66481808870905));
#9574=CARTESIAN_POINT('Ctrl Pts',(84.6987346033171,22.5492746165983,-7.7018624613729));
#9575=CARTESIAN_POINT('Ctrl Pts',(84.4318573233225,21.9808644958579,-7.73890683403675));
#9576=CARTESIAN_POINT('Ctrl Pts',(83.9872741189408,21.6546184064601,-7.77595120670061));
#9577=CARTESIAN_POINT('Ctrl Pts',(83.5426909145591,21.3283723170624,-7.81299557936446));
#9578=CARTESIAN_POINT('Ctrl Pts',(82.9204017857903,21.2442902590072,-7.85003995202831));
#9579=CARTESIAN_POINT('Ctrl Pts',(82.4051784738551,21.4408498500478,-7.88708432469217));
#9580=CARTESIAN_POINT('Ctrl Pts',(81.8899551619199,21.6374094410885,-7.92412869735602));
#9581=CARTESIAN_POINT('Ctrl Pts',(81.4817976668182,22.1146106812249,-7.96117307001987));
#9582=CARTESIAN_POINT('Ctrl Pts',(81.3674868961021,22.6540768850889,-7.99821744268373));
#9583=CARTESIAN_POINT('Ctrl Pts',(81.3435588137885,22.7670005549285,-8.00597174958589));
#9584=CARTESIAN_POINT('Ctrl Pts',(81.3325061790855,22.8826524814131,-8.01372605648805));
#9585=CARTESIAN_POINT('Ctrl Pts',(81.3335754310806,22.9985070363431,-8.02148036339021));
#9586=CARTESIAN_POINT('Ctrl Pts',(81.3366057744099,22.9995801773856,-7.82851963660979));
#9587=CARTESIAN_POINT('Ctrl Pts',(81.3360371671033,22.7474696331785,-7.81172305369484));
#9588=CARTESIAN_POINT('Ctrl Pts',(81.3897674449501,22.4955891030212,-7.7949264707799));
#9589=CARTESIAN_POINT('Ctrl Pts',(81.4990408624314,22.2706965303371,-7.77812988786495));
#9590=CARTESIAN_POINT('Ctrl Pts',(81.7400401906833,21.774702534771,-7.7410855152011));
#9591=CARTESIAN_POINT('Ctrl Pts',(82.2512069777315,21.4099806987659,-7.70404114253724));
#9592=CARTESIAN_POINT('Ctrl Pts',(82.7986212516801,21.3434347775978,-7.66699676987339));
#9593=CARTESIAN_POINT('Ctrl Pts',(83.3460355256286,21.2768888564297,-7.62995239720953));
#9594=CARTESIAN_POINT('Ctrl Pts',(83.9296972864776,21.5085188500986,-7.59290802454568));
#9595=CARTESIAN_POINT('Ctrl Pts',(84.2825114071208,21.9323265833871,-7.55586365188183));
#9596=CARTESIAN_POINT('Ctrl Pts',(84.635325527764,22.3561343166757,-7.51881927921797));
#9597=CARTESIAN_POINT('Ctrl Pts',(84.7572920082014,22.972119789584,-7.48177490655412));
#9598=CARTESIAN_POINT('Ctrl Pts',(84.5925966245821,23.4983953920944,-7.44473053389027));
#9599=CARTESIAN_POINT('Ctrl Pts',(84.4279012409627,24.0246709946049,-7.40768616122641));
#9600=CARTESIAN_POINT('Ctrl Pts',(83.9765439932867,24.4612367267175,-7.37064178856256));
#9601=CARTESIAN_POINT('Ctrl Pts',(83.445074765178,24.608312585173,-7.33359741589871));
#9602=CARTESIAN_POINT('Ctrl Pts',(82.9136055370693,24.7553884436286,-7.29655304323486));
#9603=CARTESIAN_POINT('Ctrl Pts',(82.302024328528,24.6129744284271,-7.259508670571));
#9604=CARTESIAN_POINT('Ctrl Pts',(81.8902028870342,24.2462398670019,-7.22246429790715));
#9605=CARTESIAN_POINT('Ctrl Pts',(81.542076005189,23.9362264814174,-7.19114941080803));
#9606=CARTESIAN_POINT('Ctrl Pts',(81.3366955463558,23.4659157744314,-7.15983452370891));
#9607=CARTESIAN_POINT('Ctrl Pts',(81.3326822579993,22.9986976815004,-7.12851963660979));
#9608=CARTESIAN_POINT('Origin',(83.,23.,-12.));
#9609=CARTESIAN_POINT('',(81.3325224760112,23.0012132743929,-6.42851963660979));
#9610=CARTESIAN_POINT('',(81.3361556106367,23.000944168981,-6.62148036339021));
#9611=CARTESIAN_POINT('',(81.334,23.,-12.));
#9612=CARTESIAN_POINT('',(84.2690708798524,24.0793586530485,-6.));
#9613=CARTESIAN_POINT('Ctrl Pts',(81.3325224760112,23.0012132743929,-6.42851963660979));
#9614=CARTESIAN_POINT('Ctrl Pts',(81.336457103811,22.5283745880917,-6.39681287573142));
#9615=CARTESIAN_POINT('Ctrl Pts',(81.5476198272028,22.0525508339784,-6.36510611485305));
#9616=CARTESIAN_POINT('Ctrl Pts',(81.9034041940898,21.742267204439,-6.33339935397468));
#9617=CARTESIAN_POINT('Ctrl Pts',(82.3190823746991,21.379749492578,-6.29635498131082));
#9618=CARTESIAN_POINT('Ctrl Pts',(82.9321727728451,21.2431982563679,-6.25931060864697));
#9619=CARTESIAN_POINT('Ctrl Pts',(83.4620472172122,21.3961907172468,-6.22226623598311));
#9620=CARTESIAN_POINT('Ctrl Pts',(83.9919216615793,21.5491831781257,-6.18522186331926));
#9621=CARTESIAN_POINT('Ctrl Pts',(84.4385801521673,21.9917193360936,-6.14817749065541));
#9622=CARTESIAN_POINT('Ctrl Pts',(84.5975917113444,22.5187686702513,-6.11113311799156));
#9623=CARTESIAN_POINT('Ctrl Pts',(84.7566032705217,23.0458180044091,-6.0740887453277));
#9624=CARTESIAN_POINT('Ctrl Pts',(84.627967898288,23.6573805147568,-6.03704437266385));
#9625=CARTESIAN_POINT('Ctrl Pts',(84.2690708798524,24.0793586530485,-6.));
#9626=CARTESIAN_POINT('',(81.7285276007435,24.0812047294779,-6.));
#9627=CARTESIAN_POINT('Origin',(83.,23.,-6.));
#9628=CARTESIAN_POINT('Ctrl Pts',(81.7285261364169,24.0812058551231,-6.));
#9629=CARTESIAN_POINT('Ctrl Pts',(82.0793423217202,24.4926754274034,-6.03631814560908));
#9630=CARTESIAN_POINT('Ctrl Pts',(82.6492094921542,24.7187178987082,-6.07263629121814));
#9631=CARTESIAN_POINT('Ctrl Pts',(83.1865491604904,24.6581958582692,-6.10895443682721));
#9632=CARTESIAN_POINT('Ctrl Pts',(83.7346336121355,24.5964636034197,-6.14599880949106));
#9633=CARTESIAN_POINT('Ctrl Pts',(84.2488766988198,24.2365918173637,-6.18304318215492));
#9634=CARTESIAN_POINT('Ctrl Pts',(84.4942852948547,23.742845889402,-6.22008755481878));
#9635=CARTESIAN_POINT('Ctrl Pts',(84.7396938908897,23.2490999614404,-6.25713192748263));
#9636=CARTESIAN_POINT('Ctrl Pts',(84.7162679962753,22.6214798915731,-6.29417630014648));
#9637=CARTESIAN_POINT('Ctrl Pts',(84.4345602009582,22.1474061483613,-6.33122067281033));
#9638=CARTESIAN_POINT('Ctrl Pts',(84.1528524056412,21.6733324051495,-6.36826504547418));
#9639=CARTESIAN_POINT('Ctrl Pts',(83.6128627096214,21.3528049885932,-6.40530941813804));
#9640=CARTESIAN_POINT('Ctrl Pts',(83.0617850229002,21.3323987424867,-6.44235379080189));
#9641=CARTESIAN_POINT('Ctrl Pts',(82.5107073361791,21.3119924963801,-6.47939816346575));
#9642=CARTESIAN_POINT('Ctrl Pts',(81.9485416587566,21.5917074207234,-6.5164425361296));
#9643=CARTESIAN_POINT('Ctrl Pts',(81.6325039520559,22.0435930082728,-6.55348690879345));
#9644=CARTESIAN_POINT('Ctrl Pts',(81.4391457897928,22.3200656091972,-6.57615139365904));
#9645=CARTESIAN_POINT('Ctrl Pts',(81.3379191370965,22.6609857536405,-6.59881587852463));
#9646=CARTESIAN_POINT('Ctrl Pts',(81.3361556106367,23.000944168981,-6.62148036339021));
#9647=CARTESIAN_POINT('Origin',(83.,23.,-4.45407471946233));
#9648=CARTESIAN_POINT('',(80.9445918561381,23.001823176295,-16.6459252805377));
#9649=CARTESIAN_POINT('',(80.9470731721499,22.9984940384348,-16.7040747194623));
#9650=CARTESIAN_POINT('',(80.94525,23.0000000000001,-4.45407471946233));
#9651=CARTESIAN_POINT('',(84.8174278887595,23.9586205879593,-17.));
#9652=CARTESIAN_POINT('Ctrl Pts',(80.9470731721499,22.9984940384348,-16.7040747194623));
#9653=CARTESIAN_POINT('Ctrl Pts',(80.9500636069218,23.452419291778,-16.7286277343139));
#9654=CARTESIAN_POINT('Ctrl Pts',(81.3216921078483,24.5959829414065,-16.7902251218292));
#9655=CARTESIAN_POINT('Ctrl Pts',(83.2159905896636,25.4179577199457,-16.8888668820084));
#9656=CARTESIAN_POINT('Ctrl Pts',(84.4986774253636,24.5629326473987,-16.9629556273361));
#9657=CARTESIAN_POINT('Ctrl Pts',(84.8174278887595,23.9586205879593,-17.));
#9658=CARTESIAN_POINT('',(85.0570979162306,22.9245442276038,-17.));
#9659=CARTESIAN_POINT('Origin',(83.,23.,-17.));
#9660=CARTESIAN_POINT('Ctrl Pts',(80.9445918561382,23.001823176295,-16.6459252805377));
#9661=CARTESIAN_POINT('Ctrl Pts',(80.9432972802338,23.1421867341789,-16.6535432960883));
#9662=CARTESIAN_POINT('Ctrl Pts',(81.0204256104681,23.9636912996603,-16.6982056843029));
#9663=CARTESIAN_POINT('Ctrl Pts',(82.12637451265,25.2659591550417,-16.7799124451812));
#9664=CARTESIAN_POINT('Ctrl Pts',(84.4138508336827,24.965114478167,-16.890319336118));
#9665=CARTESIAN_POINT('Ctrl Pts',(85.0806816951007,23.591021626778,-16.9636818543909));
#9666=CARTESIAN_POINT('Ctrl Pts',(85.0571001857713,22.9245440319506,-17.));
#9667=CARTESIAN_POINT('Origin',(83.,23.,-4.45407471946233));
#9668=CARTESIAN_POINT('',(80.9485828438711,22.9999504095115,-15.9459252805377));
#9669=CARTESIAN_POINT('',(80.941985868441,22.999516909691,-16.0040747194623));
#9670=CARTESIAN_POINT('',(80.94525,23.0000000000001,-4.45407471946233));
#9671=CARTESIAN_POINT('Ctrl Pts',(80.941985868441,22.999516909691,-16.0040747194623));
#9672=CARTESIAN_POINT('Ctrl Pts',(80.9440549059599,23.6536076635307,-16.0396948316641));
#9673=CARTESIAN_POINT('Ctrl Pts',(81.6350686818089,24.9917162152022,-16.1123593165296));
#9674=CARTESIAN_POINT('Ctrl Pts',(83.9141747198462,25.2499873352066,-16.2220681740591));
#9675=CARTESIAN_POINT('Ctrl Pts',(85.3860300953815,23.4524069852193,-16.3332012920506));
#9676=CARTESIAN_POINT('Ctrl Pts',(84.6743954809949,21.240621211679,-16.4443344100422));
#9677=CARTESIAN_POINT('Ctrl Pts',(82.4296924778299,20.6393768340819,-16.5554675280338));
#9678=CARTESIAN_POINT('Ctrl Pts',(81.0884934760466,21.8537197383225,-16.6420476311738));
#9679=CARTESIAN_POINT('Ctrl Pts',(80.9455517870582,22.767559353067,-16.69158336165));
#9680=CARTESIAN_POINT('Ctrl Pts',(80.9470731721499,22.9984940384348,-16.7040747194623));
#9681=CARTESIAN_POINT('Ctrl Pts',(80.9485828438712,22.9999504095115,-15.9459252805377));
#9682=CARTESIAN_POINT('Ctrl Pts',(80.9486568620999,23.34590005549,-15.9646103934386));
#9683=CARTESIAN_POINT('Ctrl Pts',(81.1957456616406,24.3778157149169,-16.0203398790033));
#9684=CARTESIAN_POINT('Ctrl Pts',(82.8298598776186,25.4226489294061,-16.1131137372319));
#9685=CARTESIAN_POINT('Ctrl Pts',(84.9430514056717,24.4569400344173,-16.2242468552234));
#9686=CARTESIAN_POINT('Ctrl Pts',(85.2779271552008,22.1577886838534,-16.335379973215));
#9687=CARTESIAN_POINT('Ctrl Pts',(83.5278718544653,20.6294494978248,-16.4465130912065));
#9688=CARTESIAN_POINT('Ctrl Pts',(81.4479222208321,21.2267962234199,-16.5500281936475));
#9689=CARTESIAN_POINT('Ctrl Pts',(80.9495924567037,22.4596362835927,-16.6164989234245));
#9690=CARTESIAN_POINT('Ctrl Pts',(80.9445918561382,23.001823176295,-16.6459252805377));
#9691=CARTESIAN_POINT('Origin',(83.,23.,-4.45407471946233));
#9692=CARTESIAN_POINT('',(80.9444684385758,22.9981936684133,-15.2459252805377));
#9693=CARTESIAN_POINT('',(80.9457759848993,23.001865484283,-15.3040747194623));
#9694=CARTESIAN_POINT('',(80.94525,23.0000000000001,-4.45407471946233));
#9695=CARTESIAN_POINT('Ctrl Pts',(80.9457759848993,23.001865484283,-15.3040747194623));
#9696=CARTESIAN_POINT('Ctrl Pts',(80.9441908674823,23.179786033038,-15.3137175563504));
#9697=CARTESIAN_POINT('Ctrl Pts',(81.0468089400269,24.039414645723,-15.3604047659024));
#9698=CARTESIAN_POINT('Ctrl Pts',(82.2507940260338,25.3101655411,-15.4441363481181));
#9699=CARTESIAN_POINT('Ctrl Pts',(84.5344926196224,24.8824203570357,-15.5552694661097));
#9700=CARTESIAN_POINT('Ctrl Pts',(85.4137607912389,22.7318111240602,-15.6664025841013));
#9701=CARTESIAN_POINT('Ctrl Pts',(84.0838648276161,20.8266566062216,-15.7775357020929));
#9702=CARTESIAN_POINT('Ctrl Pts',(81.7619636485858,20.9106360913409,-15.8886688200844));
#9703=CARTESIAN_POINT('Ctrl Pts',(80.9542066368151,22.2670451103755,-15.9641818258742));
#9704=CARTESIAN_POINT('Ctrl Pts',(80.9419031385406,22.9733632694651,-16.0026504590002));
#9705=CARTESIAN_POINT('Ctrl Pts',(80.941985868441,22.999516909691,-16.0040747194623));
#9706=CARTESIAN_POINT('Ctrl Pts',(80.9444684385758,22.9981936684133,-15.2459252805377));
#9707=CARTESIAN_POINT('Ctrl Pts',(80.9494988573722,23.5462600854287,-15.2756774907888));
#9708=CARTESIAN_POINT('Ctrl Pts',(81.4568946603439,24.7849447934067,-15.3424740737037));
#9709=CARTESIAN_POINT('Ctrl Pts',(83.5486977451864,25.3658199574776,-15.4463150292825));
#9710=CARTESIAN_POINT('Ctrl Pts',(85.2852062155397,23.822195101775,-15.5574481472741));
#9711=CARTESIAN_POINT('Ctrl Pts',(84.9302046695978,21.5260650294792,-15.6685812652657));
#9712=CARTESIAN_POINT('Ctrl Pts',(82.8086025275965,20.5789380526202,-15.7797143832572));
#9713=CARTESIAN_POINT('Ctrl Pts',(81.1894352243962,21.6343485525749,-15.8721623883479));
#9714=CARTESIAN_POINT('Ctrl Pts',(80.9485101164599,22.6600338433596,-15.9275660207747));
#9715=CARTESIAN_POINT('Ctrl Pts',(80.9485828438712,22.9999504095115,-15.9459252805377));
#9716=CARTESIAN_POINT('Origin',(83.,23.,-4.45407471946233));
#9717=CARTESIAN_POINT('',(80.9427069405049,23.0011828703653,-14.5459252805377));
#9718=CARTESIAN_POINT('',(80.9483910840592,22.9993486074027,-14.6040747194623));
#9719=CARTESIAN_POINT('',(80.94525,23.0000000000001,-4.45407471946233));
#9720=CARTESIAN_POINT('Ctrl Pts',(80.9483910840592,22.9993486074027,-14.6040747194623));
#9721=CARTESIAN_POINT('Ctrl Pts',(80.9494811123425,23.3826976046307,-14.6247846537006));
#9722=CARTESIAN_POINT('Ctrl Pts',(81.2366608737661,24.4532689341001,-14.6825389606028));
#9723=CARTESIAN_POINT('Ctrl Pts',(82.9621345872503,25.4283202829728,-14.7773376401688));
#9724=CARTESIAN_POINT('Ctrl Pts',(85.0195747495924,24.3488851074018,-14.8884707581604));
#9725=CARTESIAN_POINT('Ctrl Pts',(85.2286205736113,22.0348972082601,-14.9996038761519));
#9726=CARTESIAN_POINT('Ctrl Pts',(83.3979452064162,20.6042093336492,-15.1107369941435));
#9727=CARTESIAN_POINT('Ctrl Pts',(81.3935016039341,21.3001230071733,-15.2122272752469));
#9728=CARTESIAN_POINT('Ctrl Pts',(80.9502803286018,22.4962781412084,-15.2766731836866));
#9729=CARTESIAN_POINT('Ctrl Pts',(80.9457759848993,23.001865484283,-15.3040747194623));
#9730=CARTESIAN_POINT('Ctrl Pts',(80.9427069405049,23.0011828703653,-14.5459252805377));
#9731=CARTESIAN_POINT('Ctrl Pts',(80.9422307466888,23.0705663228386,-14.5497002154751));
#9732=CARTESIAN_POINT('Ctrl Pts',(80.9768964145428,23.8203453482233,-14.5905195230765));
#9733=CARTESIAN_POINT('Ctrl Pts',(81.8966144503262,25.1634956547744,-14.6683832033416));
#9734=CARTESIAN_POINT('Ctrl Pts',(84.2191696572937,25.1004281633947,-14.7795163213332));
#9735=CARTESIAN_POINT('Ctrl Pts',(85.4258928026212,23.1149661440179,-14.8906494393247));
#9736=CARTESIAN_POINT('Ctrl Pts',(84.4123433832198,21.0242825862308,-15.0017825573163));
#9737=CARTESIAN_POINT('Ctrl Pts',(82.1061616893797,20.7418533657775,-15.1129156753078));
#9738=CARTESIAN_POINT('Ctrl Pts',(81.0164470233792,22.0484774837239,-15.1942965830483));
#9739=CARTESIAN_POINT('Ctrl Pts',(80.9432355005669,22.8638645112809,-15.2386331181249));
#9740=CARTESIAN_POINT('Ctrl Pts',(80.9444684385758,22.9981936684133,-15.2459252805377));
#9741=CARTESIAN_POINT('Origin',(83.,23.,-4.45407471946233));
#9742=CARTESIAN_POINT('',(80.9480449766009,23.0010551249669,-13.8459252805377));
#9743=CARTESIAN_POINT('',(80.9433898278768,22.9984792505039,-13.9040747194623));
#9744=CARTESIAN_POINT('',(80.94525,23.0000000000001,-4.45407471946233));
#9745=CARTESIAN_POINT('Ctrl Pts',(80.9433898278768,22.9984792505039,-13.9040747194623));
#9746=CARTESIAN_POINT('Ctrl Pts',(80.948232962241,23.5830502245177,-13.9358517510509));
#9747=CARTESIAN_POINT('Ctrl Pts',(81.5151171939793,24.8573002990708,-14.0046731553032));
#9748=CARTESIAN_POINT('Ctrl Pts',(83.6768129281338,25.3324016450226,-14.1105389322195));
#9749=CARTESIAN_POINT('Ctrl Pts',(85.3266177853476,23.6964358225195,-14.221672050211));
#9750=CARTESIAN_POINT('Ctrl Pts',(84.8470104700268,21.423064524091,-14.3328051682026));
#9751=CARTESIAN_POINT('Ctrl Pts',(82.676946476112,20.5929666402091,-14.4439382861941));
#9752=CARTESIAN_POINT('Ctrl Pts',(81.1518515427802,21.7100345132185,-14.5343614699474));
#9753=CARTESIAN_POINT('Ctrl Pts',(80.9475313517361,22.6969917520569,-14.5877402810368));
#9754=CARTESIAN_POINT('Ctrl Pts',(80.9483910840592,22.9993486074027,-14.6040747194623));
#9755=CARTESIAN_POINT('Ctrl Pts',(80.9480449766009,23.001055124967,-13.8459252805377));
#9756=CARTESIAN_POINT('Ctrl Pts',(80.9467671657193,23.2756711098727,-13.8607673128254));
#9757=CARTESIAN_POINT('Ctrl Pts',(81.1259274853824,24.2341048917329,-13.9126537177769));
#9758=CARTESIAN_POINT('Ctrl Pts',(82.5805008911621,25.3921107031273,-14.0015844953923));
#9759=CARTESIAN_POINT('Ctrl Pts',(84.7821632663096,24.6498688464973,-14.1127176133838));
#9760=CARTESIAN_POINT('Ctrl Pts',(85.3527196747847,22.397602083335,-14.2238507313754));
#9761=CARTESIAN_POINT('Ctrl Pts',(83.7699744349188,20.6966736036812,-14.3349838493669));
#9762=CARTESIAN_POINT('Ctrl Pts',(81.5602178798653,21.0900095959384,-14.442342032421));
#9763=CARTESIAN_POINT('Ctrl Pts',(80.9469037546942,22.3896892977476,-14.5126558428113));
#9764=CARTESIAN_POINT('Ctrl Pts',(80.9427069405049,23.0011828703653,-14.5459252805377));
#9765=CARTESIAN_POINT('Origin',(83.,23.,-4.45407471946233));
#9766=CARTESIAN_POINT('',(80.9465558937026,22.998246285774,-13.1459252805377));
#9767=CARTESIAN_POINT('',(80.9436610901855,23.0016161418076,-13.2040747194623));
#9768=CARTESIAN_POINT('',(80.94525,23.0000000000001,-4.45407471946233));
#9769=CARTESIAN_POINT('Ctrl Pts',(80.9436610901855,23.0016161418076,-13.2040747194623));
#9770=CARTESIAN_POINT('Ctrl Pts',(80.9427399464891,23.1083452056402,-13.2098744757372));
#9771=CARTESIAN_POINT('Ctrl Pts',(80.9988245257335,23.895806936048,-13.252718604676));
#9772=CARTESIAN_POINT('Ctrl Pts',(82.0161587277924,25.2204120168147,-13.3326071062785));
#9773=CARTESIAN_POINT('Ctrl Pts',(84.3318254372397,25.0308653766405,-13.4437402242701));
#9774=CARTESIAN_POINT('Ctrl Pts',(85.4285530863916,22.9825908096803,-13.5548733422617));
#9775=CARTESIAN_POINT('Ctrl Pts',(84.3025733639503,20.9502498189244,-13.6660064602532));
#9776=CARTESIAN_POINT('Ctrl Pts',(81.9844272300528,20.7939208712606,-13.7771395782448));
#9777=CARTESIAN_POINT('Ctrl Pts',(80.992840331298,22.1240505870937,-13.8564956646478));
#9778=CARTESIAN_POINT('Ctrl Pts',(80.9425870329241,22.9015811278996,-13.898807378387));
#9779=CARTESIAN_POINT('Ctrl Pts',(80.9433898278768,22.9984792505039,-13.9040747194623));
#9780=CARTESIAN_POINT('Ctrl Pts',(80.9465558937026,22.998246285774,-13.1459252805377));
#9781=CARTESIAN_POINT('Ctrl Pts',(80.950443637898,23.4767580065597,-13.1718344101756));
#9782=CARTESIAN_POINT('Ctrl Pts',(81.3555437322658,24.6453701880592,-13.2347879124773));
#9783=CARTESIAN_POINT('Ctrl Pts',(83.3013691324087,25.409844344426,-13.3347857874429));
#9784=CARTESIAN_POINT('Ctrl Pts',(85.1880466324256,24.0538619704037,-13.4459189054344));
#9785=CARTESIAN_POINT('Ctrl Pts',(85.0721377337693,21.7333436414648,-13.557052023426));
#9786=CARTESIAN_POINT('Ctrl Pts',(83.0597268226234,20.5721190669662,-13.6681851414176));
#9787=CARTESIAN_POINT('Ctrl Pts',(81.2687132736902,21.4913058617477,-13.7644762271215));
#9788=CARTESIAN_POINT('Ctrl Pts',(80.94995646632,22.5902544036478,-13.8237229401615));
#9789=CARTESIAN_POINT('Ctrl Pts',(80.9480449766009,23.001055124967,-13.8459252805377));
#9790=CARTESIAN_POINT('Origin',(83.,23.,-4.45407471946233));
#9791=CARTESIAN_POINT('',(80.9418454804923,22.9999766228626,-12.4459252805377));
#9792=CARTESIAN_POINT('',(80.9484733990566,23.0004971809245,-12.5040747194623));
#9793=CARTESIAN_POINT('',(80.94525,23.0000000000001,-4.45407471946233));
#9794=CARTESIAN_POINT('Ctrl Pts',(80.9484733990566,23.0004971809245,-12.5040747194623));
#9795=CARTESIAN_POINT('Ctrl Pts',(80.9477973499854,23.3127405278041,-12.5209415730874));
#9796=CARTESIAN_POINT('Ctrl Pts',(81.1614616883935,24.3098806979921,-12.5748527993764));
#9797=CARTESIAN_POINT('Ctrl Pts',(82.7114877530095,25.4114173957764,-12.6658083983292));
#9798=CARTESIAN_POINT('Ctrl Pts',(84.8694281534639,24.5502940212596,-12.7769415163208));
#9799=CARTESIAN_POINT('Ctrl Pts',(85.3163943278932,22.2702805395079,-12.8880746343123));
#9800=CARTESIAN_POINT('Ctrl Pts',(83.6433052410424,20.6581350294767,-12.9992077523039));
#9801=CARTESIAN_POINT('Ctrl Pts',(81.4994790128079,21.1616334099512,-13.1045411140205));
#9802=CARTESIAN_POINT('Ctrl Pts',(80.9486235024093,22.4266422120513,-13.1728301030734));
#9803=CARTESIAN_POINT('Ctrl Pts',(80.9436610901855,23.0016161418076,-13.2040747194623));
#9804=CARTESIAN_POINT('Ctrl Pts',(80.941845609139,22.999976623746,-12.4459252805377));
#9805=CARTESIAN_POINT('Ctrl Pts',(80.9419597659312,23.6788458613235,-12.4829015075258));
#9806=CARTESIAN_POINT('Ctrl Pts',(81.6804454174154,25.0380482591789,-12.5569221071778));
#9807=CARTESIAN_POINT('Ctrl Pts',(83.9956695619749,25.2151332333942,-12.6679870794935));
#9808=CARTESIAN_POINT('Ctrl Pts',(85.4010382767464,23.364949738908,-12.7791201974851));
#9809=CARTESIAN_POINT('Ctrl Pts',(84.6088822566941,21.1807498790914,-12.8902533154767));
#9810=CARTESIAN_POINT('Ctrl Pts',(82.3442138703267,20.6615993349174,-13.0013864334682));
#9811=CARTESIAN_POINT('Ctrl Pts',(81.0677939508996,21.9047210022768,-13.0866104218219));
#9812=CARTESIAN_POINT('Ctrl Pts',(80.9448850164079,22.7925911990848,-13.1347900375117));
#9813=CARTESIAN_POINT('Ctrl Pts',(80.9465558937026,22.998246285774,-13.1459252805377));
#9814=CARTESIAN_POINT('Origin',(83.,23.,-4.45407471946233));
#9815=CARTESIAN_POINT('',(80.946487742054,23.0017684726493,-11.7459252805377));
#9816=CARTESIAN_POINT('',(80.9454838921393,22.9981221128236,-11.8040747194623));
#9817=CARTESIAN_POINT('',(80.94525,23.0000000000001,-4.45407471946233));
#9818=CARTESIAN_POINT('Ctrl Pts',(80.9454838921393,22.9981221128236,-11.8040747194623));
#9819=CARTESIAN_POINT('Ctrl Pts',(80.9501624736055,23.5133464089528,-11.8320086704376));
#9820=CARTESIAN_POINT('Ctrl Pts',(81.4074703003843,24.7192340376815,-11.8969869940768));
#9821=CARTESIAN_POINT('Ctrl Pts',(83.4322511648908,25.3898393468531,-11.9990096903799));
#9822=CARTESIAN_POINT('Ctrl Pts',(85.2422276109297,23.9330533286481,-12.1101428083714));
#9823=CARTESIAN_POINT('Ctrl Pts',(85.000029094227,21.6223001794432,-12.221275926363));
#9824=CARTESIAN_POINT('Ctrl Pts',(82.9273252301097,20.5724721317484,-12.3324090443545));
#9825=CARTESIAN_POINT('Ctrl Pts',(81.2256187435467,21.5665457480708,-12.426675308721));
#9826=CARTESIAN_POINT('Ctrl Pts',(80.9492821446181,22.626965980831,-12.4838972004236));
#9827=CARTESIAN_POINT('Ctrl Pts',(80.9484733990566,23.0004971809245,-12.5040747194623));
#9828=CARTESIAN_POINT('Ctrl Pts',(80.946487742054,23.0017684726493,-11.7459252805377));
#9829=CARTESIAN_POINT('Ctrl Pts',(80.9448193888947,23.2048893572511,-11.7569242322121));
#9830=CARTESIAN_POINT('Ctrl Pts',(81.0658212075453,24.0901758494269,-11.8049675565505));
#9831=CARTESIAN_POINT('Ctrl Pts',(82.3356362705467,25.3359781577142,-11.8900552535526));
#9832=CARTESIAN_POINT('Ctrl Pts',(84.6021947068076,24.825142525889,-12.0011883715442));
#9833=CARTESIAN_POINT('Ctrl Pts',(85.4023614856292,22.6438646174604,-12.1123214895358));
#9834=CARTESIAN_POINT('Ctrl Pts',(84.0037924767762,20.7885358284841,-12.2234546075273));
#9835=CARTESIAN_POINT('Ctrl Pts',(81.6865130842908,20.9572260916608,-12.3345877255189));
#9836=CARTESIAN_POINT('Ctrl Pts',(80.9424129889364,22.3173541979826,-12.4087446165223));
#9837=CARTESIAN_POINT('Ctrl Pts',(80.9418453987527,22.9987254954749,-12.4458571348619));
#9838=CARTESIAN_POINT('Ctrl Pts',(80.941845609139,22.999976623746,-12.4459252805377));
#9839=CARTESIAN_POINT('Origin',(83.,23.,-4.45407471946233));
#9840=CARTESIAN_POINT('',(80.9480833902501,22.9989795845752,-11.0459252805377));
#9841=CARTESIAN_POINT('',(80.942099557822,23.0006544392887,-11.1040747194623));
#9842=CARTESIAN_POINT('',(80.94525,23.0000000000001,-4.45407471946233));
#9843=CARTESIAN_POINT('Ctrl Pts',(80.942099557822,23.0006544392887,-11.1040747194623));
#9844=CARTESIAN_POINT('Ctrl Pts',(80.941949761973,23.0365901265997,-11.106031395124));
#9845=CARTESIAN_POINT('Ctrl Pts',(80.9590874886889,23.7527252524841,-11.1450324434495));
#9846=CARTESIAN_POINT('Ctrl Pts',(81.7920500466204,25.1069005869871,-11.2210778644389));
#9847=CARTESIAN_POINT('Ctrl Pts',(84.1149085920925,25.1575801270393,-11.3322109824305));
#9848=CARTESIAN_POINT('Ctrl Pts',(85.4173589117072,23.2335574132988,-11.4433441004221));
#9849=CARTESIAN_POINT('Ctrl Pts',(84.5073472090078,21.0957737621771,-11.5544772184136));
#9850=CARTESIAN_POINT('Ctrl Pts',(82.2177520120164,20.7008129135252,-11.6656103364052));
#9851=CARTESIAN_POINT('Ctrl Pts',(81.0396472413493,21.980504676805,-11.7488095034214));
#9852=CARTESIAN_POINT('Ctrl Pts',(80.9439580123917,22.8300860692986,-11.7949642977738));
#9853=CARTESIAN_POINT('Ctrl Pts',(80.9454838921393,22.9981221128236,-11.8040747194623));
#9854=CARTESIAN_POINT('Ctrl Pts',(80.9480833902501,22.9989795845752,-11.0459252805377));
#9855=CARTESIAN_POINT('Ctrl Pts',(80.9499186191076,23.4072776930713,-11.0679913295624));
#9856=CARTESIAN_POINT('Ctrl Pts',(81.2657181967231,24.5036404128733,-11.1271017512509));
#9857=CARTESIAN_POINT('Ctrl Pts',(83.0508160082765,25.4280837818398,-11.2232565456033));
#9858=CARTESIAN_POINT('Ctrl Pts',(85.0674751034236,24.2742526496163,-11.3343896635948));
#9859=CARTESIAN_POINT('Ctrl Pts',(85.1918996088904,21.9541753383684,-11.4455227815864));
#9860=CARTESIAN_POINT('Ctrl Pts',(83.3102113199728,20.5912779207033,-11.5566558995779));
#9861=CARTESIAN_POINT('Ctrl Pts',(81.3589375218264,21.3496378721918,-11.6567900658951));
#9862=CARTESIAN_POINT('Ctrl Pts',(80.9504383876862,22.5207800014051,-11.7198798595483));
#9863=CARTESIAN_POINT('Ctrl Pts',(80.946487742054,23.0017684726493,-11.7459252805377));
#9864=CARTESIAN_POINT('Origin',(83.,23.,-4.45407471946233));
#9865=CARTESIAN_POINT('',(80.9427635247896,22.9987822671278,-10.3459252805377));
#9866=CARTESIAN_POINT('',(80.9474130033736,23.0014635246622,-10.4040747194623));
#9867=CARTESIAN_POINT('',(80.94525,23.0000000000001,-4.45407471946233));
#9868=CARTESIAN_POINT('Ctrl Pts',(80.9474130033736,23.0014635246621,-10.4040747194623));
#9869=CARTESIAN_POINT('Ctrl Pts',(80.9458279183746,23.2422509457676,-10.4170984924742));
#9870=CARTESIAN_POINT('Ctrl Pts',(81.0963187654959,24.1660078235155,-10.46716663815));
#9871=CARTESIAN_POINT('Ctrl Pts',(82.4639279501368,25.3687127159435,-10.5542791564896));
#9872=CARTESIAN_POINT('Ctrl Pts',(84.6992789742144,24.7351150224436,-10.6654122744811));
#9873=CARTESIAN_POINT('Ctrl Pts',(85.3793829981224,22.5134717669416,-10.7765453924727));
#9874=CARTESIAN_POINT('Ctrl Pts',(83.8817820505465,20.7371182998993,-10.8876785104642));
#9875=CARTESIAN_POINT('Ctrl Pts',(81.617716369494,21.0266541288133,-10.9968549527941));
#9876=CARTESIAN_POINT('Ctrl Pts',(80.9447857420797,22.3562448763623,-11.0689870224602));
#9877=CARTESIAN_POINT('Ctrl Pts',(80.942099557822,23.0006544392887,-11.1040747194623));
#9878=CARTESIAN_POINT('Ctrl Pts',(80.9427635247896,22.9987822671278,-10.3459252805377));
#9879=CARTESIAN_POINT('Ctrl Pts',(80.9470399691646,23.6078148575591,-10.3790584269126));
#9880=CARTESIAN_POINT('Ctrl Pts',(81.5560212788413,24.9052031204881,-10.4492359459513));
#9881=CARTESIAN_POINT('Ctrl Pts',(83.7615159569619,25.3061367187622,-10.5564578376539));
#9882=CARTESIAN_POINT('Ctrl Pts',(85.3504930077305,23.6110284272776,-10.6675909556455));
#9883=CARTESIAN_POINT('Ctrl Pts',(84.7882063433206,21.3566828693041,-10.778724073637));
#9884=CARTESIAN_POINT('Ctrl Pts',(82.5892828503881,20.6063658296754,-10.8898571916286));
#9885=CARTESIAN_POINT('Ctrl Pts',(81.1282336040668,21.7607920195001,-10.9789242605955));
#9886=CARTESIAN_POINT('Ctrl Pts',(80.9468376460868,22.7218288720269,-11.0309469568985));
#9887=CARTESIAN_POINT('Ctrl Pts',(80.9480833902501,22.9989795845752,-11.0459252805377));
#9888=CARTESIAN_POINT('Origin',(83.,23.,-4.45407471946233));
#9889=CARTESIAN_POINT('',(80.944392795472,23.0017938245641,-9.64592528053768));
#9890=CARTESIAN_POINT('',(80.9473844340938,22.9985230105256,-9.70407471946232));
#9891=CARTESIAN_POINT('',(80.94525,23.0000000000001,-4.45407471946233));
#9892=CARTESIAN_POINT('Ctrl Pts',(80.9473844340938,22.9985230105256,-9.70407471946232));
#9893=CARTESIAN_POINT('Ctrl Pts',(80.9503460891386,23.4439066603514,-9.72816558982444));
#9894=CARTESIAN_POINT('Ctrl Pts',(81.3116442355096,24.5785301187141,-9.7893008328504));
#9895=CARTESIAN_POINT('Ctrl Pts',(83.1830643805896,25.4217061353262,-9.88748044854022));
#9896=CARTESIAN_POINT('Ctrl Pts',(85.1338459461496,24.1596873076041,-9.99861356653177));
#9897=CARTESIAN_POINT('Ctrl Pts',(85.1316477144354,21.8362770111152,-10.1097466845233));
#9898=CARTESIAN_POINT('Ctrl Pts',(83.1784815936336,20.5779517977441,-10.2208798025149));
#9899=CARTESIAN_POINT('Ctrl Pts',(81.3099985927049,21.4240614634891,-10.3189891474946));
#9900=CARTESIAN_POINT('Ctrl Pts',(80.9503364797073,22.5573634748289,-10.3800541198104));
#9901=CARTESIAN_POINT('Ctrl Pts',(80.9474130033736,23.0014635246621,-10.4040747194623));
#9902=CARTESIAN_POINT('Ctrl Pts',(80.944392795472,23.0017938245641,-9.64592528053768));
#9903=CARTESIAN_POINT('Ctrl Pts',(80.9431863548551,23.1335998594481,-9.65308115159894));
#9904=CARTESIAN_POINT('Ctrl Pts',(81.0147851841557,23.9464313285286,-9.69728139532405));
#9905=CARTESIAN_POINT('Ctrl Pts',(82.0978802396299,25.2548510053398,-9.778526011713));
#9906=CARTESIAN_POINT('Ctrl Pts',(84.4050829104209,24.9808874610066,-9.88965912970457));
#9907=CARTESIAN_POINT('Ctrl Pts',(85.4262983980702,22.8939377453899,-10.0007922476961));
#9908=CARTESIAN_POINT('Ctrl Pts',(84.2268700936312,20.9040603797618,-10.1119253656877));
#9909=CARTESIAN_POINT('Ctrl Pts',(81.9045619903646,20.8324694499553,-10.2230584836792));
#9910=CARTESIAN_POINT('Ctrl Pts',(80.9783022594501,22.1745804170201,-10.3010584552959));
#9911=CARTESIAN_POINT('Ctrl Pts',(80.9422587088125,22.9268885733755,-10.3420140542487));
#9912=CARTESIAN_POINT('Ctrl Pts',(80.9427635247896,22.9987822671278,-10.3459252805377));
#9913=CARTESIAN_POINT('Origin',(83.,23.,-4.45407471946233));
#9914=CARTESIAN_POINT('',(80.9485808590134,23.0000908847554,-8.94592528053768));
#9915=CARTESIAN_POINT('',(80.9420824460358,22.9993679634637,-9.00407471946233));
#9916=CARTESIAN_POINT('',(80.94525,23.0000000000001,-4.45407471946233));
#9917=CARTESIAN_POINT('Ctrl Pts',(80.9420824460358,22.9993679634637,-9.00407471946233));
#9918=CARTESIAN_POINT('Ctrl Pts',(80.9446923112335,23.6450537804481,-9.03923268717465));
#9919=CARTESIAN_POINT('Ctrl Pts',(81.6199952950891,24.9757743563403,-9.11143502755083));
#9920=CARTESIAN_POINT('Ctrl Pts',(83.8860623965075,25.2612091019686,-9.22068174059087));
#9921=CARTESIAN_POINT('Ctrl Pts',(85.3802993685163,23.4820249885188,-9.33181485858242));
#9922=CARTESIAN_POINT('Ctrl Pts',(84.6959926707885,21.2616726332633,-9.44294797657398));
#9923=CARTESIAN_POINT('Ctrl Pts',(82.4594467271343,20.632305903941,-9.55408109456555));
#9924=CARTESIAN_POINT('Ctrl Pts',(81.0952171682793,21.8366242266362,-9.64112334219499));
#9925=CARTESIAN_POINT('Ctrl Pts',(80.9457919716852,22.7590431558563,-9.69112121716058));
#9926=CARTESIAN_POINT('Ctrl Pts',(80.9473844340938,22.9985230105256,-9.70407471946232));
#9927=CARTESIAN_POINT('Ctrl Pts',(80.9485808590134,23.0000908847555,-8.94592528053767));
#9928=CARTESIAN_POINT('Ctrl Pts',(80.9484477321286,23.3374830514234,-8.96414824894915));
#9929=CARTESIAN_POINT('Ctrl Pts',(81.1868156697076,24.3605622630378,-9.01941559002447));
#9930=CARTESIAN_POINT('Ctrl Pts',(82.7997191606577,25.4203430963022,-9.11172730376366));
#9931=CARTESIAN_POINT('Ctrl Pts',(84.9247819088485,24.4810090214786,-9.22286042175521));
#9932=CARTESIAN_POINT('Ctrl Pts',(85.2882084953573,22.1861971982837,-9.33399353974677));
#9933=CARTESIAN_POINT('Ctrl Pts',(83.5573766039194,20.6362097301691,-9.44512665773833));
#9934=CARTESIAN_POINT('Ctrl Pts',(81.4607076296431,21.2101562866457,-9.54910390466863));
#9935=CARTESIAN_POINT('Ctrl Pts',(80.9494318329284,22.4512689686606,-9.61603677893508));
#9936=CARTESIAN_POINT('Ctrl Pts',(80.944392795472,23.0017938245641,-9.64592528053768));
#9937=CARTESIAN_POINT('Origin',(83.,23.,-4.45407471946233));
#9938=CARTESIAN_POINT('',(80.944726360752,22.998158663221,-8.24592528053768));
#9939=CARTESIAN_POINT('',(80.9455227171961,23.0018771067991,-8.30407471946232));
#9940=CARTESIAN_POINT('',(80.94525,23.0000000000001,-4.45407471946233));
#9941=CARTESIAN_POINT('Ctrl Pts',(80.9455227171961,23.0018771067991,-8.30407471946232));
#9942=CARTESIAN_POINT('Ctrl Pts',(80.9439882359492,23.1712174130647,-8.31325541186101));
#9943=CARTESIAN_POINT('Ctrl Pts',(81.0405828044266,24.0221240109118,-8.35948047692355));
#9944=CARTESIAN_POINT('Ctrl Pts',(82.2221040357635,25.3006631740422,-8.44274991464995));
#9945=CARTESIAN_POINT('Ctrl Pts',(84.5109477713164,24.9013705599747,-8.55388303264151));
#9946=CARTESIAN_POINT('Ctrl Pts',(85.4169126362828,22.7618687715364,-8.66501615063307));
#9947=CARTESIAN_POINT('Ctrl Pts',(84.1108239277452,20.8403140564757,-8.77614926862462));
#9948=CARTESIAN_POINT('Ctrl Pts',(81.7880654389434,20.8953889211715,-8.88728238661619));
#9949=CARTESIAN_POINT('Ctrl Pts',(80.958434142698,22.2498852031596,-8.96325753689542));
#9950=CARTESIAN_POINT('Ctrl Pts',(80.9419424134073,22.9647236139308,-9.0021883145108));
#9951=CARTESIAN_POINT('Ctrl Pts',(80.9420824460358,22.9993679634637,-9.00407471946233));
#9952=CARTESIAN_POINT('Ctrl Pts',(80.944726360752,22.998158663221,-8.24592528053768));
#9953=CARTESIAN_POINT('Ctrl Pts',(80.9497076461214,23.5378860633926,-8.27521534629936));
#9954=CARTESIAN_POINT('Ctrl Pts',(81.444078523515,24.7683045917449,-8.3415497847249));
#9955=CARTESIAN_POINT('Ctrl Pts',(83.5192142474232,25.3724648971313,-8.44492859581431));
#9956=CARTESIAN_POINT('Ctrl Pts',(85.2747978255561,23.850569204887,-8.55606171380586));
#9957=CARTESIAN_POINT('Ctrl Pts',(84.9483968969088,21.5501991003249,-8.66719483179741));
#9958=CARTESIAN_POINT('Ctrl Pts',(82.8387464408891,20.5767438417137,-8.77832794978898));
#9959=CARTESIAN_POINT('Ctrl Pts',(81.1984096789596,21.6170977740004,-8.87123809936906));
#9960=CARTESIAN_POINT('Ctrl Pts',(80.9487183577381,22.6516188786005,-8.92710387628529));
#9961=CARTESIAN_POINT('Ctrl Pts',(80.9485808590134,23.0000908847555,-8.94592528053767));
#9962=CARTESIAN_POINT('Origin',(83.,23.,-4.45407471946233));
#9963=CARTESIAN_POINT('',(80.9425253333126,23.001059282702,-7.54592528053768));
#9964=CARTESIAN_POINT('',(80.948463814507,22.9994822145756,-7.60407471946232));
#9965=CARTESIAN_POINT('',(80.94525,23.0000000000001,-4.45407471946233));
#9966=CARTESIAN_POINT('Ctrl Pts',(80.948463814507,22.9994822145757,-7.60407471946232));
#9967=CARTESIAN_POINT('Ctrl Pts',(80.9493091967327,23.3743099216938,-7.62432250921123));
#9968=CARTESIAN_POINT('Ctrl Pts',(81.2270644273999,24.4360706544673,-7.68161467162399));
#9969=CARTESIAN_POINT('Ctrl Pts',(82.9319188372278,25.4276610173216,-7.7759512067006));
#9970=CARTESIAN_POINT('Ctrl Pts',(85.0026324571524,24.3739128224606,-7.88708432469215));
#9971=CARTESIAN_POINT('Ctrl Pts',(85.2404580324118,22.0627054938917,-7.99821744268371));
#9972=CARTESIAN_POINT('Ctrl Pts',(83.427728231352,20.6093470098792,-8.10935056067528));
#9973=CARTESIAN_POINT('Ctrl Pts',(81.4056136835162,21.283317959634,-8.21130298626814));
#9974=CARTESIAN_POINT('Ctrl Pts',(80.9501799143854,22.4879241340947,-8.27621103919716));
#9975=CARTESIAN_POINT('Ctrl Pts',(80.9455227171961,23.0018771067991,-8.30407471946232));
#9976=CARTESIAN_POINT('Ctrl Pts',(80.9425253333126,23.001059282702,-7.54592528053768));
#9977=CARTESIAN_POINT('Ctrl Pts',(80.9421429357283,23.0619343498909,-7.54923807098573));
#9978=CARTESIAN_POINT('Ctrl Pts',(80.9722035152768,23.8031452401182,-7.58959523409763));
#9979=CARTESIAN_POINT('Ctrl Pts',(81.8697768675109,25.1495971491679,-7.66699676987337));
#9980=CARTESIAN_POINT('Ctrl Pts',(84.1929368847996,25.1154372776465,-7.77812988786495));
#9981=CARTESIAN_POINT('Ctrl Pts',(85.4242743200689,23.1451456867025,-7.8892630058565));
#9982=CARTESIAN_POINT('Ctrl Pts',(84.4368203745666,21.042011180836,-8.00039612384806));
#9983=CARTESIAN_POINT('Ctrl Pts',(82.1343319219779,20.7309050425608,-8.11152924183962));
#9984=CARTESIAN_POINT('Ctrl Pts',(81.022161499857,22.031209731433,-8.1933722940695));
#9985=CARTESIAN_POINT('Ctrl Pts',(80.9434076059279,22.8552702197982,-8.23817097363551));
#9986=CARTESIAN_POINT('Ctrl Pts',(80.944726360752,22.998158663221,-8.24592528053768));
#9987=CARTESIAN_POINT('Origin',(83.,23.,-4.45407471946233));
#9988=CARTESIAN_POINT('',(80.9479086080167,23.0011644845222,-6.84592528053768));
#9989=CARTESIAN_POINT('',(80.943624771683,22.9983937941554,-6.90407471946232));
#9990=CARTESIAN_POINT('',(80.94525,23.0000000000001,-4.45407471946233));
#9991=CARTESIAN_POINT('Ctrl Pts',(80.943624771683,22.9983937941554,-6.90407471946232));
#9992=CARTESIAN_POINT('Ctrl Pts',(80.9485745341384,23.5746341161542,-6.93538960656144));
#9993=CARTESIAN_POINT('Ctrl Pts',(81.5015293092438,24.8408721637681,-7.00374886632442));
#9994=CARTESIAN_POINT('Ctrl Pts',(83.6477355735556,25.340642018176,-7.10915249875124));
#9995=CARTESIAN_POINT('Ctrl Pts',(85.3177709360927,23.7253357071464,-7.2202856167428));
#9996=CARTESIAN_POINT('Ctrl Pts',(84.8664912980158,21.4461709704268,-7.33141873473436));
#9997=CARTESIAN_POINT('Ctrl Pts',(82.706925266015,20.5891330421716,-7.44255185272592));
#9998=CARTESIAN_POINT('Ctrl Pts',(81.1601822794663,21.6927472756777,-7.53343718096857));
#9999=CARTESIAN_POINT('Ctrl Pts',(80.9477625264739,22.6885433546059,-7.58727813654738));
#10000=CARTESIAN_POINT('Ctrl Pts',(80.948463814507,22.9994822145757,-7.60407471946232));
#10001=CARTESIAN_POINT('Ctrl Pts',(80.9479086080167,23.0011644845222,-6.84592528053768));
#10002=CARTESIAN_POINT('Ctrl Pts',(80.9465286190407,23.2671876353822,-6.86030516833594));
#10003=CARTESIAN_POINT('Ctrl Pts',(81.1181884210441,24.2168118526317,-6.91172942879806));
#10004=CARTESIAN_POINT('Ctrl Pts',(82.5507725952567,25.3866959940047,-7.00019806192404));
#10005=CARTESIAN_POINT('Ctrl Pts',(84.7614901796242,24.6719233964163,-7.11133117991558));
#10006=CARTESIAN_POINT('Ctrl Pts',(85.3600357402078,22.4269243306697,-7.22246429790715));
#10007=CARTESIAN_POINT('Ctrl Pts',(83.7985771227055,20.7064348813032,-7.33359741589871));
#10008=CARTESIAN_POINT('Ctrl Pts',(81.5745655688421,21.0738146077992,-7.44141774344221));
#10009=CARTESIAN_POINT('Ctrl Pts',(80.9464189920752,22.381215569078,-7.51219369832188));
#10010=CARTESIAN_POINT('Ctrl Pts',(80.9425253333126,23.001059282702,-7.54592528053768));
#10011=CARTESIAN_POINT('Origin',(83.,23.,-4.45407471946233));
#10012=CARTESIAN_POINT('',(80.9473274657881,22.9976809234163,-6.14592528053767));
#10013=CARTESIAN_POINT('',(80.9434277056327,23.0014963838888,-6.20407471946233));
#10014=CARTESIAN_POINT('',(80.94525,23.0000000000001,-4.45407471946233));
#10015=CARTESIAN_POINT('',(82.4698297828114,21.0148256743283,-6.));
#10016=CARTESIAN_POINT('Ctrl Pts',(82.4698297828114,21.0148256743283,-6.));
#10017=CARTESIAN_POINT('Ctrl Pts',(81.8097404375819,21.1911123142463,-6.03704437266385));
#10018=CARTESIAN_POINT('Ctrl Pts',(81.0750709872232,21.8872127590751,-6.08568613284308));
#10019=CARTESIAN_POINT('Ctrl Pts',(80.9457104606,22.7834123400653,-6.1343278930223));
#10020=CARTESIAN_POINT('Ctrl Pts',(80.9473274657881,22.9976809234163,-6.14592528053767));
#10021=CARTESIAN_POINT('',(83.531311299962,21.0112683144402,-6.));
#10022=CARTESIAN_POINT('Origin',(83.,23.,-6.));
#10023=CARTESIAN_POINT('Ctrl Pts',(83.5313119958266,21.0112661450614,-6.));
#10024=CARTESIAN_POINT('Ctrl Pts',(82.8867917747511,20.8399706654375,-6.03631814560907));
#10025=CARTESIAN_POINT('Ctrl Pts',(81.5070301779678,21.1592646346911,-6.1043430520965));
#10026=CARTESIAN_POINT('Ctrl Pts',(80.9482804526145,22.418323940505,-6.17236795858395));
#10027=CARTESIAN_POINT('Ctrl Pts',(80.9434277056327,23.0014963838888,-6.20407471946233));
#10028=CARTESIAN_POINT('Origin',(83.,-23.,-12.));
#10029=CARTESIAN_POINT('',(81.3313535412238,-23.0003916921662,-16.2285196366098));
#10030=CARTESIAN_POINT('',(81.3334663482475,-22.9985217515097,-16.4214803633902));
#10031=CARTESIAN_POINT('',(81.334,-23.,-12.));
#10032=CARTESIAN_POINT('',(82.2300979593295,-24.4774325188554,-17.));
#10033=CARTESIAN_POINT('Ctrl Pts',(81.3334663482475,-22.9985217515097,-16.4214803633902));
#10034=CARTESIAN_POINT('Ctrl Pts',(81.3324167011274,-22.8847143817383,-16.4290983789409));
#10035=CARTESIAN_POINT('Ctrl Pts',(81.3430833954876,-22.7711019357605,-16.4367163944915));
#10036=CARTESIAN_POINT('Ctrl Pts',(81.3661911854064,-22.660076333029,-16.4443344100422));
#10037=CARTESIAN_POINT('Ctrl Pts',(81.4785581890567,-22.1201885137589,-16.4813787827061));
#10038=CARTESIAN_POINT('Ctrl Pts',(81.885109434169,-21.6414696256838,-16.5184231553699));
#10039=CARTESIAN_POINT('Ctrl Pts',(82.3995342859918,-21.4430319247283,-16.5554675280338));
#10040=CARTESIAN_POINT('Ctrl Pts',(82.9139591378146,-21.2445942237728,-16.5925119006976));
#10041=CARTESIAN_POINT('Ctrl Pts',(83.5362575963479,-21.3264377099369,-16.6295562733615));
#10042=CARTESIAN_POINT('Ctrl Pts',(83.9821833263623,-21.6510262177334,-16.6666006460253));
#10043=CARTESIAN_POINT('Ctrl Pts',(84.4281090563767,-21.9756147255299,-16.7036450186892));
#10044=CARTESIAN_POINT('Ctrl Pts',(84.6976620578723,-22.5429482549589,-16.740689391353));
#10045=CARTESIAN_POINT('Ctrl Pts',(84.6664136178775,-23.09358162467,-16.7777337640169));
#10046=CARTESIAN_POINT('Ctrl Pts',(84.6351651778828,-23.6442149943811,-16.8147781366807));
#10047=CARTESIAN_POINT('Ctrl Pts',(84.3031152963976,-24.1781482043742,-16.8518225093446));
#10048=CARTESIAN_POINT('Ctrl Pts',(83.8246635830312,-24.4504525233503,-16.8888668820084));
#10049=CARTESIAN_POINT('Ctrl Pts',(83.3462118696648,-24.7227568423263,-16.9259112546723));
#10050=CARTESIAN_POINT('Ctrl Pts',(82.7213583244172,-24.7334322702853,-16.9629556273362));
#10051=CARTESIAN_POINT('Ctrl Pts',(82.2300979593296,-24.4774325188554,-17.));
#10052=CARTESIAN_POINT('',(81.662974037086,-22.0009968623267,-17.));
#10053=CARTESIAN_POINT('Origin',(83.,-23.,-17.));
#10054=CARTESIAN_POINT('',(81.3354783154905,-23.001221079894,-16.9285196366098));
#10055=CARTESIAN_POINT('Ctrl Pts',(81.6629726161761,-22.000995687242,-17.));
#10056=CARTESIAN_POINT('Ctrl Pts',(81.4510074599991,-22.2854498000758,-16.9761732122033));
#10057=CARTESIAN_POINT('Ctrl Pts',(81.3378311424635,-22.644062616804,-16.9523464244065));
#10058=CARTESIAN_POINT('Ctrl Pts',(81.3354783154905,-23.001221079894,-16.9285196366098));
#10059=CARTESIAN_POINT('',(81.334,-23.,-18.));
#10060=CARTESIAN_POINT('',(81.334,-23.,-12.));
#10061=CARTESIAN_POINT('Origin',(83.,-23.,-18.));
#10062=CARTESIAN_POINT('Ctrl Pts',(81.3354783154905,-23.001221079894,-16.9285196366098));
#10063=CARTESIAN_POINT('Ctrl Pts',(81.3342448297249,-23.1884638671393,-16.9160282787975));
#10064=CARTESIAN_POINT('Ctrl Pts',(81.3634706586964,-23.3753069321328,-16.9035369209851));
#10065=CARTESIAN_POINT('Ctrl Pts',(81.4248898698669,-23.5508552241813,-16.8910455631728));
#10066=CARTESIAN_POINT('Ctrl Pts',(81.6070346920316,-24.0714612662822,-16.8540011905089));
#10067=CARTESIAN_POINT('Ctrl Pts',(82.0723133658506,-24.492732216851,-16.8169568178451));
#10068=CARTESIAN_POINT('Ctrl Pts',(82.6082885283144,-24.6221191089392,-16.7799124451812));
#10069=CARTESIAN_POINT('Ctrl Pts',(83.1442636907781,-24.7515060010274,-16.7428680725174));
#10070=CARTESIAN_POINT('Ctrl Pts',(83.7509353418865,-24.589008834635,-16.7058236998535));
#10071=CARTESIAN_POINT('Ctrl Pts',(84.1504371851532,-24.2088727275756,-16.6687793271897));
#10072=CARTESIAN_POINT('Ctrl Pts',(84.5499390284198,-23.8287366205161,-16.6317349545258));
#10073=CARTESIAN_POINT('Ctrl Pts',(84.7422710638447,-23.2309615727897,-16.594690581862));
#10074=CARTESIAN_POINT('Ctrl Pts',(84.6395393530548,-22.6891597720865,-16.5576462091981));
#10075=CARTESIAN_POINT('Ctrl Pts',(84.536807642265,-22.1473579713834,-16.5206018365343));
#10076=CARTESIAN_POINT('Ctrl Pts',(84.1390121852604,-21.6615294177034,-16.4835574638704));
#10077=CARTESIAN_POINT('Ctrl Pts',(83.6281313466739,-21.4539694514453,-16.4465130912065));
#10078=CARTESIAN_POINT('Ctrl Pts',(83.1172505080875,-21.2464094851871,-16.4094687185427));
#10079=CARTESIAN_POINT('Ctrl Pts',(82.4932842879192,-21.3171181063508,-16.3724243458788));
#10080=CARTESIAN_POINT('Ctrl Pts',(82.0418023292256,-21.6337523848716,-16.335379973215));
#10081=CARTESIAN_POINT('Ctrl Pts',(81.6076786858952,-21.9382128930889,-16.2997598610133));
#10082=CARTESIAN_POINT('Ctrl Pts',(81.3330311221208,-22.4700521740837,-16.2641397488115));
#10083=CARTESIAN_POINT('Ctrl Pts',(81.3313535412238,-23.0003916921662,-16.2285196366098));
#10084=CARTESIAN_POINT('Origin',(83.,-23.,-12.));
#10085=CARTESIAN_POINT('',(81.3344265803655,-22.9984874575686,-15.5285196366098));
#10086=CARTESIAN_POINT('',(81.3367022463126,-23.0000402080689,-15.7214803633902));
#10087=CARTESIAN_POINT('',(81.334,-23.,-12.));
#10088=CARTESIAN_POINT('Ctrl Pts',(81.3367022463126,-23.0000402080689,-15.7214803633902));
#10089=CARTESIAN_POINT('Ctrl Pts',(81.3367622607545,-22.7195427638815,-15.7401654762911));
#10090=CARTESIAN_POINT('Ctrl Pts',(81.403932944649,-22.4390181888952,-15.758850589192));
#10091=CARTESIAN_POINT('Ctrl Pts',(81.5380528521339,-22.1953422621795,-15.7775357020929));
#10092=CARTESIAN_POINT('Ctrl Pts',(81.8039537252442,-21.7122399182789,-15.8145800747567));
#10093=CARTESIAN_POINT('Ctrl Pts',(82.3330016941159,-21.373972932507,-15.8516244474206));
#10094=CARTESIAN_POINT('Ctrl Pts',(82.8830897925016,-21.3353395855451,-15.8886688200844));
#10095=CARTESIAN_POINT('Ctrl Pts',(83.4331778908874,-21.2967062385831,-15.9257131927483));
#10096=CARTESIAN_POINT('Ctrl Pts',(84.0043061187875,-21.5577065304311,-15.9627575654121));
#10097=CARTESIAN_POINT('Ctrl Pts',(84.33512334448,-21.9989002927704,-15.999801938076));
#10098=CARTESIAN_POINT('Ctrl Pts',(84.6659405701726,-22.4400940551098,-16.0368463107398));
#10099=CARTESIAN_POINT('Ctrl Pts',(84.7564467936577,-23.0614812879405,-16.0738906834037));
#10100=CARTESIAN_POINT('Ctrl Pts',(84.5652078620693,-23.5787055542428,-16.1109350560675));
#10101=CARTESIAN_POINT('Ctrl Pts',(84.3739689304809,-24.0959298205451,-16.1479794287314));
#10102=CARTESIAN_POINT('Ctrl Pts',(83.9009848438189,-24.508991120319,-16.1850238013952));
#10103=CARTESIAN_POINT('Ctrl Pts',(83.3627357838583,-24.6288593090619,-16.2220681740591));
#10104=CARTESIAN_POINT('Ctrl Pts',(82.8244867238977,-24.7487274978049,-16.2591125467229));
#10105=CARTESIAN_POINT('Ctrl Pts',(82.2209726906385,-24.575402575517,-16.2961569193868));
#10106=CARTESIAN_POINT('Ctrl Pts',(81.828307055103,-24.1882117391405,-16.3332012920507));
#10107=CARTESIAN_POINT('Ctrl Pts',(81.5163914148467,-23.8806450291963,-16.3626276491638));
#10108=CARTESIAN_POINT('Ctrl Pts',(81.3375208544104,-23.4381291903146,-16.392054006277));
#10109=CARTESIAN_POINT('Ctrl Pts',(81.3334663482475,-22.9985217515097,-16.4214803633902));
#10110=CARTESIAN_POINT('Ctrl Pts',(81.3313535412238,-23.0003916921662,-16.2285196366098));
#10111=CARTESIAN_POINT('Ctrl Pts',(81.3312864636096,-23.0215971730145,-16.2270953761477));
#10112=CARTESIAN_POINT('Ctrl Pts',(81.3316558045061,-23.0428002560741,-16.2256711156856));
#10113=CARTESIAN_POINT('Ctrl Pts',(81.3324688192059,-23.0639863098917,-16.2242468552234));
#10114=CARTESIAN_POINT('Ctrl Pts',(81.3536149650986,-23.6150260205131,-16.1872024825596));
#10115=CARTESIAN_POINT('Ctrl Pts',(81.6749049541029,-24.1545455058778,-16.1501581098957));
#10116=CARTESIAN_POINT('Ctrl Pts',(82.1493178143438,-24.4356537351314,-16.1131137372319));
#10117=CARTESIAN_POINT('Ctrl Pts',(82.6237306745847,-24.716761964385,-16.076069364568));
#10118=CARTESIAN_POINT('Ctrl Pts',(83.2512664060623,-24.7394589375276,-16.0390249919042));
#10119=CARTESIAN_POINT('Ctrl Pts',(83.7447484720246,-24.4933562158936,-16.0019806192403));
#10120=CARTESIAN_POINT('Ctrl Pts',(84.2382305379868,-24.2472534942596,-15.9649362465765));
#10121=CARTESIAN_POINT('Ctrl Pts',(84.5976589384339,-23.7323510778492,-15.9278918739126));
#10122=CARTESIAN_POINT('Ctrl Pts',(84.6585540875959,-23.1842793768616,-15.8908475012488));
#10123=CARTESIAN_POINT('Ctrl Pts',(84.7194492367579,-22.6362076758741,-15.8538031285849));
#10124=CARTESIAN_POINT('Ctrl Pts',(84.4818111346349,-22.0549666903095,-15.8167587559211));
#10125=CARTESIAN_POINT('Ctrl Pts',(84.0543866887268,-21.706543266871,-15.7797143832572));
#10126=CARTESIAN_POINT('Ctrl Pts',(83.6269622428187,-21.3581198434324,-15.7426700105933));
#10127=CARTESIAN_POINT('Ctrl Pts',(83.0097514531255,-21.2425139821199,-15.7056256379295));
#10128=CARTESIAN_POINT('Ctrl Pts',(82.4852026073696,-21.4126294343583,-15.6685812652656));
#10129=CARTESIAN_POINT('Ctrl Pts',(81.9606537616137,-21.5827448865967,-15.6315368926018));
#10130=CARTESIAN_POINT('Ctrl Pts',(81.5287668597951,-22.0385816523861,-15.5944925199379));
#10131=CARTESIAN_POINT('Ctrl Pts',(81.3871816050425,-22.5715397394835,-15.5574481472741));
#10132=CARTESIAN_POINT('Ctrl Pts',(81.3503262497169,-22.7102714153768,-15.547805310386));
#10133=CARTESIAN_POINT('Ctrl Pts',(81.3331413605435,-22.8542287327907,-15.5381624734979));
#10134=CARTESIAN_POINT('Ctrl Pts',(81.3344265803655,-22.9984874575686,-15.5285196366098));
#10135=CARTESIAN_POINT('Origin',(83.,-23.,-12.));
#10136=CARTESIAN_POINT('',(81.3365469135995,-23.0005281518415,-14.8285196366098));
#10137=CARTESIAN_POINT('',(81.3333662687744,-23.0014645813323,-15.0214803633902));
#10138=CARTESIAN_POINT('',(81.334,-23.,-12.));
#10139=CARTESIAN_POINT('Ctrl Pts',(81.3333662687744,-23.0014645813323,-15.0214803633902));
#10140=CARTESIAN_POINT('Ctrl Pts',(81.3374449537321,-22.5570899997421,-15.0512325736413));
#10141=CARTESIAN_POINT('Ctrl Pts',(81.5206881577281,-22.1097458291912,-15.0809847838924));
#10142=CARTESIAN_POINT('Ctrl Pts',(81.8387594570367,-21.8015500092252,-15.1107369941435));
#10143=CARTESIAN_POINT('Ctrl Pts',(82.2347889165566,-21.4178164744086,-15.1477813668074));
#10144=CARTESIAN_POINT('Ctrl Pts',(82.839837690827,-21.249799796086,-15.1848257394712));
#10145=CARTESIAN_POINT('Ctrl Pts',(83.3770234867105,-21.3743877231352,-15.2218701121351));
#10146=CARTESIAN_POINT('Ctrl Pts',(83.914209282594,-21.4989756501844,-15.2589144847989));
#10147=CARTESIAN_POINT('Ctrl Pts',(84.3835321000906,-21.9161681826054,-15.2959588574628));
#10148=CARTESIAN_POINT('Ctrl Pts',(84.5702207149372,-22.4350497866678,-15.3330032301266));
#10149=CARTESIAN_POINT('Ctrl Pts',(84.7569093297838,-22.9539313907302,-15.3700476027905));
#10150=CARTESIAN_POINT('Ctrl Pts',(84.6609637419804,-23.5745020664339,-15.4070919754543));
#10151=CARTESIAN_POINT('Ctrl Pts',(84.3262902750188,-24.0127765010024,-15.4441363481182));
#10152=CARTESIAN_POINT('Ctrl Pts',(83.9916168080572,-24.4510509355709,-15.481180720782));
#10153=CARTESIAN_POINT('Ctrl Pts',(83.4182154619373,-24.7070291290041,-15.5182250934459));
#10154=CARTESIAN_POINT('Ctrl Pts',(82.8684865069619,-24.6635703403376,-15.5552694661097));
#10155=CARTESIAN_POINT('Ctrl Pts',(82.3187575519866,-24.6201115516712,-15.5923138387736));
#10156=CARTESIAN_POINT('Ctrl Pts',(81.7927009881558,-24.2772157809052,-15.6293582114374));
#10157=CARTESIAN_POINT('Ctrl Pts',(81.5310495949151,-23.7917990445074,-15.6664025841013));
#10158=CARTESIAN_POINT('Ctrl Pts',(81.4013746793903,-23.5512256101106,-15.6847618438643));
#10159=CARTESIAN_POINT('Ctrl Pts',(81.3366432784737,-23.2756460054758,-15.7031211036272));
#10160=CARTESIAN_POINT('Ctrl Pts',(81.3367022463126,-23.0000402080689,-15.7214803633902));
#10161=CARTESIAN_POINT('Ctrl Pts',(81.3344265803655,-22.9984874575686,-15.5285196366098));
#10162=CARTESIAN_POINT('Ctrl Pts',(81.3380787210521,-23.4084197890849,-15.501118100834));
#10163=CARTESIAN_POINT('Ctrl Pts',(81.4908761802709,-23.820785971822,-15.4737165650583));
#10164=CARTESIAN_POINT('Ctrl Pts',(81.7652753558034,-24.1225936800591,-15.4463150292825));
#10165=CARTESIAN_POINT('Ctrl Pts',(82.1362379690038,-24.5306101251318,-15.4092706566187));
#10166=CARTESIAN_POINT('Ctrl Pts',(82.7294468030913,-24.7365636068717,-15.3722262839548));
#10167=CARTESIAN_POINT('Ctrl Pts',(83.2734377603458,-24.6462057293775,-15.335181911291));
#10168=CARTESIAN_POINT('Ctrl Pts',(83.8174287176003,-24.5558478518833,-15.2981375386271));
#10169=CARTESIAN_POINT('Ctrl Pts',(84.3122017980218,-24.1691786151549,-15.2610931659633));
#10170=CARTESIAN_POINT('Ctrl Pts',(84.5313391335624,-23.6631454863052,-15.2240487932994));
#10171=CARTESIAN_POINT('Ctrl Pts',(84.7504764691031,-23.1571123574555,-15.1870044206356));
#10172=CARTESIAN_POINT('Ctrl Pts',(84.6939780597629,-22.5317153364845,-15.1499600479717));
#10173=CARTESIAN_POINT('Ctrl Pts',(84.3876986741927,-22.0731484004554,-15.1129156753078));
#10174=CARTESIAN_POINT('Ctrl Pts',(84.0814192886225,-21.6145814644263,-15.075871302644));
#10175=CARTESIAN_POINT('Ctrl Pts',(83.5253589268223,-21.3228446133391,-15.0388269299802));
#10176=CARTESIAN_POINT('Ctrl Pts',(82.9739817612062,-21.3314423753008,-15.0017825573163));
#10177=CARTESIAN_POINT('Ctrl Pts',(82.4226045955901,-21.3400401372625,-14.9647381846524));
#10178=CARTESIAN_POINT('Ctrl Pts',(81.8759106261582,-21.6489725122731,-14.9276938119886));
#10179=CARTESIAN_POINT('Ctrl Pts',(81.5840777682971,-22.1168659639303,-14.8906494393247));
#10180=CARTESIAN_POINT('Ctrl Pts',(81.4209264214049,-22.3784453056102,-14.8699395050864));
#10181=CARTESIAN_POINT('Ctrl Pts',(81.3374307130897,-22.6897071821857,-14.8492295708481));
#10182=CARTESIAN_POINT('Ctrl Pts',(81.3365469135995,-23.0005281518415,-14.8285196366098));
#10183=CARTESIAN_POINT('Origin',(83.,-23.,-12.));
#10184=CARTESIAN_POINT('',(81.3324918741766,-23.0012330300494,-14.1285196366098));
#10185=CARTESIAN_POINT('',(81.3319380386485,-22.9990409236778,-14.3214803633902));
#10186=CARTESIAN_POINT('',(81.334,-23.,-12.));
#10187=CARTESIAN_POINT('Ctrl Pts',(81.3319380386485,-22.9990409236778,-14.3214803633902));
#10188=CARTESIAN_POINT('Ctrl Pts',(81.3315519386774,-22.9427845253567,-14.3252552983277));
#10189=CARTESIAN_POINT('Ctrl Pts',(81.3341512567505,-22.8865642275187,-14.3290302332651));
#10190=CARTESIAN_POINT('Ctrl Pts',(81.3398535979727,-22.8306604466783,-14.3328051682026));
#10191=CARTESIAN_POINT('Ctrl Pts',(81.3958120864737,-22.2820627820619,-14.3698495408664));
#10192=CARTESIAN_POINT('Ctrl Pts',(81.750591195306,-21.7639456524137,-14.4068939135303));
#10193=CARTESIAN_POINT('Ctrl Pts',(82.241837022815,-21.5134096526244,-14.4439382861942));
#10194=CARTESIAN_POINT('Ctrl Pts',(82.733082850324,-21.262873652835,-14.480982658858));
#10195=CARTESIAN_POINT('Ctrl Pts',(83.3607953965097,-21.2799187829043,-14.5180270315219));
#10196=CARTESIAN_POINT('Ctrl Pts',(83.837721045914,-21.556744856032,-14.5550714041857));
#10197=CARTESIAN_POINT('Ctrl Pts',(84.3146466953183,-21.8335709291597,-14.5921157768496));
#10198=CARTESIAN_POINT('Ctrl Pts',(84.6407854479411,-22.3701779453458,-14.6291601495134));
#10199=CARTESIAN_POINT('Ctrl Pts',(84.6668897943504,-22.9210039733326,-14.6662045221773));
#10200=CARTESIAN_POINT('Ctrl Pts',(84.6929941407597,-23.4718300013195,-14.7032488948411));
#10201=CARTESIAN_POINT('Ctrl Pts',(84.4190640809555,-24.0368750411072,-14.740293267505));
#10202=CARTESIAN_POINT('Ctrl Pts',(83.9704553969745,-24.3575633631643,-14.7773376401688));
#10203=CARTESIAN_POINT('Ctrl Pts',(83.5218467129935,-24.6782516852214,-14.8143820128327));
#10204=CARTESIAN_POINT('Ctrl Pts',(82.8985594048357,-24.754583289548,-14.8514263854965));
#10205=CARTESIAN_POINT('Ctrl Pts',(82.3858220193069,-24.5516273305094,-14.8884707581604));
#10206=CARTESIAN_POINT('Ctrl Pts',(81.873084633778,-24.3486713714708,-14.9255151308242));
#10207=CARTESIAN_POINT('Ctrl Pts',(81.4708971708781,-23.8664278490671,-14.9625595034881));
#10208=CARTESIAN_POINT('Ctrl Pts',(81.3633085118128,-23.3255808922099,-14.9996038761519));
#10209=CARTESIAN_POINT('Ctrl Pts',(81.342129749176,-23.2191154950054,-15.0068960385647));
#10210=CARTESIAN_POINT('Ctrl Pts',(81.3323665973923,-23.1103792331753,-15.0141882009775));
#10211=CARTESIAN_POINT('Ctrl Pts',(81.3333662687744,-23.0014645813323,-15.0214803633902));
#10212=CARTESIAN_POINT('Ctrl Pts',(81.3365469135995,-23.0005281518415,-14.8285196366098));
#10213=CARTESIAN_POINT('Ctrl Pts',(81.3358498390368,-23.2456803542478,-14.8121851981843));
#10214=CARTESIAN_POINT('Ctrl Pts',(81.3865445413348,-23.4905582742853,-14.7958507597587));
#10215=CARTESIAN_POINT('Ctrl Pts',(81.4900815300601,-23.7105685812494,-14.7795163213332));
#10216=CARTESIAN_POINT('Ctrl Pts',(81.7248898959745,-24.2095232186075,-14.7424719486693));
#10217=CARTESIAN_POINT('Ctrl Pts',(82.2314783740936,-24.5805779650201,-14.7054275760055));
#10218=CARTESIAN_POINT('Ctrl Pts',(82.778022106296,-24.6539308657728,-14.6683832033416));
#10219=CARTESIAN_POINT('Ctrl Pts',(83.3245658384983,-24.7272837665254,-14.6313388306778));
#10220=CARTESIAN_POINT('Ctrl Pts',(83.9110648247838,-24.5029348216182,-14.5942944580139));
#10221=CARTESIAN_POINT('Ctrl Pts',(84.2691255873272,-24.0835505236204,-14.55725008535));
#10222=CARTESIAN_POINT('Ctrl Pts',(84.6271863498705,-23.6641662256226,-14.5202057126862));
#10223=CARTESIAN_POINT('Ctrl Pts',(84.7568088886717,-23.0497465745342,-14.4831613400223));
#10224=CARTESIAN_POINT('Ctrl Pts',(84.5986753787846,-22.521462094236,-14.4461169673585));
#10225=CARTESIAN_POINT('Ctrl Pts',(84.4405418688976,-21.9931776139378,-14.4090725946946));
#10226=CARTESIAN_POINT('Ctrl Pts',(83.9946523103222,-21.5510283044299,-14.3720282220308));
#10227=CARTESIAN_POINT('Ctrl Pts',(83.465054540206,-21.3973503912159,-14.3349838493669));
#10228=CARTESIAN_POINT('Ctrl Pts',(82.9354567700899,-21.2436724780019,-14.2979394767031));
#10229=CARTESIAN_POINT('Ctrl Pts',(82.3221507884329,-21.3784659610818,-14.2608951040392));
#10230=CARTESIAN_POINT('Ctrl Pts',(81.9057974821241,-21.7400466898587,-14.2238507313754));
#10231=CARTESIAN_POINT('Ctrl Pts',(81.5486454718412,-22.0502142379612,-14.1920736997868));
#10232=CARTESIAN_POINT('Ctrl Pts',(81.3364187077672,-22.5272604403474,-14.1602966681983));
#10233=CARTESIAN_POINT('Ctrl Pts',(81.3324918741766,-23.0012330300494,-14.1285196366098));
#10234=CARTESIAN_POINT('Origin',(83.,-23.,-12.));
#10235=CARTESIAN_POINT('',(81.3327118147905,-22.9986896254657,-13.4285196366098));
#10236=CARTESIAN_POINT('',(81.3362661410155,-22.99914450019,-13.6214803633902));
#10237=CARTESIAN_POINT('',(81.334,-23.,-12.));
#10238=CARTESIAN_POINT('Ctrl Pts',(81.3362661410155,-22.99914450019,-13.6214803633902));
#10239=CARTESIAN_POINT('Ctrl Pts',(81.3352300865187,-22.776484691814,-13.6363223956779));
#10240=CARTESIAN_POINT('Ctrl Pts',(81.376782632399,-22.5541957175097,-13.6511644279656));
#10241=CARTESIAN_POINT('Ctrl Pts',(81.4627522870129,-22.3506684747836,-13.6660064602532));
#10242=CARTESIAN_POINT('Ctrl Pts',(81.6773247836614,-21.8426828512073,-13.7030508329171));
#10243=CARTESIAN_POINT('Ctrl Pts',(82.1685965611403,-21.4515746602874,-13.7400952055809));
#10244=CARTESIAN_POINT('Ctrl Pts',(82.7117519859494,-21.3563227071218,-13.7771395782448));
#10245=CARTESIAN_POINT('Ctrl Pts',(83.2549074107585,-21.2610707539562,-13.8141839509087));
#10246=CARTESIAN_POINT('Ctrl Pts',(83.8499464828978,-21.4616750385448,-13.8512283235725));
#10247=CARTESIAN_POINT('Ctrl Pts',(84.2245676126847,-21.8663350924087,-13.8882726962364));
#10248=CARTESIAN_POINT('Ctrl Pts',(84.5991887424716,-22.2709951462725,-13.9253170689002));
#10249=CARTESIAN_POINT('Ctrl Pts',(84.7533919299061,-22.8797109694116,-13.9623614415641));
#10250=CARTESIAN_POINT('Ctrl Pts',(84.6166107617626,-23.4139222217417,-13.9994058142279));
#10251=CARTESIAN_POINT('Ctrl Pts',(84.479829593619,-23.9481334740717,-14.0364501868918));
#10252=CARTESIAN_POINT('Ctrl Pts',(84.0520640698975,-24.4078401555926,-14.0734945595556));
#10253=CARTESIAN_POINT('Ctrl Pts',(83.5290681125294,-24.5826714419116,-14.1105389322195));
#10254=CARTESIAN_POINT('Ctrl Pts',(83.0060721551613,-24.7575027282305,-14.1475833048833));
#10255=CARTESIAN_POINT('Ctrl Pts',(82.3878457641466,-24.6474586193474,-14.1846276775472));
#10256=CARTESIAN_POINT('Ctrl Pts',(81.9573015027242,-24.3028974651135,-14.221672050211));
#10257=CARTESIAN_POINT('Ctrl Pts',(81.5706310190902,-23.9934481469204,-14.2549414879374));
#10258=CARTESIAN_POINT('Ctrl Pts',(81.3353408334404,-23.4948425127546,-14.2882109256638));
#10259=CARTESIAN_POINT('Ctrl Pts',(81.3319380386485,-22.9990409236778,-14.3214803633902));
#10260=CARTESIAN_POINT('Ctrl Pts',(81.3324918741766,-23.0012330300494,-14.1285196366098));
#10261=CARTESIAN_POINT('Ctrl Pts',(81.3318409646726,-23.0797984329682,-14.1232522955345));
#10262=CARTESIAN_POINT('Ctrl Pts',(81.3369133399439,-23.1582793847753,-14.1179849544591));
#10263=CARTESIAN_POINT('Ctrl Pts',(81.3479976357627,-23.2359018492069,-14.1127176133838));
#10264=CARTESIAN_POINT('Ctrl Pts',(81.4259517266709,-23.7818083053044,-14.07567324072));
#10265=CARTESIAN_POINT('Ctrl Pts',(81.801260539448,-24.2852532430257,-14.0386288680561));
#10266=CARTESIAN_POINT('Ctrl Pts',(82.3021753753463,-24.5158503511622,-14.0015844953923));
#10267=CARTESIAN_POINT('Ctrl Pts',(82.8030902112445,-24.7464474592986,-13.9645401227284));
#10268=CARTESIAN_POINT('Ctrl Pts',(83.429611070264,-24.7041967378502,-13.9274957500646));
#10269=CARTESIAN_POINT('Ctrl Pts',(83.8950296775147,-24.4084329484417,-13.8904513774007));
#10270=CARTESIAN_POINT('Ctrl Pts',(84.3604482847654,-24.1126691590331,-13.8534070047368));
#10271=CARTESIAN_POINT('Ctrl Pts',(84.6647646402474,-23.5633923016643,-13.816362632073));
#10272=CARTESIAN_POINT('Ctrl Pts',(84.6687175908008,-23.0119622759285,-13.7793182594091));
#10273=CARTESIAN_POINT('Ctrl Pts',(84.6726705413541,-22.4605322501928,-13.7422738867453));
#10274=CARTESIAN_POINT('Ctrl Pts',(84.3762600869788,-21.9069490560902,-13.7052295140814));
#10275=CARTESIAN_POINT('Ctrl Pts',(83.9151294848998,-21.6045432576541,-13.6681851414176));
#10276=CARTESIAN_POINT('Ctrl Pts',(83.4539988828207,-21.302137459218,-13.6311407687537));
#10277=CARTESIAN_POINT('Ctrl Pts',(82.8281481330379,-21.2509090564484,-13.5940963960899));
#10278=CARTESIAN_POINT('Ctrl Pts',(82.3239788552738,-21.4743011746173,-13.557052023426));
#10279=CARTESIAN_POINT('Ctrl Pts',(81.8198095775097,-21.6976932927862,-13.5200076507622));
#10280=CARTESIAN_POINT('Ctrl Pts',(81.4373217717644,-22.1957059318936,-13.4829632780983));
#10281=CARTESIAN_POINT('Ctrl Pts',(81.3515493852339,-22.7404387074911,-13.4459189054345));
#10282=CARTESIAN_POINT('Ctrl Pts',(81.3381206536555,-22.825723383846,-13.4401191491596));
#10283=CARTESIAN_POINT('Ctrl Pts',(81.3319649476304,-22.9121532542978,-13.4343193928847));
#10284=CARTESIAN_POINT('Ctrl Pts',(81.3327118147905,-22.9986896254657,-13.4285196366098));
#10285=CARTESIAN_POINT('Origin',(83.,-23.,-12.));
#10286=CARTESIAN_POINT('',(81.3366136549425,-22.9995968836278,-12.7285196366098));
#10287=CARTESIAN_POINT('',(81.3350587862692,-23.0014219189523,-12.9214803633902));
#10288=CARTESIAN_POINT('',(81.334,-23.,-12.));
#10289=CARTESIAN_POINT('Ctrl Pts',(81.3350587862692,-23.0014219189523,-12.9214803633902));
#10290=CARTESIAN_POINT('Ctrl Pts',(81.3382109857955,-22.613442580851,-12.9473894930281));
#10291=CARTESIAN_POINT('Ctrl Pts',(81.4733906271644,-22.2234832157686,-12.973298622666));
#10292=CARTESIAN_POINT('Ctrl Pts',(81.7211701893928,-21.9279196502921,-12.9992077523039));
#10293=CARTESIAN_POINT('Ctrl Pts',(82.0754406172289,-21.5053285784039,-13.0362521249677));
#10294=CARTESIAN_POINT('Ctrl Pts',(82.6598959956844,-21.2757082679968,-13.0732964976316));
#10295=CARTESIAN_POINT('Ctrl Pts',(83.2070780416085,-21.3441374919967,-13.1103408702954));
#10296=CARTESIAN_POINT('Ctrl Pts',(83.7542600875325,-21.4125667159967,-13.1473852429593));
#10297=CARTESIAN_POINT('Ctrl Pts',(84.2641688009252,-21.7790454744038,-13.1844296156232));
#10298=CARTESIAN_POINT('Ctrl Pts',(84.5034599196319,-22.2758658751392,-13.221473988287));
#10299=CARTESIAN_POINT('Ctrl Pts',(84.7427510383386,-22.7726862758745,-13.2585183609509));
#10300=CARTESIAN_POINT('Ctrl Pts',(84.7114245623595,-23.3998483189383,-13.2955627336147));
#10301=CARTESIAN_POINT('Ctrl Pts',(84.4238161036021,-23.8703503109956,-13.3326071062786));
#10302=CARTESIAN_POINT('Ctrl Pts',(84.1362076448448,-24.340852303053,-13.3696514789424));
#10303=CARTESIAN_POINT('Ctrl Pts',(83.5923172033091,-24.6546942441039,-13.4066958516063));
#10304=CARTESIAN_POINT('Ctrl Pts',(83.0410397487005,-24.6682558855744,-13.4437402242701));
#10305=CARTESIAN_POINT('Ctrl Pts',(82.4897622940919,-24.681817527045,-13.480784596934));
#10306=CARTESIAN_POINT('Ctrl Pts',(81.9310978264102,-24.3950988689351,-13.5178289695978));
#10307=CARTESIAN_POINT('Ctrl Pts',(81.6207022004784,-23.9393080117639,-13.5548733422617));
#10308=CARTESIAN_POINT('Ctrl Pts',(81.4346682945799,-23.6661322761914,-13.5770756826379));
#10309=CARTESIAN_POINT('Ctrl Pts',(81.3378159850085,-23.3322234719803,-13.599278023014));
#10310=CARTESIAN_POINT('Ctrl Pts',(81.3362661410155,-22.99914450019,-13.6214803633902));
#10311=CARTESIAN_POINT('Ctrl Pts',(81.3327118147905,-22.9986896254657,-13.4285196366098));
#10312=CARTESIAN_POINT('Ctrl Pts',(81.3367353593684,-23.4648808915603,-13.3972750202208));
#10313=CARTESIAN_POINT('Ctrl Pts',(81.5410870292824,-23.9341630468355,-13.3660304038319));
#10314=CARTESIAN_POINT('Ctrl Pts',(81.887846800212,-24.2441369515021,-13.3347857874429));
#10315=CARTESIAN_POINT('Ctrl Pts',(82.2989735690362,-24.6116495078282,-13.297741414779));
#10316=CARTESIAN_POINT('Ctrl Pts',(82.9102840740004,-24.7552217083932,-13.2606970421152));
#10317=CARTESIAN_POINT('Ctrl Pts',(83.4420305975594,-24.6091520887451,-13.2236526694514));
#10318=CARTESIAN_POINT('Ctrl Pts',(83.9737771211185,-24.463082469097,-13.1866082967875));
#10319=CARTESIAN_POINT('Ctrl Pts',(84.4259596632723,-24.0273710292358,-13.1495639241236));
#10320=CARTESIAN_POINT('Ctrl Pts',(84.5916505938657,-23.5014078987596,-13.1125195514598));
#10321=CARTESIAN_POINT('Ctrl Pts',(84.757341524459,-22.9754447682834,-13.0754751787959));
#10322=CARTESIAN_POINT('Ctrl Pts',(84.636540843492,-22.3592299471921,-13.0384308061321));
#10323=CARTESIAN_POINT('Ctrl Pts',(84.2845293199092,-21.9347554646067,-13.0013864334682));
#10324=CARTESIAN_POINT('Ctrl Pts',(83.9325177963264,-21.5102809820213,-12.9643420608044));
#10325=CARTESIAN_POINT('Ctrl Pts',(83.3492954301278,-21.2775468379417,-12.9272976881405));
#10326=CARTESIAN_POINT('Ctrl Pts',(82.8017562537904,-21.3430567568621,-12.8902533154767));
#10327=CARTESIAN_POINT('Ctrl Pts',(82.2542170774529,-21.4085666757825,-12.8532089428128));
#10328=CARTESIAN_POINT('Ctrl Pts',(81.7423610909766,-21.7723206577029,-12.816164570149));
#10329=CARTESIAN_POINT('Ctrl Pts',(81.5004236670005,-22.2678577218878,-12.7791201974851));
#10330=CARTESIAN_POINT('Ctrl Pts',(81.3902659608985,-22.4934831145288,-12.76225334386));
#10331=CARTESIAN_POINT('Ctrl Pts',(81.3360655115292,-22.7464286725523,-12.7453864902349));
#10332=CARTESIAN_POINT('Ctrl Pts',(81.3366136549425,-22.9995968836278,-12.7285196366098));
#10333=CARTESIAN_POINT('Origin',(83.,-23.,-12.));
#10334=CARTESIAN_POINT('',(81.3341897502355,-23.0015225987737,-12.0285196366098));
#10335=CARTESIAN_POINT('',(81.3312395632066,-23.0000189542825,-12.2214803633902));
#10336=CARTESIAN_POINT('',(81.334,-23.,-12.));
#10337=CARTESIAN_POINT('Ctrl Pts',(81.3312396675144,-23.0000189535663,-12.2214803633902));
#10338=CARTESIAN_POINT('Ctrl Pts',(81.3313322263269,-22.4495888888226,-12.2584565903783));
#10339=CARTESIAN_POINT('Ctrl Pts',(81.6304402577157,-21.8990726361851,-12.2954328173664));
#10340=CARTESIAN_POINT('Ctrl Pts',(82.0923259468198,-21.5996822596601,-12.3324090443545));
#10341=CARTESIAN_POINT('Ctrl Pts',(82.5550628723794,-21.2997401189022,-12.3694534170184));
#10342=CARTESIAN_POINT('Ctrl Pts',(83.1811779936747,-21.2518503366662,-12.4064977896822));
#10343=CARTESIAN_POINT('Ctrl Pts',(83.6841487093753,-21.4779282197651,-12.4435421623461));
#10344=CARTESIAN_POINT('Ctrl Pts',(84.1871194250758,-21.704006102864,-12.4805865350099));
#10345=CARTESIAN_POINT('Ctrl Pts',(84.5669457351817,-22.2040516512977,-12.5176309076738));
#10346=CARTESIAN_POINT('Ctrl Pts',(84.6498116452796,-22.7492341813025,-12.5546752803377));
#10347=CARTESIAN_POINT('Ctrl Pts',(84.7326775553775,-23.2944167113074,-12.5917196530015));
#10348=CARTESIAN_POINT('Ctrl Pts',(84.5185830654674,-23.8847362228833,-12.6287640256654));
#10349=CARTESIAN_POINT('Ctrl Pts',(84.1055020274706,-24.2500508901584,-12.6658083983292));
#10350=CARTESIAN_POINT('Ctrl Pts',(83.6924209894737,-24.6153655574334,-12.7028527709931));
#10351=CARTESIAN_POINT('Ctrl Pts',(83.0803534033903,-24.7556753804077,-12.7398971436569));
#10352=CARTESIAN_POINT('Ctrl Pts',(82.5493934419846,-24.6067718228176,-12.7769415163208));
#10353=CARTESIAN_POINT('Ctrl Pts',(82.018433480579,-24.4578682652276,-12.8139858889846));
#10354=CARTESIAN_POINT('Ctrl Pts',(81.5685811438512,-24.0197513270734,-12.8510302616485));
#10355=CARTESIAN_POINT('Ctrl Pts',(81.4056977140957,-23.4929119413115,-12.8880746343123));
#10356=CARTESIAN_POINT('Ctrl Pts',(81.3567362539654,-23.3345482230394,-12.8992098773383));
#10357=CARTESIAN_POINT('Ctrl Pts',(81.3337040318532,-23.1681679377955,-12.9103451203643));
#10358=CARTESIAN_POINT('Ctrl Pts',(81.3350587862692,-23.0014219189523,-12.9214803633902));
#10359=CARTESIAN_POINT('Ctrl Pts',(81.3366136549425,-22.9995968836278,-12.7285196366098));
#10360=CARTESIAN_POINT('Ctrl Pts',(81.3372693892249,-23.3024575423211,-12.708342117571));
#10361=CARTESIAN_POINT('Ctrl Pts',(81.4162753651713,-23.6056368378878,-12.6881645985323));
#10362=CARTESIAN_POINT('Ctrl Pts',(81.571562362921,-23.8627441166811,-12.6679870794935));
#10363=CARTESIAN_POINT('Ctrl Pts',(81.8566573442934,-24.3347733008397,-12.6309427068297));
#10364=CARTESIAN_POINT('Ctrl Pts',(82.398866168514,-24.6515115227075,-12.5938983341658));
#10365=CARTESIAN_POINT('Ctrl Pts',(82.9500634070537,-24.6680131386102,-12.556853961502));
#10366=CARTESIAN_POINT('Ctrl Pts',(83.5012606455935,-24.684514754513,-12.5198095888381));
#10367=CARTESIAN_POINT('Ctrl Pts',(84.0614462984525,-24.4007797644507,-12.4827652161743));
#10368=CARTESIAN_POINT('Ctrl Pts',(84.3742683865361,-23.946650883726,-12.4457208435104));
#10369=CARTESIAN_POINT('Ctrl Pts',(84.6870904746197,-23.4925220030013,-12.4086764708466));
#10370=CARTESIAN_POINT('Ctrl Pts',(84.752548997928,-22.8679992316143,-12.3716320981827));
#10371=CARTESIAN_POINT('Ctrl Pts',(84.5406888479839,-22.35887648024,-12.3345877255189));
#10372=CARTESIAN_POINT('Ctrl Pts',(84.3288286980399,-21.8497537288657,-12.297543352855));
#10373=CARTESIAN_POINT('Ctrl Pts',(83.8396498748435,-21.4560309975041,-12.2604989801912));
#10374=CARTESIAN_POINT('Ctrl Pts',(83.2970102348348,-21.3578835564142,-12.2234546075273));
#10375=CARTESIAN_POINT('Ctrl Pts',(82.7543705948261,-21.2597361153243,-12.1864102348635));
#10376=CARTESIAN_POINT('Ctrl Pts',(82.1582701380051,-21.457163964506,-12.1493658621996));
#10377=CARTESIAN_POINT('Ctrl Pts',(81.7814961645559,-21.8598202348316,-12.1123214895357));
#10378=CARTESIAN_POINT('Ctrl Pts',(81.4973832225279,-22.163450171212,-12.0843875385604));
#10379=CARTESIAN_POINT('Ctrl Pts',(81.3379831636485,-22.5837765854249,-12.0564535875851));
#10380=CARTESIAN_POINT('Ctrl Pts',(81.3341897502355,-23.0015225987737,-12.0285196366098));
#10381=CARTESIAN_POINT('Origin',(83.,-23.,-12.));
#10382=CARTESIAN_POINT('',(81.3314457178217,-22.9994693778887,-11.3285196366098));
#10383=CARTESIAN_POINT('',(81.3350035286226,-22.9985661148555,-11.5214803633902));
#10384=CARTESIAN_POINT('',(81.334,-23.,-12.));
#10385=CARTESIAN_POINT('Ctrl Pts',(81.3350035286226,-22.9985661148555,-11.5214803633902));
#10386=CARTESIAN_POINT('Ctrl Pts',(81.3336508207863,-22.8338748378415,-11.5324793150647));
#10387=CARTESIAN_POINT('Ctrl Pts',(81.3561116693081,-22.6695443672682,-11.5434782667392));
#10388=CARTESIAN_POINT('Ctrl Pts',(81.4038994461849,-22.5129425261447,-11.5544772184136));
#10389=CARTESIAN_POINT('Ctrl Pts',(81.5648482591078,-21.9855089002755,-11.5915215910775));
#10390=CARTESIAN_POINT('Ctrl Pts',(82.0130896610182,-21.5457439380849,-11.6285659637413));
#10391=CARTESIAN_POINT('Ctrl Pts',(82.543499565097,-21.3948927407614,-11.6656103364052));
#10392=CARTESIAN_POINT('Ctrl Pts',(83.0739094691758,-21.2440415434378,-11.702654709069));
#10393=CARTESIAN_POINT('Ctrl Pts',(83.6864878754231,-21.3821041109814,-11.7396990817329));
#10394=CARTESIAN_POINT('Ctrl Pts',(84.1009068497144,-21.7459002954393,-11.7767434543967));
#10395=CARTESIAN_POINT('Ctrl Pts',(84.5153258240058,-22.1096964798972,-11.8137878270606));
#10396=CARTESIAN_POINT('Ctrl Pts',(84.7315853663412,-22.6992262812694,-11.8508321997244));
#10397=CARTESIAN_POINT('Ctrl Pts',(84.6507208542018,-23.2447092606146,-11.8878765723883));
#10398=CARTESIAN_POINT('Ctrl Pts',(84.5698563420624,-23.7901922399597,-11.9249209450521));
#10399=CARTESIAN_POINT('Ctrl Pts',(84.191867775448,-24.2916283972779,-11.961965317716));
#10400=CARTESIAN_POINT('Ctrl Pts',(83.689730161184,-24.5195506788128,-11.9990096903799));
#10401=CARTESIAN_POINT('Ctrl Pts',(83.18759254692,-24.7474729603476,-12.0360540630437));
#10402=CARTESIAN_POINT('Ctrl Pts',(82.5613058850063,-24.7018813660993,-12.0730984357076));
#10403=CARTESIAN_POINT('Ctrl Pts',(82.0974712771361,-24.4036395068296,-12.1101428083714));
#10404=CARTESIAN_POINT('Ctrl Pts',(81.632783413548,-24.1048490111119,-12.147255326711));
#10405=CARTESIAN_POINT('Ctrl Pts',(81.3311467675376,-23.5524778585552,-12.1843678450506));
#10406=CARTESIAN_POINT('Ctrl Pts',(81.3312396675144,-23.0000189535663,-12.2214803633902));
#10407=CARTESIAN_POINT('Ctrl Pts',(81.3341897502355,-23.0015225987737,-12.0285196366098));
#10408=CARTESIAN_POINT('Ctrl Pts',(81.3329525605568,-23.1377669253881,-12.0194092149213));
#10409=CARTESIAN_POINT('Ctrl Pts',(81.3482669854987,-23.2737367791447,-12.0102987932327));
#10410=CARTESIAN_POINT('Ctrl Pts',(81.3812047643192,-23.4052943113693,-12.0011883715442));
#10411=CARTESIAN_POINT('Ctrl Pts',(81.5151348276092,-23.9402274261121,-11.9641439988803));
#10412=CARTESIAN_POINT('Ctrl Pts',(81.9404424442667,-24.4022089641281,-11.9270996262165));
#10413=CARTESIAN_POINT('Ctrl Pts',(82.462498478937,-24.5798270819132,-11.8900552535526));
#10414=CARTESIAN_POINT('Ctrl Pts',(82.9845545136073,-24.7574451996984,-11.8530108808888));
#10415=CARTESIAN_POINT('Ctrl Pts',(83.6033589662905,-24.6506998972526,-11.8159665082249));
#10416=CARTESIAN_POINT('Ctrl Pts',(84.0357347414856,-24.3084399257021,-11.7789221355611));
#10417=CARTESIAN_POINT('Ctrl Pts',(84.4681105166806,-23.9661799541517,-11.7418777628972));
#10418=CARTESIAN_POINT('Ctrl Pts',(84.7140576143876,-23.3884053134966,-11.7048333902334));
#10419=CARTESIAN_POINT('Ctrl Pts',(84.6610258025042,-22.8395170497948,-11.6677890175695));
#10420=CARTESIAN_POINT('Ctrl Pts',(84.6079939906208,-22.290628786093,-11.6307446449057));
#10421=CARTESIAN_POINT('Ctrl Pts',(84.255983269147,-21.7706268993444,-11.5937002722418));
#10422=CARTESIAN_POINT('Ctrl Pts',(83.7660806717326,-21.5174744864626,-11.556655899578));
#10423=CARTESIAN_POINT('Ctrl Pts',(83.2761780743183,-21.2643220735809,-11.5196115269141));
#10424=CARTESIAN_POINT('Ctrl Pts',(82.6483836009633,-21.2780191345659,-11.4825671542502));
#10425=CARTESIAN_POINT('Ctrl Pts',(82.1699883575499,-21.5522976247554,-11.4455227815864));
#10426=CARTESIAN_POINT('Ctrl Pts',(81.6915931141365,-21.826576114945,-11.4084784089225));
#10427=CARTESIAN_POINT('Ctrl Pts',(81.3625971006646,-22.3614360343391,-11.3714340362587));
#10428=CARTESIAN_POINT('Ctrl Pts',(81.3335553674774,-22.9121149578823,-11.3343896635948));
#10429=CARTESIAN_POINT('Ctrl Pts',(81.3320213894825,-22.9412016981782,-11.3324329879332));
#10430=CARTESIAN_POINT('Ctrl Pts',(81.3313242627211,-22.9703325723772,-11.3304763122715));
#10431=CARTESIAN_POINT('Ctrl Pts',(81.3314457178217,-22.9994693778887,-11.3285196366098));
#10432=CARTESIAN_POINT('Origin',(83.,-23.,-12.));
#10433=CARTESIAN_POINT('',(81.3357538816894,-22.9988133680852,-10.6285196366098));
#10434=CARTESIAN_POINT('',(81.3362972869656,-23.0008273571659,-10.8214803633902));
#10435=CARTESIAN_POINT('',(81.334,-23.,-12.));
#10436=CARTESIAN_POINT('Ctrl Pts',(81.3362972869656,-23.0008273571659,-10.8214803633902));
#10437=CARTESIAN_POINT('Ctrl Pts',(81.3377852983276,-22.6697775144948,-10.8435464124149));
#10438=CARTESIAN_POINT('Ctrl Pts',(81.4333699328181,-22.3379359375284,-10.8656124614396));
#10439=CARTESIAN_POINT('Ctrl Pts',(81.6172641946395,-22.0657603876407,-10.8876785104643));
#10440=CARTESIAN_POINT('Ctrl Pts',(81.9259849610095,-21.6088334367057,-10.9247228831281));
#10441=CARTESIAN_POINT('Ctrl Pts',(82.4835933983085,-21.3200663904382,-10.961767255792));
#10442=CARTESIAN_POINT('Ctrl Pts',(83.0349169120014,-21.3316047320903,-10.9988116284558));
#10443=CARTESIAN_POINT('Ctrl Pts',(83.5862404256943,-21.3431430737424,-11.0358560011197));
#10444=CARTESIAN_POINT('Ctrl Pts',(84.1312790157812,-21.6549868033142,-11.0729003737835));
#10445=CARTESIAN_POINT('Ctrl Pts',(84.4206122971833,-22.1244300931287,-11.1099447464474));
#10446=CARTESIAN_POINT('Ctrl Pts',(84.7099455785855,-22.5938733829432,-11.1469891191112));
#10447=CARTESIAN_POINT('Ctrl Pts',(84.7435735513029,-23.2209162330006,-11.1840334917751));
#10448=CARTESIAN_POINT('Ctrl Pts',(84.506107393228,-23.7186114950314,-11.2210778644389));
#10449=CARTESIAN_POINT('Ctrl Pts',(84.2686412351531,-24.2163067570623,-11.2581222371028));
#10450=CARTESIAN_POINT('Ctrl Pts',(83.7600809462859,-24.5846544310667,-11.2951666097666));
#10451=CARTESIAN_POINT('Ctrl Pts',(83.213153723181,-24.6550913724086,-11.3322109824305));
#10452=CARTESIAN_POINT('Ctrl Pts',(82.6662265000761,-24.7255283137505,-11.3692553550943));
#10453=CARTESIAN_POINT('Ctrl Pts',(82.0809323427335,-24.4980545224299,-11.4062997277582));
#10454=CARTESIAN_POINT('Ctrl Pts',(81.72511337603,-24.0767664819958,-11.4433441004221));
#10455=CARTESIAN_POINT('Ctrl Pts',(81.4749416463615,-23.7805642903574,-11.4693895214114));
#10456=CARTESIAN_POINT('Ctrl Pts',(81.3382067289016,-23.3885536127611,-11.4954349424008));
#10457=CARTESIAN_POINT('Ctrl Pts',(81.3350035286226,-22.9985661148555,-11.5214803633902));
#10458=CARTESIAN_POINT('Ctrl Pts',(81.3314457178217,-22.9994693778887,-11.3285196366098));
#10459=CARTESIAN_POINT('Ctrl Pts',(81.3336236872483,-23.5219593456538,-11.2934319396076));
#10460=CARTESIAN_POINT('Ctrl Pts',(81.5990309145572,-24.0463566302869,-11.2583442426054));
#10461=CARTESIAN_POINT('Ctrl Pts',(82.0223180957112,-24.3523681406768,-11.2232565456033));
#10462=CARTESIAN_POINT('Ctrl Pts',(82.4692100100346,-24.6754444722357,-11.1862121729394));
#10463=CARTESIAN_POINT('Ctrl Pts',(83.092081291584,-24.7550992076612,-11.1491678002756));
#10464=CARTESIAN_POINT('Ctrl Pts',(83.6058937839349,-24.5548807724326,-11.1121234276117));
#10465=CARTESIAN_POINT('Ctrl Pts',(84.1197062762858,-24.354662337204,-11.0750790549479));
#10466=CARTESIAN_POINT('Ctrl Pts',(84.5244599794382,-23.8745707313213,-11.038034682284));
#10467=CARTESIAN_POINT('Ctrl Pts',(84.6349316333544,-23.3343053217472,-11.0009903096202));
#10468=CARTESIAN_POINT('Ctrl Pts',(84.7454032872706,-22.7940399121731,-10.9639459369563));
#10469=CARTESIAN_POINT('Ctrl Pts',(84.5615928919505,-22.1936006989076,-10.9269015642925));
#10470=CARTESIAN_POINT('Ctrl Pts',(84.167615701646,-21.8077604824695,-10.8898571916286));
#10471=CARTESIAN_POINT('Ctrl Pts',(83.7736385113415,-21.4219202660315,-10.8528128189647));
#10472=CARTESIAN_POINT('Ctrl Pts',(83.1694945260525,-21.2506790464209,-10.8157684463009));
#10473=CARTESIAN_POINT('Ctrl Pts',(82.631651922885,-21.3724001757259,-10.778724073637));
#10474=CARTESIAN_POINT('Ctrl Pts',(82.0938093197176,-21.4941213050309,-10.7416797009732));
#10475=CARTESIAN_POINT('Ctrl Pts',(81.6222680986716,-21.9088047832515,-10.7046353283093));
#10476=CARTESIAN_POINT('Ctrl Pts',(81.4328148023386,-22.4266832898627,-10.6675909556455));
#10477=CARTESIAN_POINT('Ctrl Pts',(81.3662082829035,-22.6087549955722,-10.6545671826336));
#10478=CARTESIAN_POINT('Ctrl Pts',(81.3344686881453,-22.80358192037,-10.6415434096217));
#10479=CARTESIAN_POINT('Ctrl Pts',(81.3357538816894,-22.9988133680852,-10.6285196366098));
#10480=CARTESIAN_POINT('Origin',(83.,-23.,-12.));
#10481=CARTESIAN_POINT('',(81.3357307175978,-23.0011975492408,-9.92851963660979));
#10482=CARTESIAN_POINT('',(81.3319839174274,-23.0009873429913,-10.1214803633902));
#10483=CARTESIAN_POINT('',(81.334,-23.,-12.));
#10484=CARTESIAN_POINT('Ctrl Pts',(81.3319839174274,-23.0009873429913,-10.1214803633902));
#10485=CARTESIAN_POINT('Ctrl Pts',(81.3354512767123,-22.5071811287366,-10.1546135097651));
#10486=CARTESIAN_POINT('Ctrl Pts',(81.5685740227169,-22.0105308872886,-10.18774665614));
#10487=CARTESIAN_POINT('Ctrl Pts',(81.9525268434233,-21.700938051139,-10.2208798025149));
#10488=CARTESIAN_POINT('Ctrl Pts',(82.3818036532575,-21.3547991041577,-10.2579241751788));
#10489=CARTESIAN_POINT('Ctrl Pts',(82.9996220147682,-21.242486822828,-10.2949685478426));
#10490=CARTESIAN_POINT('Ctrl Pts',(83.523256087181,-21.4153975173706,-10.3320129205065));
#10491=CARTESIAN_POINT('Ctrl Pts',(84.0468901595938,-21.5883082119132,-10.3690572931703));
#10492=CARTESIAN_POINT('Ctrl Pts',(84.4763399429088,-22.0464418823281,-10.4061016658342));
#10493=CARTESIAN_POINT('Ctrl Pts',(84.6150807647917,-22.5801475450506,-10.443146038498));
#10494=CARTESIAN_POINT('Ctrl Pts',(84.7538215866746,-23.1138532077731,-10.4801904111619));
#10495=CARTESIAN_POINT('Ctrl Pts',(84.6018534471254,-23.7231308628033,-10.5172347838257));
#10496=CARTESIAN_POINT('Ctrl Pts',(84.2287199575057,-24.1291630647319,-10.5542791564896));
#10497=CARTESIAN_POINT('Ctrl Pts',(83.8555864678859,-24.5351952666605,-10.5913235291534));
#10498=CARTESIAN_POINT('Ctrl Pts',(83.2612876281956,-24.7379820154875,-10.6283679018173));
#10499=CARTESIAN_POINT('Ctrl Pts',(82.7177862831642,-24.6447241041454,-10.6654122744811));
#10500=CARTESIAN_POINT('Ctrl Pts',(82.1742849381328,-24.5514661928033,-10.702456647145));
#10501=CARTESIAN_POINT('Ctrl Pts',(81.6815810877603,-24.1621636212921,-10.7395010198088));
#10502=CARTESIAN_POINT('Ctrl Pts',(81.4651457102945,-23.6549689077352,-10.7765453924727));
#10503=CARTESIAN_POINT('Ctrl Pts',(81.3776333866262,-23.4498925082327,-10.7915237161119));
#10504=CARTESIAN_POINT('Ctrl Pts',(81.3352872323004,-23.2255423334935,-10.806502039751));
#10505=CARTESIAN_POINT('Ctrl Pts',(81.3362972869656,-23.0008273571659,-10.8214803633902));
#10506=CARTESIAN_POINT('Ctrl Pts',(81.3357538816894,-22.9988133680852,-10.6285196366098));
#10507=CARTESIAN_POINT('Ctrl Pts',(81.3381242485233,-23.3588915451814,-10.6044990369578));
#10508=CARTESIAN_POINT('Ctrl Pts',(81.4528345315299,-23.720345781685,-10.5804784373059));
#10509=CARTESIAN_POINT('Ctrl Pts',(81.6683272585003,-24.005688422643,-10.5564578376539));
#10510=CARTESIAN_POINT('Ctrl Pts',(82.0006583826149,-24.4457415138104,-10.5194134649901));
#10511=CARTESIAN_POINT('Ctrl Pts',(82.5726860024639,-24.7047741611435,-10.4823690923262));
#10512=CARTESIAN_POINT('Ctrl Pts',(83.1226390218108,-24.6642479275098,-10.4453247196624));
#10513=CARTESIAN_POINT('Ctrl Pts',(83.6725920411577,-24.6237216938762,-10.4082803469985));
#10514=CARTESIAN_POINT('Ctrl Pts',(84.2004704600023,-24.2836365792757,-10.3712359743347));
#10515=CARTESIAN_POINT('Ctrl Pts',(84.4647067253352,-23.7996222249595,-10.3341916016708));
#10516=CARTESIAN_POINT('Ctrl Pts',(84.7289429906682,-23.3156078706434,-10.297147229007));
#10517=CARTESIAN_POINT('Ctrl Pts',(84.7295371024896,-22.6876642766114,-10.2601028563431));
#10518=CARTESIAN_POINT('Ctrl Pts',(84.4662171835379,-22.2031507893022,-10.2230584836792));
#10519=CARTESIAN_POINT('Ctrl Pts',(84.2028972645862,-21.718637301993,-10.1860141110154));
#10520=CARTESIAN_POINT('Ctrl Pts',(83.6756633148615,-21.3775539214065,-10.1489697383515));
#10521=CARTESIAN_POINT('Ctrl Pts',(83.1257879656207,-21.3359871149548,-10.1119253656877));
#10522=CARTESIAN_POINT('Ctrl Pts',(82.57591261638,-21.294420308503,-10.0748809930238));
#10523=CARTESIAN_POINT('Ctrl Pts',(82.0033958676232,-21.5523700761859,-10.03783662036));
#10524=CARTESIAN_POINT('Ctrl Pts',(81.6702326506014,-21.9917935279097,-10.0007922476961));
#10525=CARTESIAN_POINT('Ctrl Pts',(81.4535683830342,-22.2775614502231,-9.97670137733401));
#10526=CARTESIAN_POINT('Ctrl Pts',(81.3381320398903,-22.6400786239042,-9.9526105069719));
#10527=CARTESIAN_POINT('Ctrl Pts',(81.3357307175978,-23.0011975492408,-9.92851963660979));
#10528=CARTESIAN_POINT('Origin',(83.,-23.,-12.));
#10529=CARTESIAN_POINT('',(81.331431843514,-23.0005124578661,-9.22851963660979));
#10530=CARTESIAN_POINT('',(81.3333049370251,-22.9985455594153,-9.42148036339021));
#10531=CARTESIAN_POINT('',(81.334,-23.,-12.));
#10532=CARTESIAN_POINT('Ctrl Pts',(81.3333049370251,-22.9985455594153,-9.42148036339021));
#10533=CARTESIAN_POINT('Ctrl Pts',(81.3323267498425,-22.8916766658214,-9.42863623445147));
#10534=CARTESIAN_POINT('Ctrl Pts',(81.3417252765875,-22.7849791349272,-9.43579210551273));
#10535=CARTESIAN_POINT('Ctrl Pts',(81.3621246357665,-22.6804280175552,-9.44294797657399));
#10536=CARTESIAN_POINT('Ctrl Pts',(81.4677276374222,-22.1391898480586,-9.47999234923785));
#10537=CARTESIAN_POINT('Ctrl Pts',(81.8681425497088,-21.655473532047,-9.5170367219017));
#10538=CARTESIAN_POINT('Ctrl Pts',(82.3801316286753,-21.4506371751721,-9.55408109456555));
#10539=CARTESIAN_POINT('Ctrl Pts',(82.8921207076418,-21.2458008182972,-9.59112546722941));
#10540=CARTESIAN_POINT('Ctrl Pts',(83.5156839532884,-21.3198444205589,-9.62816983989325));
#10541=CARTESIAN_POINT('Ctrl Pts',(83.965466552802,-21.6388841723983,-9.66521421255711));
#10542=CARTESIAN_POINT('Ctrl Pts',(84.4152491523155,-21.9579239242376,-9.70225858522096));
#10543=CARTESIAN_POINT('Ctrl Pts',(84.6912511056959,-22.5219598256545,-9.73930295788482));
#10544=CARTESIAN_POINT('Ctrl Pts',(84.667168487411,-23.0728779480423,-9.77634733054867));
#10545=CARTESIAN_POINT('Ctrl Pts',(84.6430858691261,-23.6237960704302,-9.81339170321253));
#10546=CARTESIAN_POINT('Ctrl Pts',(84.3189186791757,-24.161596413789,-9.85043607587638));
#10547=CARTESIAN_POINT('Ctrl Pts',(83.8430122032293,-24.44017095719,-9.88748044854023));
#10548=CARTESIAN_POINT('Ctrl Pts',(83.3671057272829,-24.7187455005911,-9.92452482120408));
#10549=CARTESIAN_POINT('Ctrl Pts',(82.7394599653405,-24.7380942440345,-9.96156919386794));
#10550=CARTESIAN_POINT('Ctrl Pts',(82.2472979700152,-24.4893628217409,-9.99861356653179));
#10551=CARTESIAN_POINT('Ctrl Pts',(81.7551359746898,-24.2406313994473,-10.0356579391956));
#10552=CARTESIAN_POINT('Ctrl Pts',(81.3984577459816,-23.7238198114168,-10.0727023118595));
#10553=CARTESIAN_POINT('Ctrl Pts',(81.3404862607064,-23.175431211085,-10.1097466845233));
#10554=CARTESIAN_POINT('Ctrl Pts',(81.3343655038704,-23.1175311373102,-10.1136579108123));
#10555=CARTESIAN_POINT('Ctrl Pts',(81.3315746104864,-23.0592790556162,-10.1175691371013));
#10556=CARTESIAN_POINT('Ctrl Pts',(81.3319839174274,-23.0009873429913,-10.1214803633902));
#10557=CARTESIAN_POINT('Ctrl Pts',(81.3357307175978,-23.0011975492408,-9.92851963660979));
#10558=CARTESIAN_POINT('Ctrl Pts',(81.3344395424192,-23.1953688166229,-9.91556613430805));
#10559=CARTESIAN_POINT('Ctrl Pts',(81.3658283975604,-23.3891358305449,-9.90261263200631));
#10560=CARTESIAN_POINT('Ctrl Pts',(81.4317327528845,-23.5703501867417,-9.88965912970457));
#10561=CARTESIAN_POINT('Ctrl Pts',(81.6202057574764,-24.088586258085,-9.85261475704071));
#10562=CARTESIAN_POINT('Ctrl Pts',(82.0909614519471,-24.5041612650069,-9.81557038437686));
#10563=CARTESIAN_POINT('Ctrl Pts',(82.6285727661251,-24.6268999059032,-9.77852601171301));
#10564=CARTESIAN_POINT('Ctrl Pts',(83.1661840803031,-24.7496385467995,-9.74148163904916));
#10565=CARTESIAN_POINT('Ctrl Pts',(83.7706510141882,-24.5795408216701,-9.7044372663853));
#10566=CARTESIAN_POINT('Ctrl Pts',(84.1653576030415,-24.1944467970255,-9.66739289372145));
#10567=CARTESIAN_POINT('Ctrl Pts',(84.5600641918947,-23.8093527723809,-9.63034852105759));
#10568=CARTESIAN_POINT('Ctrl Pts',(84.745010435716,-23.2092624482211,-9.59330414839375));
#10569=CARTESIAN_POINT('Ctrl Pts',(84.635561293626,-22.6687889665429,-9.55625977572989));
#10570=CARTESIAN_POINT('Ctrl Pts',(84.5261121515361,-22.1283154848647,-9.51921540306604));
#10571=CARTESIAN_POINT('Ctrl Pts',(84.1222676235349,-21.6474588456682,-9.48217103040219));
#10572=CARTESIAN_POINT('Ctrl Pts',(83.6088349132188,-21.4462685102183,-9.44512665773833));
#10573=CARTESIAN_POINT('Ctrl Pts',(83.0954022029027,-21.2450781747684,-9.40808228507448));
#10574=CARTESIAN_POINT('Ctrl Pts',(82.4723813102717,-21.3235541430652,-9.37103791241062));
#10575=CARTESIAN_POINT('Ctrl Pts',(82.0248788567251,-21.6457842676196,-9.33399353974677));
#10576=CARTESIAN_POINT('Ctrl Pts',(81.600164502517,-21.9516055165803,-9.29883557203444));
#10577=CARTESIAN_POINT('Ctrl Pts',(81.3335479331276,-22.4769876979749,-9.26367760432212));
#10578=CARTESIAN_POINT('Ctrl Pts',(81.331431843514,-23.0005124578661,-9.22851963660979));
#10579=CARTESIAN_POINT('Origin',(83.,-23.,-12.));
#10580=CARTESIAN_POINT('',(81.3342212297538,-22.9984780339595,-8.52851963660979));
#10581=CARTESIAN_POINT('',(81.3367006367545,-22.9999263102539,-8.72148036339021));
#10582=CARTESIAN_POINT('',(81.334,-23.,-12.));
#10583=CARTESIAN_POINT('Ctrl Pts',(81.3367006367545,-22.9999263102539,-8.72148036339021));
#10584=CARTESIAN_POINT('Ctrl Pts',(81.3365926969101,-22.7263673067472,-8.73970333180169));
#10585=CARTESIAN_POINT('Ctrl Pts',(81.4003183665741,-22.4528556568932,-8.75792630021316));
#10586=CARTESIAN_POINT('Ctrl Pts',(81.5281532603125,-22.2135973451411,-8.77614926862464));
#10587=CARTESIAN_POINT('Ctrl Pts',(81.7880211005105,-21.7272235632556,-8.81319364128849));
#10588=CARTESIAN_POINT('Ctrl Pts',(82.3128162721351,-21.3823995440889,-8.85023801395235));
#10589=CARTESIAN_POINT('Ctrl Pts',(82.8623821768039,-21.3369235449087,-8.8872823866162));
#10590=CARTESIAN_POINT('Ctrl Pts',(83.4119480814727,-21.2914475457284,-8.92432675928005));
#10591=CARTESIAN_POINT('Ctrl Pts',(83.9862847191857,-21.5453195665347,-8.9613711319439));
#10592=CARTESIAN_POINT('Ctrl Pts',(84.3225643416799,-21.9823627744406,-8.99841550460776));
#10593=CARTESIAN_POINT('Ctrl Pts',(84.658843964174,-22.4194059823464,-9.03545987727161));
#10594=CARTESIAN_POINT('Ctrl Pts',(84.7570665714493,-23.0396203773518,-9.07250424993546));
#10595=CARTESIAN_POINT('Ctrl Pts',(84.5722835654198,-23.5591836466087,-9.10954862259931));
#10596=CARTESIAN_POINT('Ctrl Pts',(84.3875005593903,-24.0787469158655,-9.14659299526317));
#10597=CARTESIAN_POINT('Ctrl Pts',(83.9197119400561,-24.4976590593737,-9.18363736792702));
#10598=CARTESIAN_POINT('Ctrl Pts',(83.3829869856121,-24.62421763615,-9.22068174059087));
#10599=CARTESIAN_POINT('Ctrl Pts',(82.8462620311681,-24.7507762129263,-9.25772611325472));
#10600=CARTESIAN_POINT('Ctrl Pts',(82.2406007416144,-24.5849812229706,-9.29477048591858));
#10601=CARTESIAN_POINT('Ctrl Pts',(81.84316564235,-24.202703716502,-9.33181485858243));
#10602=CARTESIAN_POINT('Ctrl Pts',(81.5225031841386,-23.8942708549605,-9.36170336018503));
#10603=CARTESIAN_POINT('Ctrl Pts',(81.3373906100235,-23.4449134537085,-9.39159186178762));
#10604=CARTESIAN_POINT('Ctrl Pts',(81.3333049370251,-22.9985455594153,-9.42148036339021));
#10605=CARTESIAN_POINT('Ctrl Pts',(81.331431843514,-23.0005124578661,-9.22851963660979));
#10606=CARTESIAN_POINT('Ctrl Pts',(81.3313183044734,-23.0286022413082,-9.22663323165827));
#10607=CARTESIAN_POINT('Ctrl Pts',(81.3319662284119,-23.056686677472,-9.22474682670674));
#10608=CARTESIAN_POINT('Ctrl Pts',(81.3333920509507,-23.084731564703,-9.22286042175522));
#10609=CARTESIAN_POINT('Ctrl Pts',(81.3613917131847,-23.6354644564197,-9.18581604909136));
#10610=CARTESIAN_POINT('Ctrl Pts',(81.6893750521149,-24.170945959041,-9.1487716764275));
#10611=CARTESIAN_POINT('Ctrl Pts',(82.1672504371963,-24.4461291987769,-9.11172730376365));
#10612=CARTESIAN_POINT('Ctrl Pts',(82.6451258222777,-24.7213124385128,-9.0746829310998));
#10613=CARTESIAN_POINT('Ctrl Pts',(83.2728932535105,-24.7361974153634,-9.03763855843595));
#10614=CARTESIAN_POINT('Ctrl Pts',(83.7632740000222,-24.4839724710224,-9.0005941857721));
#10615=CARTESIAN_POINT('Ctrl Pts',(84.2536547465338,-24.2317475266814,-8.96354981310824));
#10616=CARTESIAN_POINT('Ctrl Pts',(84.6066488083243,-23.7124126611489,-8.92650544044439));
#10617=CARTESIAN_POINT('Ctrl Pts',(84.6607191558582,-23.1636257292351,-8.88946106778053));
#10618=CARTESIAN_POINT('Ctrl Pts',(84.7147895033921,-22.6148387973213,-8.85241669511668));
#10619=CARTESIAN_POINT('Ctrl Pts',(84.4699361366694,-22.0365997990262,-8.81537232245283));
#10620=CARTESIAN_POINT('Ctrl Pts',(84.0382087749791,-21.6935222797378,-8.77832794978898));
#10621=CARTESIAN_POINT('Ctrl Pts',(83.6064814132889,-21.3504447604494,-8.74128357712513));
#10622=CARTESIAN_POINT('Ctrl Pts',(82.9878800566311,-21.2425287201677,-8.70423920446127));
#10623=CARTESIAN_POINT('Ctrl Pts',(82.4654888597494,-21.4191586624222,-8.66719483179742));
#10624=CARTESIAN_POINT('Ctrl Pts',(81.9430976628678,-21.5957886046768,-8.63015045913356));
#10625=CARTESIAN_POINT('Ctrl Pts',(81.5169166257624,-22.0569645294676,-8.59310608646971));
#10626=CARTESIAN_POINT('Ctrl Pts',(81.3819745782115,-22.5916432582957,-8.55606171380586));
#10627=CARTESIAN_POINT('Ctrl Pts',(81.3485319433084,-22.7241524786849,-8.54688102140717));
#10628=CARTESIAN_POINT('Ctrl Pts',(81.3329770659435,-22.861176205662,-8.53770032900848));
#10629=CARTESIAN_POINT('Ctrl Pts',(81.3342212297538,-22.9984780339595,-8.52851963660979));
#10630=CARTESIAN_POINT('Origin',(83.,-23.,-12.));
#10631=CARTESIAN_POINT('',(81.3366058837444,-23.0004198226253,-7.82851963660979));
#10632=CARTESIAN_POINT('',(81.3335753931735,-23.0014929636922,-8.02148036339021));
#10633=CARTESIAN_POINT('',(81.334,-23.,-12.));
#10634=CARTESIAN_POINT('Ctrl Pts',(81.3335753931735,-23.0014929636922,-8.02148036339021));
#10635=CARTESIAN_POINT('Ctrl Pts',(81.337614240534,-22.5638796924227,-8.05077042915191));
#10636=CARTESIAN_POINT('Ctrl Pts',(81.5146048346072,-22.123375374204,-8.0800604949136));
#10637=CARTESIAN_POINT('Ctrl Pts',(81.8239355420513,-21.8160936061122,-8.10935056067529));
#10638=CARTESIAN_POINT('Ctrl Pts',(82.2151590406997,-21.4274614868599,-8.14639493333914));
#10639=CARTESIAN_POINT('Ctrl Pts',(82.8180700802442,-21.2519284296373,-8.18343930600298));
#10640=CARTESIAN_POINT('Ctrl Pts',(83.356764705155,-21.3698218175571,-8.22048367866684));
#10641=CARTESIAN_POINT('Ctrl Pts',(83.8954593300658,-21.4877152054768,-8.25752805133069));
#10642=CARTESIAN_POINT('Ctrl Pts',(84.369937540343,-21.8990350385389,-8.29457242399455));
#10643=CARTESIAN_POINT('Ctrl Pts',(84.5630687686518,-22.415553265601,-8.33161679665841));
#10644=CARTESIAN_POINT('Ctrl Pts',(84.7561999969607,-22.9320714926631,-8.36866116932226));
#10645=CARTESIAN_POINT('Ctrl Pts',(84.6679842433012,-23.5537881137252,-8.40570554198611));
#10646=CARTESIAN_POINT('Ctrl Pts',(84.3387907729539,-23.9961933681454,-8.44274991464996));
#10647=CARTESIAN_POINT('Ctrl Pts',(84.0095973026066,-24.4385986225656,-8.47979428731381));
#10648=CARTESIAN_POINT('Ctrl Pts',(83.4394261155714,-24.701692510344,-8.51683865997767));
#10649=CARTESIAN_POINT('Ctrl Pts',(82.8891987677264,-24.6650780905852,-8.55388303264152));
#10650=CARTESIAN_POINT('Ctrl Pts',(82.3389714198814,-24.6284636708265,-8.59092740530537));
#10651=CARTESIAN_POINT('Ctrl Pts',(81.8086879112266,-24.2921409435307,-8.62797177796922));
#10652=CARTESIAN_POINT('Ctrl Pts',(81.5410164112849,-23.8100178075807,-8.66501615063307));
#10653=CARTESIAN_POINT('Ctrl Pts',(81.4050186025769,-23.5650619940897,-8.68383755488545));
#10654=CARTESIAN_POINT('Ctrl Pts',(81.3368121213051,-23.2824688947341,-8.70265895913783));
#10655=CARTESIAN_POINT('Ctrl Pts',(81.3367006367545,-22.9999263102539,-8.72148036339021));
#10656=CARTESIAN_POINT('Ctrl Pts',(81.3342212297538,-22.9984780339595,-8.52851963660979));
#10657=CARTESIAN_POINT('Ctrl Pts',(81.3379973047056,-23.4151932529611,-8.50065595634463));
#10658=CARTESIAN_POINT('Ctrl Pts',(81.4965162247509,-23.8344701770685,-8.47279227607947));
#10659=CARTESIAN_POINT('Ctrl Pts',(81.7793408475925,-24.1378720174819,-8.4449285958143));
#10660=CARTESIAN_POINT('Ctrl Pts',(82.1553522225205,-24.5412405149744,-8.40788422315045));
#10661=CARTESIAN_POINT('Ctrl Pts',(82.7510780303727,-24.7397959770939,-8.37083985048659));
#10662=CARTESIAN_POINT('Ctrl Pts',(83.293902417857,-24.6426755189852,-8.33379547782274));
#10663=CARTESIAN_POINT('Ctrl Pts',(83.8367268053414,-24.5455550608765,-8.29675110515889));
#10664=CARTESIAN_POINT('Ctrl Pts',(84.326649772458,-24.1527586825395,-8.25970673249504));
#10665=CARTESIAN_POINT('Ctrl Pts',(84.5394729275635,-23.6440377325831,-8.22266235983118));
#10666=CARTESIAN_POINT('Ctrl Pts',(84.7522960826691,-23.1353167826267,-8.18561798716733));
#10667=CARTESIAN_POINT('Ctrl Pts',(84.6880194257635,-22.5106712610509,-8.14857361450348));
#10668=CARTESIAN_POINT('Ctrl Pts',(84.3760572205986,-22.055951259959,-8.11152924183962));
#10669=CARTESIAN_POINT('Ctrl Pts',(84.0640950154338,-21.601231258867,-8.07448486917577));
#10670=CARTESIAN_POINT('Ctrl Pts',(83.5044472620097,-21.3164367782588,-8.03744049651192));
#10671=CARTESIAN_POINT('Ctrl Pts',(82.9532197848582,-21.3318953601593,-8.00039612384806));
#10672=CARTESIAN_POINT('Ctrl Pts',(82.4019923077066,-21.3473539420599,-7.96335175118421));
#10673=CARTESIAN_POINT('Ctrl Pts',(81.8591851068275,-21.6630655864691,-7.92630737852036));
#10674=CARTESIAN_POINT('Ctrl Pts',(81.5731974420689,-22.1345544656655,-7.8892630058565));
#10675=CARTESIAN_POINT('Ctrl Pts',(81.416881713379,-22.3922618314115,-7.8690152161076));
#10676=CARTESIAN_POINT('Ctrl Pts',(81.3372913231897,-22.6965079505961,-7.84876742635869));
#10677=CARTESIAN_POINT('Ctrl Pts',(81.3366058837444,-23.0004198226253,-7.82851963660979));
#10678=CARTESIAN_POINT('Origin',(83.,-23.,-12.));
#10679=CARTESIAN_POINT('',(81.3326823670782,-23.0013023207031,-7.12851963660979));
#10680=CARTESIAN_POINT('',(81.3317907907837,-22.9991411291167,-7.32148036339021));
#10681=CARTESIAN_POINT('',(81.334,-23.,-12.));
#10682=CARTESIAN_POINT('Ctrl Pts',(81.3317907907837,-22.9991411291167,-7.32148036339021));
#10683=CARTESIAN_POINT('Ctrl Pts',(81.3314807411988,-22.9497833657722,-7.32479315383826));
#10684=CARTESIAN_POINT('Ctrl Pts',(81.3334814629917,-22.9004510906902,-7.32810594428632));
#10685=CARTESIAN_POINT('Ctrl Pts',(81.337874792749,-22.851332821333,-7.33141873473437));
#10686=CARTESIAN_POINT('Ctrl Pts',(81.3870020005563,-22.302081215111,-7.36846310739822));
#10687=CARTESIAN_POINT('Ctrl Pts',(81.7353061391843,-21.7795893526127,-7.40550748006207));
#10688=CARTESIAN_POINT('Ctrl Pts',(82.223396212068,-21.5229595829052,-7.44255185272593));
#10689=CARTESIAN_POINT('Ctrl Pts',(82.7114862849517,-21.2663298131978,-7.47959622538978));
#10690=CARTESIAN_POINT('Ctrl Pts',(83.339362292091,-21.2755621362812,-7.51664059805363));
#10691=CARTESIAN_POINT('Ctrl Pts',(83.8196959004573,-21.5464317645881,-7.55368497071749));
#10692=CARTESIAN_POINT('Ctrl Pts',(84.3000295088237,-21.8173013928951,-7.59072934338134));
#10693=CARTESIAN_POINT('Ctrl Pts',(84.6328207184171,-22.3498083264256,-7.62777371604519));
#10694=CARTESIAN_POINT('Ctrl Pts',(84.6657776801849,-22.9002668600333,-7.66481808870904));
#10695=CARTESIAN_POINT('Ctrl Pts',(84.6987346419527,-23.450725393641,-7.7018624613729));
#10696=CARTESIAN_POINT('Ctrl Pts',(84.4318573558949,-24.0191355273259,-7.73890683403675));
#10697=CARTESIAN_POINT('Ctrl Pts',(83.9872741414016,-24.3453816241485,-7.77595120670061));
#10698=CARTESIAN_POINT('Ctrl Pts',(83.5426909269083,-24.6716277209712,-7.81299557936446));
#10699=CARTESIAN_POINT('Ctrl Pts',(82.9204017839794,-24.7557097809315,-7.85003995202831));
#10700=CARTESIAN_POINT('Ctrl Pts',(82.4051784603229,-24.5591501854178,-7.88708432469216));
#10701=CARTESIAN_POINT('Ctrl Pts',(81.8899551366663,-24.362590589904,-7.92412869735602));
#10702=CARTESIAN_POINT('Ctrl Pts',(81.4817976322821,-23.8853893389161,-7.96117307001987));
#10703=CARTESIAN_POINT('Ctrl Pts',(81.3674868589662,-23.3459231227812,-7.99821744268372));
#10704=CARTESIAN_POINT('Ctrl Pts',(81.3435587761084,-23.2329994503731,-8.00597174958589));
#10705=CARTESIAN_POINT('Ctrl Pts',(81.332506141154,-23.1173475212576,-8.01372605648805));
#10706=CARTESIAN_POINT('Ctrl Pts',(81.3335753931735,-23.0014929636922,-8.02148036339021));
#10707=CARTESIAN_POINT('Ctrl Pts',(81.3366058837444,-23.0004198226253,-7.82851963660979));
#10708=CARTESIAN_POINT('Ctrl Pts',(81.3360372764733,-23.2525303502769,-7.81172305369484));
#10709=CARTESIAN_POINT('Ctrl Pts',(81.3897675507874,-23.5044108638859,-7.79492647077989));
#10710=CARTESIAN_POINT('Ctrl Pts',(81.4990409610885,-23.7293034217695,-7.77812988786494));
#10711=CARTESIAN_POINT('Ctrl Pts',(81.7400402735046,-24.2252973846937,-7.74108551520109));
#10712=CARTESIAN_POINT('Ctrl Pts',(82.2512070269747,-24.5900191965585,-7.70404114253724));
#10713=CARTESIAN_POINT('Ctrl Pts',(82.7986212649283,-24.6565651134249,-7.66699676987338));
#10714=CARTESIAN_POINT('Ctrl Pts',(83.3460355028819,-24.7231110302912,-7.62995239720953));
#10715=CARTESIAN_POINT('Ctrl Pts',(83.929697225319,-24.4914810521591,-7.59290802454568));
#10716=CARTESIAN_POINT('Ctrl Pts',(84.282511322795,-24.067673346594,-7.55586365188182));
#10717=CARTESIAN_POINT('Ctrl Pts',(84.635325420271,-23.6438656410289,-7.51881927921797));
#10718=CARTESIAN_POINT('Ctrl Pts',(84.7572918927858,-23.0278802080309,-7.48177490655412));
#10719=CARTESIAN_POINT('Ctrl Pts',(84.5925965199425,-22.5016046403627,-7.44473053389027));
#10720=CARTESIAN_POINT('Ctrl Pts',(84.4279011470992,-21.9753290726945,-7.40768616122642));
#10721=CARTESIAN_POINT('Ctrl Pts',(83.9765439288979,-21.5387633703561,-7.37064178856256));
#10722=CARTESIAN_POINT('Ctrl Pts',(83.4450747358265,-21.3916875211121,-7.33359741589871));
#10723=CARTESIAN_POINT('Ctrl Pts',(82.9136055427551,-21.2446116718681,-7.29655304323486));
#10724=CARTESIAN_POINT('Ctrl Pts',(82.3020243748137,-21.3870256757184,-7.259508670571));
#10725=CARTESIAN_POINT('Ctrl Pts',(81.8902029601806,-21.7537602138678,-7.22246429790715));
#10726=CARTESIAN_POINT('Ctrl Pts',(81.5420761010417,-22.0637735797765,-7.19114941080803));
#10727=CARTESIAN_POINT('Ctrl Pts',(81.3366956550969,-22.5340842585654,-7.15983452370891));
#10728=CARTESIAN_POINT('Ctrl Pts',(81.3326823670782,-23.0013023207031,-7.12851963660979));
#10729=CARTESIAN_POINT('Origin',(83.,-23.,-12.));
#10730=CARTESIAN_POINT('',(81.3325225746862,-22.9987867636662,-6.42851963660979));
#10731=CARTESIAN_POINT('',(81.3361555725406,-22.9990558295284,-6.62148036339021));
#10732=CARTESIAN_POINT('',(81.334,-23.,-12.));
#10733=CARTESIAN_POINT('',(84.2690708798524,-21.9206413469515,-6.));
#10734=CARTESIAN_POINT('Ctrl Pts',(81.3325225746862,-22.9987867636662,-6.42851963660979));
#10735=CARTESIAN_POINT('Ctrl Pts',(81.3364572466955,-23.4716253593496,-6.39681287573142));
#10736=CARTESIAN_POINT('Ctrl Pts',(81.547620038085,-23.9474489563196,-6.36510611485305));
#10737=CARTESIAN_POINT('Ctrl Pts',(81.903404325475,-24.2577326133438,-6.33339935397467));
#10738=CARTESIAN_POINT('Ctrl Pts',(82.3190824132044,-24.6202503573164,-6.29635498131082));
#10739=CARTESIAN_POINT('Ctrl Pts',(82.9321725171365,-24.7568018776601,-6.25931060864697));
#10740=CARTESIAN_POINT('Ctrl Pts',(83.462047088432,-24.6038092974618,-6.22226623598312));
#10741=CARTESIAN_POINT('Ctrl Pts',(83.9919216597275,-24.4508167172636,-6.18522186331926));
#10742=CARTESIAN_POINT('Ctrl Pts',(84.4385806983865,-24.0082800365234,-6.14817749065541));
#10743=CARTESIAN_POINT('Ctrl Pts',(84.5975922580266,-23.4812307285184,-6.11113311799156));
#10744=CARTESIAN_POINT('Ctrl Pts',(84.7566038176667,-22.9541814205133,-6.0740887453277));
#10745=CARTESIAN_POINT('Ctrl Pts',(84.627967898288,-22.3426194852432,-6.03704437266385));
#10746=CARTESIAN_POINT('Ctrl Pts',(84.2690708798524,-21.9206413469515,-6.));
#10747=CARTESIAN_POINT('',(81.7285275672489,-21.9187953038495,-6.));
#10748=CARTESIAN_POINT('Origin',(83.,-23.,-6.));
#10749=CARTESIAN_POINT('Ctrl Pts',(81.7285261019851,-21.9187941775198,-6.));
#10750=CARTESIAN_POINT('Ctrl Pts',(82.0793422764381,-21.5073246555327,-6.03631814560907));
#10751=CARTESIAN_POINT('Ctrl Pts',(82.6492094739697,-21.281282050469,-6.07263629121814));
#10752=CARTESIAN_POINT('Ctrl Pts',(83.1865491620181,-21.3418040640572,-6.10895443682721));
#10753=CARTESIAN_POINT('Ctrl Pts',(83.7346336337695,-21.403536291519,-6.14599880949106));
#10754=CARTESIAN_POINT('Ctrl Pts',(84.2488767328762,-21.7634081614138,-6.18304318215492));
#10755=CARTESIAN_POINT('Ctrl Pts',(84.4942853325427,-22.257154116884,-6.22008755481877));
#10756=CARTESIAN_POINT('Ctrl Pts',(84.7396939322092,-22.7509000723541,-6.25713192748263));
#10757=CARTESIAN_POINT('Ctrl Pts',(84.7162680324355,-23.3785201133997,-6.29417630014648));
#10758=CARTESIAN_POINT('Ctrl Pts',(84.4345602306372,-23.8525938579917,-6.33122067281033));
#10759=CARTESIAN_POINT('Ctrl Pts',(84.1528524288388,-24.3266676025837,-6.36826504547418));
#10760=CARTESIAN_POINT('Ctrl Pts',(83.6128627250159,-24.6471950507222,-6.40530941813804));
#10761=CARTESIAN_POINT('Ctrl Pts',(83.0617850263329,-24.6676013026721,-6.44235379080189));
#10762=CARTESIAN_POINT('Ctrl Pts',(82.5107073276499,-24.6880075546221,-6.47939816346575));
#10763=CARTESIAN_POINT('Ctrl Pts',(81.948541634107,-24.4082926103835,-6.5164425361296));
#10764=CARTESIAN_POINT('Ctrl Pts',(81.6325039196586,-23.9564070095206,-6.55348690879346));
#10765=CARTESIAN_POINT('Ctrl Pts',(81.4391457526553,-23.6799344004507,-6.57615139365904));
#10766=CARTESIAN_POINT('Ctrl Pts',(81.337919098353,-23.3390142503256,-6.59881587852463));
#10767=CARTESIAN_POINT('Ctrl Pts',(81.3361555725406,-22.9990558295284,-6.62148036339021));
#10768=CARTESIAN_POINT('Origin',(83.,-23.,-4.45407471946233));
#10769=CARTESIAN_POINT('',(80.9445918241665,-22.9981768120733,-16.6459252805377));
#10770=CARTESIAN_POINT('',(80.9470732705607,-23.0015060107516,-16.7040747194623));
#10771=CARTESIAN_POINT('',(80.94525,-22.9999999999999,-4.45407471946233));
#10772=CARTESIAN_POINT('',(84.8174278887595,-22.0413794120407,-17.));
#10773=CARTESIAN_POINT('Ctrl Pts',(80.9470732705607,-23.0015060107516,-16.7040747194623));
#10774=CARTESIAN_POINT('Ctrl Pts',(80.9500635605842,-22.5475808384988,-16.7286277343139));
#10775=CARTESIAN_POINT('Ctrl Pts',(81.3216916635813,-21.4040173658448,-16.7902251218292));
#10776=CARTESIAN_POINT('Ctrl Pts',(83.2159924080748,-20.5820415540093,-16.8888668820084));
#10777=CARTESIAN_POINT('Ctrl Pts',(84.4986774253636,-21.4370673526013,-16.9629556273361));
#10778=CARTESIAN_POINT('Ctrl Pts',(84.8174278887595,-22.0413794120407,-17.));
#10779=CARTESIAN_POINT('',(85.0570979189415,-23.0754558306091,-17.));
#10780=CARTESIAN_POINT('Origin',(83.,-23.,-17.));
#10781=CARTESIAN_POINT('Ctrl Pts',(80.9445918241665,-22.9981768120733,-16.6459252805377));
#10782=CARTESIAN_POINT('Ctrl Pts',(80.9432972488844,-22.8578132508263,-16.6535432960884));
#10783=CARTESIAN_POINT('Ctrl Pts',(81.020425579335,-22.0363086702384,-16.6982056843029));
#10784=CARTESIAN_POINT('Ctrl Pts',(82.1263744182192,-20.7340408632062,-16.7799124451812));
#10785=CARTESIAN_POINT('Ctrl Pts',(84.4138509810425,-21.0348853436204,-16.890319336118));
#10786=CARTESIAN_POINT('Ctrl Pts',(85.0806816672165,-22.4089784863789,-16.9636818543909));
#10787=CARTESIAN_POINT('Ctrl Pts',(85.0571001899048,-23.0754560264203,-17.));
#10788=CARTESIAN_POINT('Origin',(83.,-23.,-4.45407471946233));
#10789=CARTESIAN_POINT('',(80.9485827974856,-23.0000495903536,-15.9459252805377));
#10790=CARTESIAN_POINT('',(80.9419860077008,-23.0004830909235,-16.0040747194623));
#10791=CARTESIAN_POINT('',(80.94525,-22.9999999999999,-4.45407471946233));
#10792=CARTESIAN_POINT('Ctrl Pts',(80.9419860077008,-23.0004830909235,-16.0040747194623));
#10793=CARTESIAN_POINT('Ctrl Pts',(80.9440550409229,-22.346392379771,-16.0396948316641));
#10794=CARTESIAN_POINT('Ctrl Pts',(81.6350687429363,-21.0082839131029,-16.1123593165297));
#10795=CARTESIAN_POINT('Ctrl Pts',(83.9141747133152,-20.7500128153374,-16.2220681740591));
#10796=CARTESIAN_POINT('Ctrl Pts',(85.3860298428717,-22.5475930446421,-16.3332012920507));
#10797=CARTESIAN_POINT('Ctrl Pts',(84.6743955395297,-24.7593786616575,-16.4443344100422));
#10798=CARTESIAN_POINT('Ctrl Pts',(82.4296922229958,-25.3606230541752,-16.5554675280338));
#10799=CARTESIAN_POINT('Ctrl Pts',(81.0884939258943,-24.1462800951831,-16.6420476311738));
#10800=CARTESIAN_POINT('Ctrl Pts',(80.9455519591099,-23.2324406548646,-16.69158336165));
#10801=CARTESIAN_POINT('Ctrl Pts',(80.9470732705607,-23.0015060107516,-16.7040747194623));
#10802=CARTESIAN_POINT('Ctrl Pts',(80.9485827974856,-23.0000495903536,-15.9459252805377));
#10803=CARTESIAN_POINT('Ctrl Pts',(80.9486568158977,-22.6540999364258,-15.9646103934386));
#10804=CARTESIAN_POINT('Ctrl Pts',(81.195745621415,-21.6221842533796,-16.0203398790033));
#10805=CARTESIAN_POINT('Ctrl Pts',(82.8298598709625,-20.5773510168392,-16.1131137372319));
#10806=CARTESIAN_POINT('Ctrl Pts',(84.9430514548956,-21.5430599298187,-16.2242468552234));
#10807=CARTESIAN_POINT('Ctrl Pts',(85.2779271980639,-23.842211340369,-16.335379973215));
#10808=CARTESIAN_POINT('Ctrl Pts',(83.5278718822138,-25.37055054633,-16.4465130912065));
#10809=CARTESIAN_POINT('Ctrl Pts',(81.4479221613014,-24.7732038337887,-16.5500281936475));
#10810=CARTESIAN_POINT('Ctrl Pts',(80.9495924223287,-23.5403637177663,-16.6164989234245));
#10811=CARTESIAN_POINT('Ctrl Pts',(80.9445918241665,-22.9981768120733,-16.6459252805377));
#10812=CARTESIAN_POINT('Origin',(83.,-23.,-4.45407471946233));
#10813=CARTESIAN_POINT('',(80.9444683918153,-23.0018063316281,-15.2459252805377));
#10814=CARTESIAN_POINT('',(80.9457761200516,-22.9981345158697,-15.3040747194623));
#10815=CARTESIAN_POINT('',(80.94525,-22.9999999999999,-4.45407471946233));
#10816=CARTESIAN_POINT('Ctrl Pts',(80.9457761200516,-22.9981345158697,-15.3040747194623));
#10817=CARTESIAN_POINT('Ctrl Pts',(80.9441910027471,-22.8202139788124,-15.3137175563504));
#10818=CARTESIAN_POINT('Ctrl Pts',(81.0468090685297,-21.9605854226314,-15.3604047659024));
#10819=CARTESIAN_POINT('Ctrl Pts',(82.2507940745424,-20.6898346105816,-15.4441363481181));
#10820=CARTESIAN_POINT('Ctrl Pts',(84.5344925201404,-21.1175797670015,-15.5552694661097));
#10821=CARTESIAN_POINT('Ctrl Pts',(85.4137606299914,-23.2681888577979,-15.6664025841013));
#10822=CARTESIAN_POINT('Ctrl Pts',(84.0838647611703,-25.1733432517703,-15.7775357020929));
#10823=CARTESIAN_POINT('Ctrl Pts',(81.7619637210983,-25.0893637699614,-15.8886688200844));
#10824=CARTESIAN_POINT('Ctrl Pts',(80.9542067795097,-23.7329548423873,-15.9641818258742));
#10825=CARTESIAN_POINT('Ctrl Pts',(80.9419032779722,-23.0266367294426,-16.0026504590002));
#10826=CARTESIAN_POINT('Ctrl Pts',(80.9419860077008,-23.0004830909235,-16.0040747194623));
#10827=CARTESIAN_POINT('Ctrl Pts',(80.9444683918153,-23.0018063316281,-15.2459252805377));
#10828=CARTESIAN_POINT('Ctrl Pts',(80.949498810733,-22.4537399021428,-15.2756774907888));
#10829=CARTESIAN_POINT('Ctrl Pts',(81.4568946252713,-21.2150551659787,-15.3424740737037));
#10830=CARTESIAN_POINT('Ctrl Pts',(83.5486977575985,-20.6341799887301,-15.4463150292825));
#10831=CARTESIAN_POINT('Ctrl Pts',(85.2852062676543,-22.1778048794721,-15.5574481472741));
#10832=CARTESIAN_POINT('Ctrl Pts',(84.9302047132626,-24.4739350041461,-15.6685812652656));
#10833=CARTESIAN_POINT('Ctrl Pts',(82.8086025236948,-25.4210620022677,-15.7797143832572));
#10834=CARTESIAN_POINT('Ctrl Pts',(81.1894351825912,-24.3656514787605,-15.8721623883479));
#10835=CARTESIAN_POINT('Ctrl Pts',(80.9485100698943,-23.3399661643164,-15.9275660207747));
#10836=CARTESIAN_POINT('Ctrl Pts',(80.9485827974856,-23.0000495903536,-15.9459252805377));
#10837=CARTESIAN_POINT('Origin',(83.,-23.,-4.45407471946233));
#10838=CARTESIAN_POINT('',(80.9427068937054,-22.9988171296078,-14.5459252805377));
#10839=CARTESIAN_POINT('',(80.9483912189187,-23.0006513925548,-14.6040747194623));
#10840=CARTESIAN_POINT('',(80.94525,-22.9999999999999,-4.45407471946233));
#10841=CARTESIAN_POINT('Ctrl Pts',(80.9483912189187,-23.0006513925548,-14.6040747194623));
#10842=CARTESIAN_POINT('Ctrl Pts',(80.9494812471314,-22.6173024205259,-14.6247846537006));
#10843=CARTESIAN_POINT('Ctrl Pts',(81.2366609896803,-21.5467311614289,-14.6825389606028));
#10844=CARTESIAN_POINT('Ctrl Pts',(82.9621345897233,-20.571679876643,-14.7773376401688));
#10845=CARTESIAN_POINT('Ctrl Pts',(85.0195746168704,-21.6511149812732,-14.8884707581604));
#10846=CARTESIAN_POINT('Ctrl Pts',(85.2286204270596,-23.9651027282846,-14.9996038761519));
#10847=CARTESIAN_POINT('Ctrl Pts',(83.397945180368,-25.3957905088984,-15.1107369941435));
#10848=CARTESIAN_POINT('Ctrl Pts',(81.3935017093533,-24.699876881042,-15.2122272752469));
#10849=CARTESIAN_POINT('Ctrl Pts',(80.9502804634345,-23.5037218257036,-15.2766731836866));
#10850=CARTESIAN_POINT('Ctrl Pts',(80.9457761200516,-22.9981345158697,-15.3040747194623));
#10851=CARTESIAN_POINT('Ctrl Pts',(80.9427068937054,-22.9988171296078,-14.5459252805377));
#10852=CARTESIAN_POINT('Ctrl Pts',(80.9422306998785,-22.9294336755561,-14.5497002154751));
#10853=CARTESIAN_POINT('Ctrl Pts',(80.976896368521,-22.1796546331155,-14.5905195230764));
#10854=CARTESIAN_POINT('Ctrl Pts',(81.896614425227,-20.83650429601,-14.6683832033416));
#10855=CARTESIAN_POINT('Ctrl Pts',(84.2191696850261,-20.8995717888251,-14.7795163213332));
#10856=CARTESIAN_POINT('Ctrl Pts',(85.4258928578083,-22.8850338533659,-14.8906494393247));
#10857=CARTESIAN_POINT('Ctrl Pts',(84.4123434153425,-24.9757174587147,-15.0017825573163));
#10858=CARTESIAN_POINT('Ctrl Pts',(82.1061616690569,-25.2581466855875,-15.1129156753078));
#10859=CARTESIAN_POINT('Ctrl Pts',(81.0164469782457,-23.9515225379254,-15.1942965830483));
#10860=CARTESIAN_POINT('Ctrl Pts',(80.9432354537767,-23.1361354918168,-15.2386331181249));
#10861=CARTESIAN_POINT('Ctrl Pts',(80.9444683918153,-23.0018063316281,-15.2459252805377));
#10862=CARTESIAN_POINT('Origin',(83.,-23.,-4.45407471946233));
#10863=CARTESIAN_POINT('',(80.9480449299229,-22.998944875009,-13.8459252805377));
#10864=CARTESIAN_POINT('',(80.9433899630638,-23.0015207493961,-13.9040747194623));
#10865=CARTESIAN_POINT('',(80.94525,-22.9999999999999,-4.45407471946233));
#10866=CARTESIAN_POINT('Ctrl Pts',(80.9433899630638,-23.0015207493961,-13.9040747194623));
#10867=CARTESIAN_POINT('Ctrl Pts',(80.9482330971096,-22.4169498138078,-13.9358517510509));
#10868=CARTESIAN_POINT('Ctrl Pts',(81.5151172915851,-21.142699823015,-14.0046731553033));
#10869=CARTESIAN_POINT('Ctrl Pts',(83.6768128836446,-20.6675985082928,-14.1105389322194));
#10870=CARTESIAN_POINT('Ctrl Pts',(85.326617632413,-22.3035642232594,-14.221672050211));
#10871=CARTESIAN_POINT('Ctrl Pts',(84.8470103486162,-24.5769353722521,-14.3328051682026));
#10872=CARTESIAN_POINT('Ctrl Pts',(82.6769464973495,-25.4070332015704,-14.4439382861941));
#10873=CARTESIAN_POINT('Ctrl Pts',(81.1518516642612,-24.2899654019874,-14.5343614699474));
#10874=CARTESIAN_POINT('Ctrl Pts',(80.9475314866512,-23.3030082280256,-14.5877402810368));
#10875=CARTESIAN_POINT('Ctrl Pts',(80.9483912189187,-23.0006513925548,-14.6040747194623));
#10876=CARTESIAN_POINT('Ctrl Pts',(80.9480449299229,-22.9989448750091,-13.8459252805377));
#10877=CARTESIAN_POINT('Ctrl Pts',(80.9467671190122,-22.7243288838564,-13.8607673128254));
#10878=CARTESIAN_POINT('Ctrl Pts',(81.1259274427508,-21.7658950801937,-13.9126537177769));
#10879=CARTESIAN_POINT('Ctrl Pts',(82.5805008816194,-20.6078892424568,-14.0015844953923));
#10880=CARTESIAN_POINT('Ctrl Pts',(84.7821633068503,-21.3501311159715,-14.1127176133838));
#10881=CARTESIAN_POINT('Ctrl Pts',(85.3527197283046,-23.6023979303683,-14.2238507313754));
#10882=CARTESIAN_POINT('Ctrl Pts',(83.769974452434,-25.3033264487149,-14.3349838493669));
#10883=CARTESIAN_POINT('Ctrl Pts',(81.5602178471133,-24.9099904475101,-14.442342032421));
#10884=CARTESIAN_POINT('Ctrl Pts',(80.9469037079901,-23.6103107161358,-14.5126558428113));
#10885=CARTESIAN_POINT('Ctrl Pts',(80.9427068937054,-22.9988171296078,-14.5459252805377));
#10886=CARTESIAN_POINT('Origin',(83.,-23.,-4.45407471946233));
#10887=CARTESIAN_POINT('',(80.9465558469908,-23.0017537142658,-13.1459252805377));
#10888=CARTESIAN_POINT('',(80.9436612253546,-22.9983838582986,-13.2040747194623));
#10889=CARTESIAN_POINT('',(80.94525,-22.9999999999999,-4.45407471946233));
#10890=CARTESIAN_POINT('Ctrl Pts',(80.9436612253546,-22.9983838582986,-13.2040747194623));
#10891=CARTESIAN_POINT('Ctrl Pts',(80.9427400817188,-22.8916548014817,-13.2098744757372));
#10892=CARTESIAN_POINT('Ctrl Pts',(80.9988246572765,-22.1041931228359,-13.252718604676));
#10893=CARTESIAN_POINT('Ctrl Pts',(82.0161587924632,-20.7795881291394,-13.3326071062786));
#10894=CARTESIAN_POINT('Ctrl Pts',(84.3318253496949,-20.9691347568542,-13.4437402242701));
#10895=CARTESIAN_POINT('Ctrl Pts',(85.4285529267558,-23.0174091891753,-13.5548733422617));
#10896=CARTESIAN_POINT('Ctrl Pts',(84.3025732783284,-25.0497500463396,-13.6660064602532));
#10897=CARTESIAN_POINT('Ctrl Pts',(81.9844272968094,-25.2060789837275,-13.7771395782448));
#10898=CARTESIAN_POINT('Ctrl Pts',(80.9928404632344,-23.8759493553275,-13.8564956646478));
#10899=CARTESIAN_POINT('Ctrl Pts',(80.9425871681638,-23.098418865631,-13.898807378387));
#10900=CARTESIAN_POINT('Ctrl Pts',(80.9433899630638,-23.0015207493961,-13.9040747194623));
#10901=CARTESIAN_POINT('Ctrl Pts',(80.9465558469908,-23.0017537142658,-13.1459252805377));
#10902=CARTESIAN_POINT('Ctrl Pts',(80.9504435912746,-22.523241982595,-13.1718344101756));
#10903=CARTESIAN_POINT('Ctrl Pts',(81.3555436948577,-21.3546297745119,-13.2347879124773));
#10904=CARTESIAN_POINT('Ctrl Pts',(83.301369139264,-20.5901556007548,-13.3347857874429));
#10905=CARTESIAN_POINT('Ctrl Pts',(85.1880466821996,-21.946138005623,-13.4459189054345));
#10906=CARTESIAN_POINT('Ctrl Pts',(85.0721377809063,-24.2666563873492,-13.557052023426));
#10907=CARTESIAN_POINT('Ctrl Pts',(83.0597268239821,-25.4278809882634,-13.6681851414176));
#10908=CARTESIAN_POINT('Ctrl Pts',(81.2687132343068,-24.5086941725721,-13.7644762271215));
#10909=CARTESIAN_POINT('Ctrl Pts',(80.9499564196855,-23.4097456056731,-13.8237229401615));
#10910=CARTESIAN_POINT('Ctrl Pts',(80.9480449299229,-22.9989448750091,-13.8459252805377));
#10911=CARTESIAN_POINT('Origin',(83.,-23.,-4.45407471946233));
#10912=CARTESIAN_POINT('',(80.9418454336727,-23.0000233771379,-12.4459252805377));
#10913=CARTESIAN_POINT('',(80.9484735339094,-22.9995028191082,-12.5040747194623));
#10914=CARTESIAN_POINT('',(80.94525,-22.9999999999999,-4.45407471946233));
#10915=CARTESIAN_POINT('Ctrl Pts',(80.9484735339094,-22.9995028191082,-12.5040747194623));
#10916=CARTESIAN_POINT('Ctrl Pts',(80.9477974848827,-22.6872594927532,-12.5209415730874));
#10917=CARTESIAN_POINT('Ctrl Pts',(81.1614618092461,-21.6901193881101,-12.5748527993764));
#10918=CARTESIAN_POINT('Ctrl Pts',(82.711487771974,-20.588582762733,-12.6658083983292));
#10919=CARTESIAN_POINT('Ctrl Pts',(84.869428030581,-21.4497060806457,-12.7769415163207));
#10920=CARTESIAN_POINT('Ctrl Pts',(85.3163941756299,-23.7297194125255,-12.8880746343123));
#10921=CARTESIAN_POINT('Ctrl Pts',(83.6433051987559,-25.3418648165858,-12.9992077523039));
#10922=CARTESIAN_POINT('Ctrl Pts',(81.4994791114416,-24.8383664692076,-13.1045411140205));
#10923=CARTESIAN_POINT('Ctrl Pts',(80.9486236372523,-23.5733577502603,-13.1728301030734));
#10924=CARTESIAN_POINT('Ctrl Pts',(80.9436612253546,-22.9983838582986,-13.2040747194623));
#10925=CARTESIAN_POINT('Ctrl Pts',(80.94184556232,-23.0000233762546,-12.4459252805377));
#10926=CARTESIAN_POINT('Ctrl Pts',(80.9419597191148,-22.3211541232341,-12.4829015075258));
#10927=CARTESIAN_POINT('Ctrl Pts',(81.6804453873982,-20.9619516944595,-12.5569221071777));
#10928=CARTESIAN_POINT('Ctrl Pts',(83.9956695846244,-20.7848667162158,-12.6679870794935));
#10929=CARTESIAN_POINT('Ctrl Pts',(85.4010383313655,-22.6350502527901,-12.7791201974851));
#10930=CARTESIAN_POINT('Ctrl Pts',(84.6088822932929,-24.819250162293,-12.8902533154767));
#10931=CARTESIAN_POINT('Ctrl Pts',(82.3442138554089,-25.3384007182767,-13.0013864334682));
#10932=CARTESIAN_POINT('Ctrl Pts',(81.0677939069456,-24.0952790226387,-13.0866104218219));
#10933=CARTESIAN_POINT('Ctrl Pts',(80.9448849696581,-23.2074088056333,-13.1347900375117));
#10934=CARTESIAN_POINT('Ctrl Pts',(80.9465558469908,-23.0017537142658,-13.1459252805377));
#10935=CARTESIAN_POINT('Origin',(83.,-23.,-4.45407471946233));
#10936=CARTESIAN_POINT('',(80.9464876953405,-22.9982315273104,-11.7459252805377));
#10937=CARTESIAN_POINT('',(80.9454840271886,-23.0018778870529,-11.8040747194623));
#10938=CARTESIAN_POINT('',(80.94525,-22.9999999999999,-4.45407471946233));
#10939=CARTESIAN_POINT('Ctrl Pts',(80.9454840271886,-23.0018778870529,-11.8040747194623));
#10940=CARTESIAN_POINT('Ctrl Pts',(80.9501626083473,-22.486653624791,-11.8320086704377));
#10941=CARTESIAN_POINT('Ctrl Pts',(81.407470405066,-21.2807660753287,-11.8969869940768));
#10942=CARTESIAN_POINT('Ctrl Pts',(83.4322511364777,-20.6101608102379,-11.9990096903798));
#10943=CARTESIAN_POINT('Ctrl Pts',(85.2422274635415,-22.0669467326842,-12.1101428083714));
#10944=CARTESIAN_POINT('Ctrl Pts',(85.0000289627594,-24.3776997299966,-12.221275926363));
#10945=CARTESIAN_POINT('Ctrl Pts',(82.9273252348868,-25.4275277086832,-12.3324090443545));
#10946=CARTESIAN_POINT('Ctrl Pts',(81.2256188601819,-24.4334541577041,-12.426675308721));
#10947=CARTESIAN_POINT('Ctrl Pts',(80.9492822794177,-23.3730339946484,-12.4838972004236));
#10948=CARTESIAN_POINT('Ctrl Pts',(80.9484735339094,-22.9995028191082,-12.5040747194623));
#10949=CARTESIAN_POINT('Ctrl Pts',(80.9464876953406,-22.9982315273104,-11.7459252805377));
#10950=CARTESIAN_POINT('Ctrl Pts',(80.9448193421433,-22.7951106380881,-11.7569242322122));
#10951=CARTESIAN_POINT('Ctrl Pts',(81.0658211635465,-21.9098241257738,-11.8049675565505));
#10952=CARTESIAN_POINT('Ctrl Pts',(82.3356362554336,-20.6640217891469,-11.8900552535526));
#10953=CARTESIAN_POINT('Ctrl Pts',(84.6021947432545,-21.1748574325926,-12.0011883715442));
#10954=CARTESIAN_POINT('Ctrl Pts',(85.4023615402782,-23.356135390641,-12.1123214895358));
#10955=CARTESIAN_POINT('Ctrl Pts',(84.0037924996106,-25.2114642218224,-12.2234546075273));
#10956=CARTESIAN_POINT('Ctrl Pts',(81.6865130544115,-25.0427739548083,-12.3345877255189));
#10957=CARTESIAN_POINT('Ctrl Pts',(80.9424129421303,-23.6826458175463,-12.4087446165223));
#10958=CARTESIAN_POINT('Ctrl Pts',(80.9418453519337,-23.0012745045541,-12.4458571348619));
#10959=CARTESIAN_POINT('Ctrl Pts',(80.94184556232,-23.0000233762546,-12.4459252805377));
#10960=CARTESIAN_POINT('Origin',(83.,-23.,-4.45407471946233));
#10961=CARTESIAN_POINT('',(80.948083343573,-23.001020415448,-11.0459252805377));
#10962=CARTESIAN_POINT('',(80.9420996930937,-22.9993455607543,-11.1040747194623));
#10963=CARTESIAN_POINT('',(80.94525,-22.9999999999999,-4.45407471946233));
#10964=CARTESIAN_POINT('Ctrl Pts',(80.9420996930937,-22.9993455607543,-11.1040747194623));
#10965=CARTESIAN_POINT('Ctrl Pts',(80.9419498972546,-22.9634098758055,-11.106031395124));
#10966=CARTESIAN_POINT('Ctrl Pts',(80.959087622844,-22.2472747969947,-11.1450324434495));
#10967=CARTESIAN_POINT('Ctrl Pts',(81.7920501260224,-20.8930995515055,-11.2210778644389));
#10968=CARTESIAN_POINT('Ctrl Pts',(84.1149085188063,-20.8424200147847,-11.3322109824305));
#10969=CARTESIAN_POINT('Ctrl Pts',(85.4173587528071,-22.7664426020535,-11.443344100422));
#10970=CARTESIAN_POINT('Ctrl Pts',(84.5073471099255,-24.9042261126527,-11.5544772184136));
#10971=CARTESIAN_POINT('Ctrl Pts',(82.2177520634359,-25.2991869353425,-11.6656103364051));
#10972=CARTESIAN_POINT('Ctrl Pts',(81.039647370209,-24.0194952561807,-11.7488095034214));
#10973=CARTESIAN_POINT('Ctrl Pts',(80.9439581475414,-23.1699139195325,-11.7949642977738));
#10974=CARTESIAN_POINT('Ctrl Pts',(80.9454840271886,-23.0018778870529,-11.8040747194623));
#10975=CARTESIAN_POINT('Ctrl Pts',(80.948083343573,-23.001020415448,-11.0459252805377));
#10976=CARTESIAN_POINT('Ctrl Pts',(80.9499185724722,-22.5927222976639,-11.0679913295624));
#10977=CARTESIAN_POINT('Ctrl Pts',(81.2657181572716,-21.4963595529218,-11.1271017512509));
#10978=CARTESIAN_POINT('Ctrl Pts',(83.0508160094325,-20.571916162926,-11.2232565456033));
#10979=CARTESIAN_POINT('Ctrl Pts',(85.0674751504547,-21.7257473213969,-11.3343896635948));
#10980=CARTESIAN_POINT('Ctrl Pts',(85.1918996587519,-24.0458246854221,-11.4455227815864));
#10981=CARTESIAN_POINT('Ctrl Pts',(83.3102113270295,-25.4087221340905,-11.556655899578));
#10982=CARTESIAN_POINT('Ctrl Pts',(81.3589374844954,-24.6503621653507,-11.656790065895));
#10983=CARTESIAN_POINT('Ctrl Pts',(80.9504383410627,-23.4792200094962,-11.7198798595483));
#10984=CARTESIAN_POINT('Ctrl Pts',(80.9464876953406,-22.9982315273104,-11.7459252805377));
#10985=CARTESIAN_POINT('Origin',(83.,-23.,-4.45407471946233));
#10986=CARTESIAN_POINT('',(80.9427634779915,-23.0012177328999,-10.3459252805377));
#10987=CARTESIAN_POINT('',(80.9474131382961,-22.998536475434,-10.4040747194623));
#10988=CARTESIAN_POINT('',(80.94525,-22.9999999999999,-4.45407471946233));
#10989=CARTESIAN_POINT('Ctrl Pts',(80.9474131382961,-22.998536475434,-10.4040747194623));
#10990=CARTESIAN_POINT('Ctrl Pts',(80.9458280534013,-22.7577490701563,-10.4170984924742));
#10991=CARTESIAN_POINT('Ctrl Pts',(81.0963188906304,-21.8339922531296,-10.46716663815));
#10992=CARTESIAN_POINT('Ctrl Pts',(82.4639279853743,-20.6312874397589,-10.5542791564896));
#10993=CARTESIAN_POINT('Ctrl Pts',(84.699278862516,-21.2648850916105,-10.6654122744811));
#10994=CARTESIAN_POINT('Ctrl Pts',(85.3793828417187,-23.4865282010775,-10.7765453924727));
#10995=CARTESIAN_POINT('Ctrl Pts',(83.8817819925845,-25.2628815513549,-10.8876785104643));
#10996=CARTESIAN_POINT('Ctrl Pts',(81.6177164603555,-24.973345741473,-10.9968549527941));
#10997=CARTESIAN_POINT('Ctrl Pts',(80.9447858771748,-23.6437550813218,-11.0689870224602));
#10998=CARTESIAN_POINT('Ctrl Pts',(80.9420996930937,-22.9993455607543,-11.1040747194623));
#10999=CARTESIAN_POINT('Ctrl Pts',(80.9427634779915,-23.0012177328999,-10.3459252805377));
#11000=CARTESIAN_POINT('Ctrl Pts',(80.9470399224638,-22.3921851286143,-10.3790584269126));
#11001=CARTESIAN_POINT('Ctrl Pts',(81.5560212459934,-21.0947968361722,-10.4492359459513));
#11002=CARTESIAN_POINT('Ctrl Pts',(83.7615159742851,-20.6938632287777,-10.5564578376539));
#11003=CARTESIAN_POINT('Ctrl Pts',(85.3504930611994,-22.3889715588227,-10.6675909556455));
#11004=CARTESIAN_POINT('Ctrl Pts',(84.7882063839989,-24.6433171680781,-10.778724073637));
#11005=CARTESIAN_POINT('Ctrl Pts',(82.5892828410451,-25.3936342247751,-10.8898571916286));
#11006=CARTESIAN_POINT('Ctrl Pts',(81.1282335614878,-24.2392080086894,-10.9789242605955));
#11007=CARTESIAN_POINT('Ctrl Pts',(80.9468375993813,-23.278171134301,-11.0309469568985));
#11008=CARTESIAN_POINT('Ctrl Pts',(80.948083343573,-23.001020415448,-11.0459252805377));
#11009=CARTESIAN_POINT('Origin',(83.,-23.,-4.45407471946233));
#11010=CARTESIAN_POINT('',(80.944392748711,-22.9982061753951,-9.64592528053768));
#11011=CARTESIAN_POINT('',(80.9473845690181,-23.0014769893773,-9.70407471946233));
#11012=CARTESIAN_POINT('',(80.94525,-22.9999999999999,-4.45407471946233));
#11013=CARTESIAN_POINT('Ctrl Pts',(80.9473845690181,-23.0014769893773,-9.70407471946233));
#11014=CARTESIAN_POINT('Ctrl Pts',(80.9503462238683,-22.5560933688278,-9.72816558982444));
#11015=CARTESIAN_POINT('Ctrl Pts',(81.3116443464902,-21.4214699850473,-9.78930083285041));
#11016=CARTESIAN_POINT('Ctrl Pts',(83.1830643685562,-20.5782940238596,-9.88748044854021));
#11017=CARTESIAN_POINT('Ctrl Pts',(85.1338458058857,-21.8403127686255,-9.99861356653179));
#11018=CARTESIAN_POINT('Ctrl Pts',(85.131647574316,-24.1637229123899,-10.1097466845233));
#11019=CARTESIAN_POINT('Ctrl Pts',(83.1784815819015,-25.4220480430476,-10.2208798025149));
#11020=CARTESIAN_POINT('Ctrl Pts',(81.3099987037936,-24.5759384329199,-10.3189891474946));
#11021=CARTESIAN_POINT('Ctrl Pts',(80.9503366144376,-23.4426364960753,-10.3800541198104));
#11022=CARTESIAN_POINT('Ctrl Pts',(80.9474131382961,-22.998536475434,-10.4040747194623));
#11023=CARTESIAN_POINT('Ctrl Pts',(80.944392748711,-22.9982061753951,-9.64592528053768));
#11024=CARTESIAN_POINT('Ctrl Pts',(80.9431863080667,-22.8664001375128,-9.65308115159894));
#11025=CARTESIAN_POINT('Ctrl Pts',(81.014785138996,-22.053568649942,-9.69728139532405));
#11026=CARTESIAN_POINT('Ctrl Pts',(82.0978802191083,-20.7451489433667,-9.77852601171301));
#11027=CARTESIAN_POINT('Ctrl Pts',(84.4050829423841,-21.0191124939321,-9.88965912970458));
#11028=CARTESIAN_POINT('Ctrl Pts',(85.4262984532635,-23.1060622570228,-10.0007922476961));
#11029=CARTESIAN_POINT('Ctrl Pts',(84.2268701215403,-25.0959396679168,-10.1119253656877));
#11030=CARTESIAN_POINT('Ctrl Pts',(81.9045619654454,-25.1675305993517,-10.2230584836792));
#11031=CARTESIAN_POINT('Ctrl Pts',(80.9783022134605,-23.8254196017566,-10.3010584552959));
#11032=CARTESIAN_POINT('Ctrl Pts',(80.9422586620029,-23.0731114282876,-10.3420140542487));
#11033=CARTESIAN_POINT('Ctrl Pts',(80.9427634779915,-23.0012177328999,-10.3459252805377));
#11034=CARTESIAN_POINT('Origin',(83.,-23.,-4.45407471946233));
#11035=CARTESIAN_POINT('',(80.9485808123477,-22.9999091152425,-8.94592528053768));
#11036=CARTESIAN_POINT('',(80.9420825813087,-23.0006320364948,-9.00407471946233));
#11037=CARTESIAN_POINT('',(80.94525,-22.9999999999999,-4.45407471946233));
#11038=CARTESIAN_POINT('Ctrl Pts',(80.9420825813087,-23.0006320364948,-9.00407471946233));
#11039=CARTESIAN_POINT('Ctrl Pts',(80.9446924463348,-22.3549462619531,-9.03923268717465));
#11040=CARTESIAN_POINT('Ctrl Pts',(81.6199953858007,-21.024225773533,-9.11143502755082));
#11041=CARTESIAN_POINT('Ctrl Pts',(83.886062338264,-20.7387910466673,-9.22068174059087));
#11042=CARTESIAN_POINT('Ctrl Pts',(85.3802992120524,-22.517975043166,-9.33181485858242));
#11043=CARTESIAN_POINT('Ctrl Pts',(84.695992559306,-24.7383272524714,-9.44294797657398));
#11044=CARTESIAN_POINT('Ctrl Pts',(82.4594467626664,-25.3676939404236,-9.55408109456554));
#11045=CARTESIAN_POINT('Ctrl Pts',(81.0952172934861,-24.1633756968917,-9.64112334219499));
#11046=CARTESIAN_POINT('Ctrl Pts',(80.9457921067143,-23.2409568283049,-9.69112121716059));
#11047=CARTESIAN_POINT('Ctrl Pts',(80.9473845690181,-23.0014769893773,-9.70407471946233));
#11048=CARTESIAN_POINT('Ctrl Pts',(80.9485808123477,-22.9999091152425,-8.94592528053768));
#11049=CARTESIAN_POINT('Ctrl Pts',(80.9484476854599,-22.6625169408995,-8.96414824894915));
#11050=CARTESIAN_POINT('Ctrl Pts',(81.1868156284612,-21.6394377060121,-9.01941559002448));
#11051=CARTESIAN_POINT('Ctrl Pts',(82.7997191561016,-20.5796568486397,-9.11172730376366));
#11052=CARTESIAN_POINT('Ctrl Pts',(84.9247819526336,-21.5189909448313,-9.22286042175521));
#11053=CARTESIAN_POINT('Ctrl Pts',(85.2882085474095,-23.8138028202287,-9.33399353974677));
#11054=CARTESIAN_POINT('Ctrl Pts',(83.5573766165987,-25.3637903236025,-9.44512665773833));
#11055=CARTESIAN_POINT('Ctrl Pts',(81.460707594627,-24.7898437540697,-9.54910390466863));
#11056=CARTESIAN_POINT('Ctrl Pts',(80.949431786282,-23.5487310438219,-9.61603677893508));
#11057=CARTESIAN_POINT('Ctrl Pts',(80.944392748711,-22.9982061753951,-9.64592528053768));
#11058=CARTESIAN_POINT('Origin',(83.,-23.,-4.45407471946233));
#11059=CARTESIAN_POINT('',(80.9447263139995,-23.0018413368225,-8.24592528053768));
#11060=CARTESIAN_POINT('',(80.9455228522428,-22.9981228933243,-8.30407471946232));
#11061=CARTESIAN_POINT('',(80.94525,-22.9999999999999,-4.45407471946233));
#11062=CARTESIAN_POINT('Ctrl Pts',(80.9455228522428,-22.9981228933243,-8.30407471946232));
#11063=CARTESIAN_POINT('Ctrl Pts',(80.9439883710969,-22.8287825981896,-8.31325541186101));
#11064=CARTESIAN_POINT('Ctrl Pts',(81.0405829332249,-21.9778760562739,-8.35948047692355));
#11065=CARTESIAN_POINT('Ctrl Pts',(82.2221040868968,-20.6993369771883,-8.44274991464995));
#11066=CARTESIAN_POINT('Ctrl Pts',(84.5109476719975,-21.0986295650073,-8.55388303264151));
#11067=CARTESIAN_POINT('Ctrl Pts',(85.4169124774121,-23.2381312128108,-8.66501615063307));
#11068=CARTESIAN_POINT('Ctrl Pts',(84.1108238547277,-25.1596858015617,-8.77614926862463));
#11069=CARTESIAN_POINT('Ctrl Pts',(81.7880655186073,-25.1046109404864,-8.88728238661618));
#11070=CARTESIAN_POINT('Ctrl Pts',(80.9584342768961,-23.7501147475331,-8.96325753689542));
#11071=CARTESIAN_POINT('Ctrl Pts',(80.9419425486894,-23.0352763837504,-9.0021883145108));
#11072=CARTESIAN_POINT('Ctrl Pts',(80.9420825813087,-23.0006320364948,-9.00407471946233));
#11073=CARTESIAN_POINT('Ctrl Pts',(80.9447263139995,-23.0018413368225,-8.24592528053768));
#11074=CARTESIAN_POINT('Ctrl Pts',(80.9497075994821,-22.4621139243731,-8.27521534629936));
#11075=CARTESIAN_POINT('Ctrl Pts',(81.4440784881194,-21.2316953680273,-8.3415497847249));
#11076=CARTESIAN_POINT('Ctrl Pts',(83.5192142592352,-20.6275350489011,-8.44492859581431));
#11077=CARTESIAN_POINT('Ctrl Pts',(85.2747978773029,-22.1494307757635,-8.55606171380584));
#11078=CARTESIAN_POINT('Ctrl Pts',(84.9483969412313,-24.4498009326555,-8.66719483179743));
#11079=CARTESIAN_POINT('Ctrl Pts',(82.8387464372207,-25.4232562134105,-8.77832794978897));
#11080=CARTESIAN_POINT('Ctrl Pts',(81.1984096379769,-24.382902257458,-8.87123809936907));
#11081=CARTESIAN_POINT('Ctrl Pts',(80.9487183110755,-23.3483811293246,-8.9271038762853));
#11082=CARTESIAN_POINT('Ctrl Pts',(80.9485808123477,-22.9999091152425,-8.94592528053768));
#11083=CARTESIAN_POINT('Origin',(83.,-23.,-4.45407471946233));
#11084=CARTESIAN_POINT('',(80.9425252865322,-22.9989407173183,-7.54592528053768));
#11085=CARTESIAN_POINT('',(80.948463949354,-23.0005177854378,-7.60407471946232));
#11086=CARTESIAN_POINT('',(80.94525,-22.9999999999999,-4.45407471946233));
#11087=CARTESIAN_POINT('Ctrl Pts',(80.948463949354,-23.0005177854378,-7.60407471946232));
#11088=CARTESIAN_POINT('Ctrl Pts',(80.949309331527,-22.6256901029336,-7.62432250921123));
#11089=CARTESIAN_POINT('Ctrl Pts',(81.2270645439503,-21.5639294398427,-7.68161467162399));
#11090=CARTESIAN_POINT('Ctrl Pts',(82.9319188416964,-20.5723391423155,-7.77595120670059));
#11091=CARTESIAN_POINT('Ctrl Pts',(85.0026323255168,-21.6260872678191,-7.88708432469216));
#11092=CARTESIAN_POINT('Ctrl Pts',(85.2404578851386,-23.9372944445138,-7.99821744268371));
#11093=CARTESIAN_POINT('Ctrl Pts',(83.4277282032368,-25.3906528329675,-8.10935056067527));
#11094=CARTESIAN_POINT('Ctrl Pts',(81.4056137883196,-24.716681927527,-8.21130298626814));
#11095=CARTESIAN_POINT('Ctrl Pts',(80.950180049126,-23.512075832246,-8.27621103919716));
#11096=CARTESIAN_POINT('Ctrl Pts',(80.9455228522428,-22.9981228933243,-8.30407471946232));
#11097=CARTESIAN_POINT('Ctrl Pts',(80.9425252865322,-22.9989407173183,-7.54592528053768));
#11098=CARTESIAN_POINT('Ctrl Pts',(80.9421428889425,-22.9380656487517,-7.54923807098573));
#11099=CARTESIAN_POINT('Ctrl Pts',(80.9722034692092,-22.1968547417379,-7.58959523409763));
#11100=CARTESIAN_POINT('Ctrl Pts',(81.8697768417376,-20.8504028018083,-7.66699676987338));
#11101=CARTESIAN_POINT('Ctrl Pts',(84.192936911971,-20.8845626742973,-7.77812988786495));
#11102=CARTESIAN_POINT('Ctrl Pts',(85.4242743751978,-22.854854309961,-7.8892630058565));
#11103=CARTESIAN_POINT('Ctrl Pts',(84.4368204072615,-24.9579888637226,-8.00039612384806));
#11104=CARTESIAN_POINT('Ctrl Pts',(82.1343319022801,-25.2690950090472,-8.11152924183961));
#11105=CARTESIAN_POINT('Ctrl Pts',(81.0221614548658,-23.9687902906062,-8.1933722940695));
#11106=CARTESIAN_POINT('Ctrl Pts',(80.9434075591455,-23.1447297834958,-8.23817097363551));
#11107=CARTESIAN_POINT('Ctrl Pts',(80.9447263139995,-23.0018413368225,-8.24592528053768));
#11108=CARTESIAN_POINT('Origin',(83.,-23.,-4.45407471946233));
#11109=CARTESIAN_POINT('',(80.9479085610311,-22.9988355136393,-6.84592528053768));
#11110=CARTESIAN_POINT('',(80.9436249062149,-23.0016062085623,-6.90407471946232));
#11111=CARTESIAN_POINT('',(80.94525,-22.9999999999999,-4.45407471946233));
#11112=CARTESIAN_POINT('Ctrl Pts',(80.9436249062148,-23.0016062085623,-6.90407471946232));
#11113=CARTESIAN_POINT('Ctrl Pts',(80.9485746682535,-22.4253659245422,-6.93538960656144));
#11114=CARTESIAN_POINT('Ctrl Pts',(81.5015294086587,-21.1591279528445,-7.00374886632441));
#11115=CARTESIAN_POINT('Ctrl Pts',(83.6477355304943,-20.659358138271,-7.10915249875124));
#11116=CARTESIAN_POINT('Ctrl Pts',(85.3177707839745,-22.2746643391349,-7.2202856167428));
#11117=CARTESIAN_POINT('Ctrl Pts',(84.8664911752114,-24.5538289281854,-7.33141873473436));
#11118=CARTESIAN_POINT('Ctrl Pts',(82.7069252853353,-25.4108667989543,-7.44255185272592));
#11119=CARTESIAN_POINT('Ctrl Pts',(81.1601824003909,-24.3072526384942,-7.53343718096857));
#11120=CARTESIAN_POINT('Ctrl Pts',(80.9477626613646,-23.3114566249889,-7.58727813654737));
#11121=CARTESIAN_POINT('Ctrl Pts',(80.948463949354,-23.0005177854378,-7.60407471946232));
#11122=CARTESIAN_POINT('Ctrl Pts',(80.9479085610311,-22.9988355136393,-6.84592528053768));
#11123=CARTESIAN_POINT('Ctrl Pts',(80.9465285725618,-22.7328123585093,-6.86030516833594));
#11124=CARTESIAN_POINT('Ctrl Pts',(81.118188380378,-21.7831881263893,-6.91172942879806));
#11125=CARTESIAN_POINT('Ctrl Pts',(82.550772583103,-20.6133039463769,-7.00019806192403));
#11126=CARTESIAN_POINT('Ctrl Pts',(84.7614902208339,-21.3280765684321,-7.11133117991559));
#11127=CARTESIAN_POINT('Ctrl Pts',(85.3600357932379,-23.5730756808161,-7.22246429790715));
#11128=CARTESIAN_POINT('Ctrl Pts',(83.7985771412431,-25.2935651717014,-7.33359741589871));
#11129=CARTESIAN_POINT('Ctrl Pts',(81.5745655362259,-24.9261854356127,-7.44141774344221));
#11130=CARTESIAN_POINT('Ctrl Pts',(80.9464189453495,-23.6187844449696,-7.51219369832188));
#11131=CARTESIAN_POINT('Ctrl Pts',(80.9425252865322,-22.9989407173183,-7.54592528053768));
#11132=CARTESIAN_POINT('Origin',(83.,-23.,-4.45407471946233));
#11133=CARTESIAN_POINT('',(80.9473274916068,-23.0023188026375,-6.14592528053767));
#11134=CARTESIAN_POINT('',(80.9434278273328,-22.9985036630511,-6.20407471946232));
#11135=CARTESIAN_POINT('',(80.94525,-22.9999999999999,-4.45407471946233));
#11136=CARTESIAN_POINT('',(82.4698297828114,-24.9851743256717,-6.));
#11137=CARTESIAN_POINT('Ctrl Pts',(82.4698297828114,-24.9851743256717,-6.));
#11138=CARTESIAN_POINT('Ctrl Pts',(81.8097404375819,-24.8088876857537,-6.03704437266385));
#11139=CARTESIAN_POINT('Ctrl Pts',(81.0750710560616,-24.1127868016837,-6.08568613284308));
#11140=CARTESIAN_POINT('Ctrl Pts',(80.9457104966695,-23.2165873425108,-6.1343278930223));
#11141=CARTESIAN_POINT('Ctrl Pts',(80.9473274916068,-23.0023188026375,-6.14592528053767));
#11142=CARTESIAN_POINT('',(83.5313111338805,-24.9887317157019,-5.99999999999999));
#11143=CARTESIAN_POINT('Origin',(83.,-23.,-6.));
#11144=CARTESIAN_POINT('Ctrl Pts',(83.5313118283826,-24.9887338811667,-6.));
#11145=CARTESIAN_POINT('Ctrl Pts',(82.8867914735066,-25.1600294862445,-6.03631814560907));
#11146=CARTESIAN_POINT('Ctrl Pts',(81.5070305341199,-24.840734884675,-6.10434305209651));
#11147=CARTESIAN_POINT('Ctrl Pts',(80.94828062884,-23.581675994672,-6.17236795858395));
#11148=CARTESIAN_POINT('Ctrl Pts',(80.9434278273328,-22.9985036630511,-6.20407471946232));
#11149=CARTESIAN_POINT('Origin',(83.,-23.,-17.));
#11150=CARTESIAN_POINT('Ctrl Pts',(82.2300979593296,-24.4774325188554,-17.));
#11151=CARTESIAN_POINT('Ctrl Pts',(82.2818390981198,-24.5125050767042,-17.));
#11152=CARTESIAN_POINT('Ctrl Pts',(82.3355567268774,-24.5443225394793,-17.));
#11153=CARTESIAN_POINT('Ctrl Pts',(82.3909195452282,-24.5729489534796,-17.));
#11154=CARTESIAN_POINT('Ctrl Pts',(82.4260295600056,-24.5911032644146,-17.));
#11155=CARTESIAN_POINT('Ctrl Pts',(82.4618021381845,-24.607973536627,-17.));
#11156=CARTESIAN_POINT('Ctrl Pts',(82.4981603817539,-24.6235688924305,-17.));
#11157=CARTESIAN_POINT('Ctrl Pts',(82.522943255033,-24.6341991564002,-17.));
#11158=CARTESIAN_POINT('Ctrl Pts',(82.5479983580097,-24.6442369519448,-17.));
#11159=CARTESIAN_POINT('Ctrl Pts',(82.5733025786055,-24.6536835842467,-17.));
#11160=CARTESIAN_POINT('Ctrl Pts',(82.5867931904283,-24.6587199317973,-17.));
#11161=CARTESIAN_POINT('Ctrl Pts',(82.6003545666375,-24.6635880767879,-17.));
#11162=CARTESIAN_POINT('Ctrl Pts',(82.6139694944138,-24.6682836926456,-17.));
#11163=CARTESIAN_POINT('Ctrl Pts',(82.6763337730807,-24.6897923411434,-17.));
#11164=CARTESIAN_POINT('Ctrl Pts',(82.7398893644175,-24.7077113174207,-17.));
#11165=CARTESIAN_POINT('Ctrl Pts',(82.8042863740348,-24.7220871703776,-17.));
#11166=CARTESIAN_POINT('Ctrl Pts',(82.8507390234662,-24.7324571621155,-17.));
#11167=CARTESIAN_POINT('Ctrl Pts',(82.8976303986295,-24.7409826885964,-17.));
#11168=CARTESIAN_POINT('Ctrl Pts',(82.9448382797826,-24.7476671912803,-17.));
#11169=CARTESIAN_POINT('Ctrl Pts',(82.9577357961264,-24.7494934431795,-17.));
#11170=CARTESIAN_POINT('Ctrl Pts',(82.9706569702704,-24.7511822070801,-17.));
#11171=CARTESIAN_POINT('Ctrl Pts',(82.983599376443,-24.7527333925106,-17.));
#11172=CARTESIAN_POINT('Ctrl Pts',(82.9969328091843,-24.7543314436251,-17.));
#11173=CARTESIAN_POINT('Ctrl Pts',(83.0102808606987,-24.7557824881839,-17.));
#11174=CARTESIAN_POINT('Ctrl Pts',(83.0236352576791,-24.7570864480777,-17.));
#11175=CARTESIAN_POINT('Ctrl Pts',(83.0911664152792,-24.763680375248,-17.));
#11176=CARTESIAN_POINT('Ctrl Pts',(83.1589012578161,-24.7665219197639,-17.));
#11177=CARTESIAN_POINT('Ctrl Pts',(83.2264851078505,-24.7656590371379,-17.));
#11178=CARTESIAN_POINT('Ctrl Pts',(83.2950476435056,-24.7647836590591,-17.));
#11179=CARTESIAN_POINT('Ctrl Pts',(83.3634557918544,-24.760096122702,-17.));
#11180=CARTESIAN_POINT('Ctrl Pts',(83.4313607347552,-24.7515982025416,-17.));
#11181=CARTESIAN_POINT('Ctrl Pts',(83.4734287914636,-24.7463336227933,-17.));
#11182=CARTESIAN_POINT('Ctrl Pts',(83.5153040865525,-24.73960565681,-17.));
#11183=CARTESIAN_POINT('Ctrl Pts',(83.5569050591773,-24.7314047821333,-17.));
#11184=CARTESIAN_POINT('Ctrl Pts',(83.5909684950016,-24.7246897956648,-17.));
#11185=CARTESIAN_POINT('Ctrl Pts',(83.6248480498378,-24.7169871539346,-17.));
#11186=CARTESIAN_POINT('Ctrl Pts',(83.6584986050691,-24.7082876471674,-17.));
#11187=CARTESIAN_POINT('Ctrl Pts',(83.6722821884436,-24.7047242475141,-17.));
#11188=CARTESIAN_POINT('Ctrl Pts',(83.6860298150871,-24.7009927099034,-17.));
#11189=CARTESIAN_POINT('Ctrl Pts',(83.6997151251742,-24.6970992429687,-17.));
#11190=CARTESIAN_POINT('Ctrl Pts',(83.7675104829974,-24.6778114824186,-17.));
#11191=CARTESIAN_POINT('Ctrl Pts',(83.8338962305779,-24.6545245448285,-17.));
#11192=CARTESIAN_POINT('Ctrl Pts',(83.8985096339753,-24.6272571466379,-17.));
#11193=CARTESIAN_POINT('Ctrl Pts',(83.9056765518862,-24.6242326471657,-17.));
#11194=CARTESIAN_POINT('Ctrl Pts',(83.9128216721735,-24.6211591229274,-17.));
#11195=CARTESIAN_POINT('Ctrl Pts',(83.9199445039688,-24.6180365600954,-17.));
#11196=CARTESIAN_POINT('Ctrl Pts',(83.9816971879894,-24.5909649344499,-17.));
#11197=CARTESIAN_POINT('Ctrl Pts',(84.0417754148873,-24.5602117258275,-17.));
#11198=CARTESIAN_POINT('Ctrl Pts',(84.1000372506631,-24.5260871320529,-17.));
#11199=CARTESIAN_POINT('Ctrl Pts',(84.1627131029041,-24.4893772006076,-17.));
#11200=CARTESIAN_POINT('Ctrl Pts',(84.2232879180125,-24.4487656795587,-17.));
#11201=CARTESIAN_POINT('Ctrl Pts',(84.2815651125216,-24.4045776673306,-17.));
#11202=CARTESIAN_POINT('Ctrl Pts',(84.2920907285267,-24.3965967400973,-17.));
#11203=CARTESIAN_POINT('Ctrl Pts',(84.3025413203083,-24.3884989956002,-17.));
#11204=CARTESIAN_POINT('Ctrl Pts',(84.3129156246037,-24.3802861603243,-17.));
#11205=CARTESIAN_POINT('Ctrl Pts',(84.3220913046107,-24.3730222179629,-17.));
#11206=CARTESIAN_POINT('Ctrl Pts',(84.3312003064953,-24.3656737636397,-17.));
#11207=CARTESIAN_POINT('Ctrl Pts',(84.3402399813965,-24.3582440922858,-17.));
#11208=CARTESIAN_POINT('Ctrl Pts',(84.395143202012,-24.3131193627022,-17.));
#11209=CARTESIAN_POINT('Ctrl Pts',(84.447514283769,-24.2649838963252,-17.));
#11210=CARTESIAN_POINT('Ctrl Pts',(84.4972032115259,-24.2141876925674,-17.));
#11211=CARTESIAN_POINT('Ctrl Pts',(84.547939867273,-24.1623204130814,-17.));
#11212=CARTESIAN_POINT('Ctrl Pts',(84.5958808308285,-24.107678464869,-17.));
#11213=CARTESIAN_POINT('Ctrl Pts',(84.6408461878852,-24.050583168076,-17.));
#11214=CARTESIAN_POINT('Ctrl Pts',(84.6860842877404,-23.9931415528714,-17.));
#11215=CARTESIAN_POINT('Ctrl Pts',(84.7283113614493,-23.9332160077481,-17.));
#11216=CARTESIAN_POINT('Ctrl Pts',(84.7673122483243,-23.8710921936606,-17.));
#11217=CARTESIAN_POINT('Ctrl Pts',(84.7769393443201,-23.8557573648973,-17.));
#11218=CARTESIAN_POINT('Ctrl Pts',(84.7863696800929,-23.840288425334,-17.));
#11219=CARTESIAN_POINT('Ctrl Pts',(84.7955996348862,-23.8246893660786,-17.));
#11220=CARTESIAN_POINT('Ctrl Pts',(84.8028491435325,-23.8124373542888,-17.));
#11221=CARTESIAN_POINT('Ctrl Pts',(84.8099757745391,-23.8001035206571,-17.));
#11222=CARTESIAN_POINT('Ctrl Pts',(84.8169673085382,-23.7877088770335,-17.));
#11223=CARTESIAN_POINT('Ctrl Pts',(84.8539824412826,-23.7220881736068,-17.));
#11224=CARTESIAN_POINT('Ctrl Pts',(84.8872834934608,-23.6546505166455,-17.));
#11225=CARTESIAN_POINT('Ctrl Pts',(84.9166897351286,-23.5857422245182,-17.));
#11226=CARTESIAN_POINT('Ctrl Pts',(84.9461280445966,-23.51675878721,-17.));
#11227=CARTESIAN_POINT('Ctrl Pts',(84.9716638092362,-23.4463006762683,-17.));
#11228=CARTESIAN_POINT('Ctrl Pts',(84.9930799698159,-23.3746776330315,-17.));
#11229=CARTESIAN_POINT('Ctrl Pts',(85.0140089050527,-23.3046840397455,-17.));
#11230=CARTESIAN_POINT('Ctrl Pts',(85.0310041061321,-23.233577039206,-17.));
#11231=CARTESIAN_POINT('Ctrl Pts',(85.043819389628,-23.1616224987288,-17.));
#11232=CARTESIAN_POINT('Ctrl Pts',(85.0465681982955,-23.1461886408205,-17.));
#11233=CARTESIAN_POINT('Ctrl Pts',(85.0491245173261,-23.1307157299229,-17.));
#11234=CARTESIAN_POINT('Ctrl Pts',(85.0514856095148,-23.115206305485,-17.));
#11235=CARTESIAN_POINT('Ctrl Pts',(85.0534987950829,-23.1019821926799,-17.));
#11236=CARTESIAN_POINT('Ctrl Pts',(85.0553700460339,-23.0887315335367,-17.));
#11237=CARTESIAN_POINT('Ctrl Pts',(85.0571001899048,-23.0754560264203,-17.));
#11238=CARTESIAN_POINT('Ctrl Pts',(84.8174278887595,-22.0413794120407,-17.));
#11239=CARTESIAN_POINT('Ctrl Pts',(84.7765814196328,-21.9788996623134,-17.));
#11240=CARTESIAN_POINT('Ctrl Pts',(84.7321382587602,-21.9189706353617,-17.));
#11241=CARTESIAN_POINT('Ctrl Pts',(84.6844272556429,-21.8617421036743,-17.));
#11242=CARTESIAN_POINT('Ctrl Pts',(84.6379676814808,-21.8060146396012,-17.));
#11243=CARTESIAN_POINT('Ctrl Pts',(84.5884084476132,-21.7528476571992,-17.));
#11244=CARTESIAN_POINT('Ctrl Pts',(84.53602713658,-21.7024171202736,-17.));
#11245=CARTESIAN_POINT('Ctrl Pts',(84.5243354623359,-21.6911608649784,-17.));
#11246=CARTESIAN_POINT('Ctrl Pts',(84.5125015270917,-21.6800396402157,-17.));
#11247=CARTESIAN_POINT('Ctrl Pts',(84.5005334026731,-21.6690603431566,-17.));
#11248=CARTESIAN_POINT('Ctrl Pts',(84.4456122010496,-21.618676827212,-17.));
#11249=CARTESIAN_POINT('Ctrl Pts',(84.3879772657735,-21.5713777924382,-17.));
#11250=CARTESIAN_POINT('Ctrl Pts',(84.3279447447431,-21.5273357256383,-17.));
#11251=CARTESIAN_POINT('Ctrl Pts',(84.2858002354275,-21.4964169625633,-17.));
#11252=CARTESIAN_POINT('Ctrl Pts',(84.2424734095645,-21.4671042688097,-17.));
#11253=CARTESIAN_POINT('Ctrl Pts',(84.1980683256475,-21.4394717254802,-17.));
#11254=CARTESIAN_POINT('Ctrl Pts',(84.1811929239341,-21.4289704443675,-17.));
#11255=CARTESIAN_POINT('Ctrl Pts',(84.1641617661438,-21.4187119484129,-17.));
#11256=CARTESIAN_POINT('Ctrl Pts',(84.1469804883186,-21.4087007908574,-17.));
#11257=CARTESIAN_POINT('Ctrl Pts',(84.1305957095552,-21.3991537360118,-17.));
#11258=CARTESIAN_POINT('Ctrl Pts',(84.1140690908491,-21.3898288825432,-17.));
#11259=CARTESIAN_POINT('Ctrl Pts',(84.0974351122763,-21.3807460873294,-17.));
#11260=CARTESIAN_POINT('Ctrl Pts',(84.033718117405,-21.3459541454306,-17.));
#11261=CARTESIAN_POINT('Ctrl Pts',(83.9683621660843,-21.314669355336,-17.));
#11262=CARTESIAN_POINT('Ctrl Pts',(83.9016589606957,-21.287053352088,-17.));
#11263=CARTESIAN_POINT('Ctrl Pts',(83.8363880887512,-21.2600303537011,-17.));
#11264=CARTESIAN_POINT('Ctrl Pts',(83.7698262768392,-21.2365201185219,-17.));
#11265=CARTESIAN_POINT('Ctrl Pts',(83.702238233304,-21.2167223499385,-17.));
#11266=CARTESIAN_POINT('Ctrl Pts',(83.6361325166137,-21.1973587818779,-17.));
#11267=CARTESIAN_POINT('Ctrl Pts',(83.5690443270263,-21.1815465129351,-17.));
#11268=CARTESIAN_POINT('Ctrl Pts',(83.5012252689848,-21.1695209782649,-17.));
#11269=CARTESIAN_POINT('Ctrl Pts',(83.4791651243258,-21.1656093191813,-17.));
#11270=CARTESIAN_POINT('Ctrl Pts',(83.457027727715,-21.1620987189897,-17.));
#11271=CARTESIAN_POINT('Ctrl Pts',(83.4348220326898,-21.1589984540086,-17.));
#11272=CARTESIAN_POINT('Ctrl Pts',(83.4223375091993,-21.1572554177768,-17.));
#11273=CARTESIAN_POINT('Ctrl Pts',(83.4098301119865,-21.1556420422429,-17.));
#11274=CARTESIAN_POINT('Ctrl Pts',(83.3973191364083,-21.1541618553483,-17.));
#11275=CARTESIAN_POINT('Ctrl Pts',(83.3294884653499,-21.1461367361461,-17.));
#11276=CARTESIAN_POINT('Ctrl Pts',(83.2614342665035,-21.1420048354048,-17.));
#11277=CARTESIAN_POINT('Ctrl Pts',(83.1934022649708,-21.1419441932168,-17.));
#11278=CARTESIAN_POINT('Ctrl Pts',(83.1836053465211,-21.1419354604652,-17.));
#11279=CARTESIAN_POINT('Ctrl Pts',(83.173808894589,-21.1420112428234,-17.));
#11280=CARTESIAN_POINT('Ctrl Pts',(83.1640136523952,-21.142172161946,-17.));
#11281=CARTESIAN_POINT('Ctrl Pts',(83.0946494144972,-21.1433116980679,-17.));
#11282=CARTESIAN_POINT('Ctrl Pts',(83.0253443835876,-21.1487165123659,-17.));
#11283=CARTESIAN_POINT('Ctrl Pts',(82.9564235651142,-21.1582133774548,-17.));
#11284=CARTESIAN_POINT('Ctrl Pts',(82.8921283089566,-21.1670728684926,-17.));
#11285=CARTESIAN_POINT('Ctrl Pts',(82.828166910253,-21.17949449625,-17.));
#11286=CARTESIAN_POINT('Ctrl Pts',(82.7648237414818,-21.1953720660214,-17.));
#11287=CARTESIAN_POINT('Ctrl Pts',(82.7509590903951,-21.1988473731343,-17.));
#11288=CARTESIAN_POINT('Ctrl Pts',(82.7371241565956,-21.2024883622745,-17.));
#11289=CARTESIAN_POINT('Ctrl Pts',(82.7233220999365,-21.2062940979554,-17.));
#11290=CARTESIAN_POINT('Ctrl Pts',(82.7122616849786,-21.209343861979,-17.));
#11291=CARTESIAN_POINT('Ctrl Pts',(82.7012229288043,-21.2124993619089,-17.));
#11292=CARTESIAN_POINT('Ctrl Pts',(82.6902205125981,-21.2157559907085,-17.));
#11293=CARTESIAN_POINT('Ctrl Pts',(82.6246583197173,-21.2351618849685,-17.));
#11294=CARTESIAN_POINT('Ctrl Pts',(82.5602625039766,-21.2581877772728,-17.));
#11295=CARTESIAN_POINT('Ctrl Pts',(82.4973355231435,-21.2846516488133,-17.));
#11296=CARTESIAN_POINT('Ctrl Pts',(82.4346998948261,-21.3109929923786,-17.));
#11297=CARTESIAN_POINT('Ctrl Pts',(82.3735186391274,-21.3407412554097,-17.));
#11298=CARTESIAN_POINT('Ctrl Pts',(82.3141198251038,-21.3737584862197,-17.));
#11299=CARTESIAN_POINT('Ctrl Pts',(82.2559937181132,-21.406068274254,-17.));
#11300=CARTESIAN_POINT('Ctrl Pts',(82.1995738158673,-21.4415091484104,-17.));
#11301=CARTESIAN_POINT('Ctrl Pts',(82.1452074852454,-21.479981235296,-17.));
#11302=CARTESIAN_POINT('Ctrl Pts',(82.1337109572647,-21.4881167010943,-17.));
#11303=CARTESIAN_POINT('Ctrl Pts',(82.1223064242023,-21.4963877994906,-17.));
#11304=CARTESIAN_POINT('Ctrl Pts',(82.1109974490861,-21.5047937147772,-17.));
#11305=CARTESIAN_POINT('Ctrl Pts',(82.1003663825044,-21.5126957434026,-17.));
#11306=CARTESIAN_POINT('Ctrl Pts',(82.0898185292626,-21.5207180219682,-17.));
#11307=CARTESIAN_POINT('Ctrl Pts',(82.0793734282098,-21.5288466119773,-17.));
#11308=CARTESIAN_POINT('Ctrl Pts',(82.0278060377264,-21.5689774037198,-17.));
#11309=CARTESIAN_POINT('Ctrl Pts',(81.9786452211898,-21.6117656835976,-17.));
#11310=CARTESIAN_POINT('Ctrl Pts',(81.9321820573122,-21.6570794404074,-17.));
#11311=CARTESIAN_POINT('Ctrl Pts',(81.8866025322933,-21.7015314178417,-17.));
#11312=CARTESIAN_POINT('Ctrl Pts',(81.8436184450026,-21.7484143885941,-17.));
#11313=CARTESIAN_POINT('Ctrl Pts',(81.8035470978193,-21.7976294922613,-17.));
#11314=CARTESIAN_POINT('Ctrl Pts',(81.7647768670758,-21.8452465817621,-17.));
#11315=CARTESIAN_POINT('Ctrl Pts',(81.7287329529628,-21.8950473870754,-17.));
#11316=CARTESIAN_POINT('Ctrl Pts',(81.6957494077667,-21.9469577312498,-17.));
#11317=CARTESIAN_POINT('Ctrl Pts',(81.6902971226995,-21.9555386764662,-17.));
#11318=CARTESIAN_POINT('Ctrl Pts',(81.6849285755936,-21.9641772894425,-17.));
#11319=CARTESIAN_POINT('Ctrl Pts',(81.6796454131484,-21.9728732610623,-17.));
#11320=CARTESIAN_POINT('Ctrl Pts',(81.6739898323046,-21.9821822253468,-17.));
#11321=CARTESIAN_POINT('Ctrl Pts',(81.6684320988345,-21.991556920899,-17.));
#11322=CARTESIAN_POINT('Ctrl Pts',(81.6629726161762,-22.000995687242,-17.));
#11323=CARTESIAN_POINT('Origin',(83.,-23.,-4.45407471946233));
#11324=CARTESIAN_POINT('Ctrl Pts',(80.9434278273328,-22.9985036630511,-6.20407471946232));
#11325=CARTESIAN_POINT('Ctrl Pts',(80.9426108920862,-22.9003306733166,-6.20941233124781));
#11326=CARTESIAN_POINT('Ctrl Pts',(80.9936360510926,-22.1216407869118,-6.25179431569714));
#11327=CARTESIAN_POINT('Ctrl Pts',(81.9885905792076,-20.7918186937154,-6.33122067281033));
#11328=CARTESIAN_POINT('Ctrl Pts',(84.3064560817636,-20.952810958716,-6.44235379080188));
#11329=CARTESIAN_POINT('Ctrl Pts',(85.4285782577618,-22.9871398469054,-6.55348690879345));
#11330=CARTESIAN_POINT('Ctrl Pts',(84.3279817091015,-25.0334050191953,-6.664620026785));
#11331=CARTESIAN_POINT('Ctrl Pts',(82.0119581717988,-25.218534557138,-6.77575314477657));
#11332=CARTESIAN_POINT('Ctrl Pts',(80.9980258697689,-23.8931863027124,-6.855571375669));
#11333=CARTESIAN_POINT('Ctrl Pts',(80.9427192797612,-23.107037225403,-6.89834523389759));
#11334=CARTESIAN_POINT('Ctrl Pts',(80.9436249062148,-23.0016062085623,-6.90407471946232));
#11335=CARTESIAN_POINT('Ctrl Pts',(80.9473274916068,-23.0023188026375,-6.14592528053767));
#11336=CARTESIAN_POINT('Ctrl Pts',(80.9508755015445,-22.5321708193339,-6.17137226568616));
#11337=CARTESIAN_POINT('Ctrl Pts',(81.3433671183963,-21.3705995282974,-6.23386362349849));
#11338=CARTESIAN_POINT('Ctrl Pts',(83.2718171975381,-20.587166548819,-6.33339935397468));
#11339=CARTESIAN_POINT('Ctrl Pts',(85.1745320976991,-21.9187032679059,-6.44453247196624));
#11340=CARTESIAN_POINT('Ctrl Pts',(85.0878555654783,-24.2409162559102,-6.55566558995779));
#11341=CARTESIAN_POINT('Ctrl Pts',(83.0898774551597,-25.4268774336938,-6.66679870794935));
#11342=CARTESIAN_POINT('Ctrl Pts',(81.2789895846428,-24.5258398827689,-6.76355193814265));
#11343=CARTESIAN_POINT('Ctrl Pts',(80.950083593842,-23.4181209669006,-6.82326079567209));
#11344=CARTESIAN_POINT('Ctrl Pts',(80.9479085610311,-22.9988355136393,-6.84592528053768));
#11345=CARTESIAN_POINT('Ctrl Pts',(84.2690708798524,-21.9206413469515,-6.));
#11346=CARTESIAN_POINT('Ctrl Pts',(84.627967898288,-22.3426194852432,-6.03704437266385));
#11347=CARTESIAN_POINT('Ctrl Pts',(84.8852397370454,-23.5657433557833,-6.11113311799156));
#11348=CARTESIAN_POINT('Ctrl Pts',(83.5452626210686,-24.8933533980037,-6.22226623598312));
#11349=CARTESIAN_POINT('Ctrl Pts',(81.7059923092724,-24.4836988369728,-6.33339935397468));
#11350=CARTESIAN_POINT('Ctrl Pts',(81.0511940946918,-22.718246934168,-6.44453247196624));
#11351=CARTESIAN_POINT('Ctrl Pts',(82.1799449592213,-21.2095972472222,-6.55566558995779));
#11352=CARTESIAN_POINT('Ctrl Pts',(84.059280122749,-21.3401304573407,-6.66679870794935));
#11353=CARTESIAN_POINT('Ctrl Pts',(84.9691015342163,-22.9895729334198,-6.77793182594091));
#11354=CARTESIAN_POINT('Ctrl Pts',(84.0767331925359,-24.6486933991869,-6.88906494393248));
#11355=CARTESIAN_POINT('Ctrl Pts',(82.1988915022347,-24.7987972124064,-7.00019806192403));
#11356=CARTESIAN_POINT('Ctrl Pts',(81.0542582228978,-23.302604896914,-7.11133117991558));
#11357=CARTESIAN_POINT('Ctrl Pts',(81.6904432068723,-21.5294396795688,-7.22246429790715));
#11358=CARTESIAN_POINT('Ctrl Pts',(83.5251867106965,-21.1021976680177,-7.33359741589871));
#11359=CARTESIAN_POINT('Ctrl Pts',(84.8792583653007,-22.4118947750328,-7.44473053389027));
#11360=CARTESIAN_POINT('Ctrl Pts',(84.5133589477561,-24.2598510740269,-7.55586365188182));
#11361=CARTESIAN_POINT('Ctrl Pts',(82.7623737804448,-24.9547410084233,-7.66699676987339));
#11362=CARTESIAN_POINT('Ctrl Pts',(81.2288735200345,-23.8605755728289,-7.77812988786494));
#11363=CARTESIAN_POINT('Ctrl Pts',(81.3163779059484,-21.9787772308784,-7.8892630058565));
#11364=CARTESIAN_POINT('Ctrl Pts',(82.9447995085857,-21.0316422976506,-8.00039612384807));
#11365=CARTESIAN_POINT('Ctrl Pts',(84.6237427688579,-21.8860257394752,-8.11152924183962));
#11366=CARTESIAN_POINT('Ctrl Pts',(84.8165727395747,-23.7599623042025,-8.22266235983119));
#11367=CARTESIAN_POINT('Ctrl Pts',(83.3468038382248,-24.9383514392134,-8.33379547782273));
#11368=CARTESIAN_POINT('Ctrl Pts',(81.5596264146683,-24.3426850528549,-8.44492859581431));
#11369=CARTESIAN_POINT('Ctrl Pts',(81.0907355886569,-22.5181404542583,-8.55606171380585));
#11370=CARTESIAN_POINT('Ctrl Pts',(82.3692786999733,-21.134612679886,-8.66719483179742));
#11371=CARTESIAN_POINT('Ctrl Pts',(84.2250827699467,-21.458360800731,-8.77832794978898));
#11372=CARTESIAN_POINT('Ctrl Pts',(84.9596428701148,-23.1930777956164,-8.88946106778053));
#11373=CARTESIAN_POINT('Ctrl Pts',(83.9006606847433,-24.7510823922139,-9.0005941857721));
#11374=CARTESIAN_POINT('Ctrl Pts',(82.017358391045,-24.7064274616622,-9.11172730376365));
#11375=CARTESIAN_POINT('Ctrl Pts',(81.0334083742546,-23.0999829537985,-9.22286042175522));
#11376=CARTESIAN_POINT('Ctrl Pts',(81.8493604176406,-21.4020301113619,-9.33399353974677));
#11377=CARTESIAN_POINT('Ctrl Pts',(83.7184230955337,-21.1666022064717,-9.44512665773833));
#11378=CARTESIAN_POINT('Ctrl Pts',(84.9299566795373,-22.6091721240612,-9.5562597757299));
#11379=CARTESIAN_POINT('Ctrl Pts',(84.3751179480734,-24.4094430965408,-9.66739289372144));
#11380=CARTESIAN_POINT('Ctrl Pts',(82.5617171464179,-24.9197362719288,-9.77852601171301));
#11381=CARTESIAN_POINT('Ctrl Pts',(81.1494500630057,-23.6730112511631,-9.88965912970457));
#11382=CARTESIAN_POINT('Ctrl Pts',(81.4308791188664,-21.8103198438688,-10.0007922476961));
#11383=CARTESIAN_POINT('Ctrl Pts',(83.1484293651367,-21.0364705408201,-10.1119253656877));
#11384=CARTESIAN_POINT('Ctrl Pts',(84.7301312143109,-22.0597206825795,-10.2230584836792));
#11385=CARTESIAN_POINT('Ctrl Pts',(84.7283488788469,-23.9435514646753,-10.3341916016708));
#11386=CARTESIAN_POINT('Ctrl Pts',(83.144713622313,-24.9638068084766,-10.4453247196624));
#11387=CARTESIAN_POINT('Ctrl Pts',(81.4286307627658,-24.1867088664773,-10.5564578376539));
#11388=CARTESIAN_POINT('Ctrl Pts',(81.1507268776256,-22.3234882614722,-10.6675909556455));
#11389=CARTESIAN_POINT('Ctrl Pts',(82.5653505407635,-21.0794378268102,-10.7787240736371));
#11390=CARTESIAN_POINT('Ctrl Pts',(84.3777824966304,-21.5931614856421,-10.8898571916286));
#11391=CARTESIAN_POINT('Ctrl Pts',(84.9292136825907,-23.3944791254386,-11.0009903096202));
#11392=CARTESIAN_POINT('Ctrl Pts',(83.7149525731334,-24.8347539430867,-11.1121234276117));
#11393=CARTESIAN_POINT('Ctrl Pts',(81.8463387284853,-24.5957897368103,-11.2232565456033));
#11394=CARTESIAN_POINT('Ctrl Pts',(81.0336010871927,-22.8962959537331,-11.3343896635948));
#11395=CARTESIAN_POINT('Ctrl Pts',(82.0205891276083,-21.2917161955509,-11.4455227815864));
#11396=CARTESIAN_POINT('Ctrl Pts',(83.9039725476732,-21.2506250125958,-11.556655899578));
#11397=CARTESIAN_POINT('Ctrl Pts',(84.9600047120946,-22.8106306728416,-11.6677890175695));
#11398=CARTESIAN_POINT('Ctrl Pts',(84.2221634189736,-24.5439545948068,-11.7789221355611));
#11399=CARTESIAN_POINT('Ctrl Pts',(82.3657500609242,-24.8641905021442,-11.8900552535526));
#11400=CARTESIAN_POINT('Ctrl Pts',(81.0898272109517,-23.478245888096,-12.0011883715442));
#11401=CARTESIAN_POINT('Ctrl Pts',(81.5621696811842,-21.6545918136877,-12.1123214895357));
#11402=CARTESIAN_POINT('Ctrl Pts',(83.3504710516471,-21.0623082661426,-12.2234546075273));
#11403=CARTESIAN_POINT('Ctrl Pts',(84.8180075212363,-22.2434764602272,-12.3345877255189));
#11404=CARTESIAN_POINT('Ctrl Pts',(84.6216319513115,-24.1170447743883,-12.4457208435104));
#11405=CARTESIAN_POINT('Ctrl Pts',(82.9410749927345,-24.9682497445753,-12.556853961502));
#11406=CARTESIAN_POINT('Ctrl Pts',(81.3144485200729,-24.018035078972,-12.6679870794935));
#11407=CARTESIAN_POINT('Ctrl Pts',(81.2305051045002,-22.1360746396232,-12.7791201974851));
#11408=CARTESIAN_POINT('Ctrl Pts',(82.7660730639293,-21.0448126938621,-12.8902533154767));
#11409=CARTESIAN_POINT('Ctrl Pts',(84.5157401625249,-21.7430151261009,-13.0013864334682));
#11410=CARTESIAN_POINT('Ctrl Pts',(84.8781422054261,-23.5916595893747,-13.1125195514598));
#11411=CARTESIAN_POINT('Ctrl Pts',(83.5215945789647,-24.8987939089582,-13.2236526694514));
#11412=CARTESIAN_POINT('Ctrl Pts',(81.687663064072,-24.4680773072633,-13.3347857874429));
#11413=CARTESIAN_POINT('Ctrl Pts',(81.0548339660191,-22.6937185710011,-13.4459189054345));
#11414=CARTESIAN_POINT('Ctrl Pts',(82.2022973832551,-21.1996806536787,-13.557052023426));
#11415=CARTESIAN_POINT('Ctrl Pts',(84.0798496326035,-21.3533658619876,-13.6681851414176));
#11416=CARTESIAN_POINT('Ctrl Pts',(84.9690809957294,-23.0141154442955,-13.7793182594091));
#11417=CARTESIAN_POINT('Ctrl Pts',(84.0561319292834,-24.6619460164019,-13.8904513774007));
#11418=CARTESIAN_POINT('Ctrl Pts',(82.1765693522251,-24.788698180747,-14.0015844953923));
#11419=CARTESIAN_POINT('Ctrl Pts',(81.0506429138938,-23.2783633675832,-14.1127176133838));
#11420=CARTESIAN_POINT('Ctrl Pts',(81.7088448067759,-21.5132594441617,-14.2238507313754));
#11421=CARTESIAN_POINT('Ctrl Pts',(83.5487627517468,-21.1088789949219,-14.3349838493669));
#11422=CARTESIAN_POINT('Ctrl Pts',(84.8864314274729,-22.4353269234458,-14.4461169673585));
#11423=CARTESIAN_POINT('Ctrl Pts',(84.4975638110693,-24.278585876711,-14.55725008535));
#11424=CARTESIAN_POINT('Ctrl Pts',(82.7380668522128,-24.9516327114326,-14.6683832033416));
#11425=CARTESIAN_POINT('Ctrl Pts',(81.2183014178553,-23.838468472195,-14.7795163213332));
#11426=CARTESIAN_POINT('Ctrl Pts',(81.3292166567263,-21.9579048872837,-14.8906494393247));
#11427=CARTESIAN_POINT('Ctrl Pts',(82.969298565022,-21.0311077622519,-15.0017825573163));
#11428=CARTESIAN_POINT('Ctrl Pts',(84.6374796504228,-21.9063183155134,-15.1129156753078));
#11429=CARTESIAN_POINT('Ctrl Pts',(84.8069748784432,-23.7825093784266,-15.2240487932994));
#11430=CARTESIAN_POINT('Ctrl Pts',(83.3226556371789,-24.9425170886116,-15.3351819112909));
#11431=CARTESIAN_POINT('Ctrl Pts',(81.5430291349163,-24.3246566433919,-15.4463150292825));
#11432=CARTESIAN_POINT('Ctrl Pts',(81.0968799579766,-22.4944184181754,-15.5574481472741));
#11433=CARTESIAN_POINT('Ctrl Pts',(82.3925406634323,-21.1269081208074,-15.6685812652656));
#11434=CARTESIAN_POINT('Ctrl Pts',(84.244173032512,-21.4737257047449,-15.7797143832572));
#11435=CARTESIAN_POINT('Ctrl Pts',(84.9570873388809,-23.2174486614387,-15.8908475012488));
#11436=CARTESIAN_POINT('Ctrl Pts',(83.8788021375398,-24.7621559106701,-16.0019806192403));
#11437=CARTESIAN_POINT('Ctrl Pts',(81.9961949431072,-24.6940649912425,-16.1131137372319));
#11438=CARTESIAN_POINT('Ctrl Pts',(81.0323249760943,-23.0755065351483,-16.2242468552234));
#11439=CARTESIAN_POINT('Ctrl Pts',(81.8693180677509,-21.3878267275145,-16.335379973215));
#11440=CARTESIAN_POINT('Ctrl Pts',(83.7412167282557,-21.1757008640235,-16.4465130912065));
#11441=CARTESIAN_POINT('Ctrl Pts',(84.9346030992696,-22.6331865250633,-16.5576462091981));
#11442=CARTESIAN_POINT('Ctrl Pts',(84.3576069929949,-24.4265116682426,-16.6687793271897));
#11443=CARTESIAN_POINT('Ctrl Pts',(82.5375920396697,-24.9140031674198,-16.7799124451812));
#11444=CARTESIAN_POINT('Ctrl Pts',(81.1417560182126,-23.6501903157134,-16.8910455631728));
#11445=CARTESIAN_POINT('Ctrl Pts',(81.4447231066816,-21.7903669148141,-17.0021786811644));
#11446=CARTESIAN_POINT('Ctrl Pts',(83.1751275589987,-21.0395090541329,-17.1133117991559));
#11447=CARTESIAN_POINT('Ctrl Pts',(84.2151340020225,-21.7327675918889,-17.1874005444836));
#11448=CARTESIAN_POINT('Ctrl Pts',(84.4735782273626,-22.2227463683951,-17.2244449171475));
#11449=CARTESIAN_POINT('Ctrl Pts',(84.3677806246588,-21.8366876301902,-5.92518502761751));
#11450=CARTESIAN_POINT('Ctrl Pts',(84.7545930524416,-22.2914876975058,-5.96222940028136));
#11451=CARTESIAN_POINT('Ctrl Pts',(85.0318757810182,-23.6097475033545,-6.03631814560907));
#11452=CARTESIAN_POINT('Ctrl Pts',(83.5876737543099,-25.0406205315519,-6.14745126360063));
#11453=CARTESIAN_POINT('Ctrl Pts',(81.6053429515753,-24.5991025830459,-6.25858438159219));
#11454=CARTESIAN_POINT('Ctrl Pts',(80.8996138034376,-22.6963318672728,-6.36971749958374));
#11455=CARTESIAN_POINT('Ctrl Pts',(82.1161601658834,-21.0703377293866,-6.48085061757531));
#11456=CARTESIAN_POINT('Ctrl Pts',(84.1416721090871,-21.2110239577992,-6.59198373556686));
#11457=CARTESIAN_POINT('Ctrl Pts',(85.1222604420648,-22.9887619045816,-6.70311685355843));
#11458=CARTESIAN_POINT('Ctrl Pts',(84.1604826980578,-24.7769306058564,-6.81424997154999));
#11459=CARTESIAN_POINT('Ctrl Pts',(82.1365803920894,-24.9387096606502,-6.92538308954154));
#11460=CARTESIAN_POINT('Ctrl Pts',(80.9029162629441,-23.3261418424273,-7.0365162075331));
#11461=CARTESIAN_POINT('Ctrl Pts',(81.5885844226929,-21.4150578619282,-7.14764932552466));
#11462=CARTESIAN_POINT('Ctrl Pts',(83.5660363172957,-20.9545844914355,-7.25878244351622));
#11463=CARTESIAN_POINT('Ctrl Pts',(85.0254291715253,-22.3661512964002,-7.36991556150778));
#11464=CARTESIAN_POINT('Ctrl Pts',(84.6310696902412,-24.3578436920797,-7.48104867949934));
#11465=CARTESIAN_POINT('Ctrl Pts',(82.7438909487416,-25.1067829386003,-7.5921817974909));
#11466=CARTESIAN_POINT('Ctrl Pts',(81.0911133321419,-23.9275120982265,-7.70331491548245));
#11467=CARTESIAN_POINT('Ctrl Pts',(81.1854239065361,-21.8993453878419,-7.81444803347402));
#11468=CARTESIAN_POINT('Ctrl Pts',(82.940505952956,-20.8785412458722,-7.92558115146558));
#11469=CARTESIAN_POINT('Ctrl Pts',(84.7500392877441,-21.7993795822564,-8.03671426945713));
#11470=CARTESIAN_POINT('Ctrl Pts',(84.957867788096,-23.8190730176396,-8.14784738744869));
#11471=CARTESIAN_POINT('Ctrl Pts',(83.3737786265622,-25.0891185704648,-8.25898050544025));
#11472=CARTESIAN_POINT('Ctrl Pts',(81.4475925548648,-24.4471205899292,-8.37011362343181));
#11473=CARTESIAN_POINT('Ctrl Pts',(80.942230878791,-22.4806608827483,-8.48124674142337));
#11474=CARTESIAN_POINT('Ctrl Pts',(82.3202204956144,-20.9895207789868,-8.59237985941492));
#11475=CARTESIAN_POINT('Ctrl Pts',(84.3203710706302,-21.3384503888231,-8.7035129774065));
#11476=CARTESIAN_POINT('Ctrl Pts',(85.1120660725473,-23.2080956013479,-8.81464609539804));
#11477=CARTESIAN_POINT('Ctrl Pts',(83.970715074738,-24.8872835286632,-8.9257792133896));
#11478=CARTESIAN_POINT('Ctrl Pts',(81.9409274335658,-24.839155287937,-9.03691233138117));
#11479=CARTESIAN_POINT('Ctrl Pts',(80.8804446898791,-23.1077597391704,-9.14804544937272));
#11480=CARTESIAN_POINT('Ctrl Pts',(81.7598623909015,-21.2777382357701,-9.25917856736428));
#11481=CARTESIAN_POINT('Ctrl Pts',(83.7743028431105,-21.0239984865369,-9.37031168535585));
#11482=CARTESIAN_POINT('Ctrl Pts',(85.0800708570423,-22.5787730970961,-9.4814448033474));
#11483=CARTESIAN_POINT('Ctrl Pts',(84.4820761518177,-24.5190711485177,-9.59257792133897));
#11484=CARTESIAN_POINT('Ctrl Pts',(82.5276270185007,-25.0690554947604,-9.70371103933051));
#11485=CARTESIAN_POINT('Ctrl Pts',(81.0055122302712,-23.7253588149665,-9.81484415732208));
#11486=CARTESIAN_POINT('Ctrl Pts',(81.3088311511714,-21.7177851978712,-9.92597727531363));
#11487=CARTESIAN_POINT('Ctrl Pts',(83.1599743662765,-20.8837450351666,-10.0371103933052));
#11488=CARTESIAN_POINT('Ctrl Pts',(84.8647027448359,-21.9865847112615,-10.1482435112968));
#11489=CARTESIAN_POINT('Ctrl Pts',(84.8627817773365,-24.0169419472468,-10.2593766292883));
#11490=CARTESIAN_POINT('Ctrl Pts',(83.1559696088426,-25.1165538866669,-10.3705097472799));
#11491=CARTESIAN_POINT('Ctrl Pts',(81.3064079154319,-24.2790124022603,-10.4816428652714));
#11492=CARTESIAN_POINT('Ctrl Pts',(81.0068883569529,-22.2708684258674,-10.592775983263));
#11493=CARTESIAN_POINT('Ctrl Pts',(82.5315430223004,-20.9300543644598,-10.7039091012546));
#11494=CARTESIAN_POINT('Ctrl Pts',(84.4849479519257,-21.4837360209649,-10.8150422192461));
#11495=CARTESIAN_POINT('Ctrl Pts',(85.0792700689667,-23.4251621506516,-10.9261753372377));
#11496=CARTESIAN_POINT('Ctrl Pts',(83.7705623796171,-24.9774631458428,-11.0373084552292));
#11497=CARTESIAN_POINT('Ctrl Pts',(81.7566056714021,-24.7199120377677,-11.1484415732208));
#11498=CARTESIAN_POINT('Ctrl Pts',(80.880652392244,-22.8882297376495,-11.2595746912124));
#11499=CARTESIAN_POINT('Ctrl Pts',(81.944409460413,-21.1588439808691,-11.3707078092039));
#11500=CARTESIAN_POINT('Ctrl Pts',(83.974284538051,-21.1145566799921,-11.4818409271955));
#11501=CARTESIAN_POINT('Ctrl Pts',(85.1124560589988,-22.7959013159122,-11.592974045187));
#11502=CARTESIAN_POINT('Ctrl Pts',(84.3172246492909,-24.6640451007554,-11.7041071631786));
#11503=CARTESIAN_POINT('Ctrl Pts',(82.3164173950948,-25.0091893132103,-11.8152402811701));
#11504=CARTESIAN_POINT('Ctrl Pts',(80.9412518464573,-23.5154443852944,-11.9263733991617));
#11505=CARTESIAN_POINT('Ctrl Pts',(81.4503336394796,-21.5499444682637,-12.0375065171532));
#11506=CARTESIAN_POINT('Ctrl Pts',(83.3777310799239,-20.9115924475077,-12.1486396351448));
#11507=CARTESIAN_POINT('Ctrl Pts',(84.9594141686714,-22.1846332177129,-12.2597727531364));
#11508=CARTESIAN_POINT('Ctrl Pts',(84.7477642884607,-24.2039297595911,-12.370905871128));
#11509=CARTESIAN_POINT('Ctrl Pts',(82.9364917401187,-25.1213423992779,-12.4820389891195));
#11510=CARTESIAN_POINT('Ctrl Pts',(81.1833444508808,-24.0972189799224,-12.5931721071111));
#11511=CARTESIAN_POINT('Ctrl Pts',(81.0928718230625,-22.0688775640237,-12.7043052251026));
#11512=CARTESIAN_POINT('Ctrl Pts',(82.747877966611,-20.8927360501525,-12.8154383430942));
#11513=CARTESIAN_POINT('Ctrl Pts',(84.6336361185435,-21.6452454442825,-12.9265714610857));
#11514=CARTESIAN_POINT('Ctrl Pts',(85.0242261954942,-23.637679530425,-13.0377045790773));
#11515=CARTESIAN_POINT('Ctrl Pts',(83.5621647855617,-25.0464842115007,-13.1488376970689));
#11516=CARTESIAN_POINT('Ctrl Pts',(81.585588037293,-24.5822659933775,-13.2599708150604));
#11517=CARTESIAN_POINT('Ctrl Pts',(80.9035367880058,-22.6698956607323,-13.371103933052));
#11518=CARTESIAN_POINT('Ctrl Pts',(82.1402511863244,-21.0596498121656,-13.4822370510435));
#11519=CARTESIAN_POINT('Ctrl Pts',(84.1638415383007,-21.2252888269431,-13.5933701690351));
#11520=CARTESIAN_POINT('Ctrl Pts',(85.1222383060715,-23.0152133592554,-13.7045032870266));
#11521=CARTESIAN_POINT('Ctrl Pts',(84.1382790456319,-24.7912140263811,-13.8156364050182));
#11522=CARTESIAN_POINT('Ctrl Pts',(82.1125220004198,-24.9278251150738,-13.9267695230098));
#11523=CARTESIAN_POINT('Ctrl Pts',(80.899019751184,-23.3000147799777,-14.0379026410013));
#11524=CARTESIAN_POINT('Ctrl Pts',(81.6084173195078,-21.3976191098115,-14.1490357589929));
#11525=CARTESIAN_POINT('Ctrl Pts',(83.5914461290462,-20.9617854993789,-14.2601688769844));
#11526=CARTESIAN_POINT('Ctrl Pts',(85.0331601624529,-22.3914060233836,-14.371301994976));
#11527=CARTESIAN_POINT('Ctrl Pts',(84.6140459902515,-24.3780357085581,-14.4824351129676));
#11528=CARTESIAN_POINT('Ctrl Pts',(82.7176934005918,-25.1034328748119,-14.5935682309591));
#11529=CARTESIAN_POINT('Ctrl Pts',(81.0797189200944,-23.9036854827123,-14.7047013489507));
#11530=CARTESIAN_POINT('Ctrl Pts',(81.1992612696318,-21.8768495701431,-14.8158344669422));
#11531=CARTESIAN_POINT('Ctrl Pts',(82.9669105732559,-20.8779651337157,-14.9269675849338));
#11532=CARTESIAN_POINT('Ctrl Pts',(84.7648446392386,-21.8212505374333,-15.0381007029253));
#11533=CARTESIAN_POINT('Ctrl Pts',(84.9475233946487,-23.8433738283793,-15.1492338209169));
#11534=CARTESIAN_POINT('Ctrl Pts',(83.3477521515752,-25.0936082287072,-15.2603669389085));
#11535=CARTESIAN_POINT('Ctrl Pts',(81.4297043202302,-24.4276899107226,-15.3715000569));
#11536=CARTESIAN_POINT('Ctrl Pts',(80.9488531639916,-22.4550937203094,-15.4826331748916));
#11537=CARTESIAN_POINT('Ctrl Pts',(82.345291800469,-20.9812169507322,-15.5937662928831));
#11538=CARTESIAN_POINT('Ctrl Pts',(84.3409461950547,-21.3550103921638,-15.7048994108747));
#11539=CARTESIAN_POINT('Ctrl Pts',(85.1093117692511,-23.2343620602251,-15.8160325288663));
#11540=CARTESIAN_POINT('Ctrl Pts',(83.9471563454166,-24.8992183577035,-15.9271656468579));
#11541=CARTESIAN_POINT('Ctrl Pts',(81.9181178691043,-24.8258312508155,-16.0382987648494));
#11542=CARTESIAN_POINT('Ctrl Pts',(80.8792770238047,-23.0813795174491,-16.149431882841));
#11543=CARTESIAN_POINT('Ctrl Pts',(81.7813723692392,-21.2624300969265,-16.2605650008325));
#11544=CARTESIAN_POINT('Ctrl Pts',(83.7988693899422,-21.0338048477948,-16.3716981188241));
#11545=CARTESIAN_POINT('Ctrl Pts',(85.0850786804704,-22.6046553649229,-16.4828312368156));
#11546=CARTESIAN_POINT('Ctrl Pts',(84.4632031751732,-24.5374673327142,-16.5939643548072));
#11547=CARTESIAN_POINT('Ctrl Pts',(82.5016254341118,-25.0628764630049,-16.7050974727987));
#11548=CARTESIAN_POINT('Ctrl Pts',(80.997219734115,-23.7007628417706,-16.8162305907903));
#11549=CARTESIAN_POINT('Ctrl Pts',(81.3237519397594,-21.696280307798,-16.9273637087819));
#11550=CARTESIAN_POINT('Ctrl Pts',(83.1887491753573,-20.8870198874251,-17.0384968267734));
#11551=CARTESIAN_POINT('Ctrl Pts',(84.3096484764695,-21.6342008454597,-17.1125855721011));
#11552=CARTESIAN_POINT('Ctrl Pts',(84.5881947811615,-22.162290716277,-17.149629944765));
#11553=CARTESIAN_POINT('Ctrl Pts',(84.4664903694652,-21.752733913429,-5.85037005523502));
#11554=CARTESIAN_POINT('Ctrl Pts',(84.8812182065951,-22.2403559097684,-5.88741442789887));
#11555=CARTESIAN_POINT('Ctrl Pts',(85.1785118249911,-23.6537516509257,-5.96150317322658));
#11556=CARTESIAN_POINT('Ctrl Pts',(83.6300848875513,-25.1878876651001,-6.07263629121814));
#11557=CARTESIAN_POINT('Ctrl Pts',(81.5046935938781,-24.7145063291189,-6.1837694092097));
#11558=CARTESIAN_POINT('Ctrl Pts',(80.7480335121834,-22.6744168003776,-6.29490252720125));
#11559=CARTESIAN_POINT('Ctrl Pts',(82.0523753725455,-20.931078211551,-6.40603564519282));
#11560=CARTESIAN_POINT('Ctrl Pts',(84.2240640954254,-21.0819174582576,-6.51716876318437));
#11561=CARTESIAN_POINT('Ctrl Pts',(85.2754193499133,-22.9879508757435,-6.62830188117594));
#11562=CARTESIAN_POINT('Ctrl Pts',(84.2442322035796,-24.9051678125258,-6.73943499916749));
#11563=CARTESIAN_POINT('Ctrl Pts',(82.0742692819441,-25.0786221088941,-6.85056811715905));
#11564=CARTESIAN_POINT('Ctrl Pts',(80.7515743029904,-23.3496787879405,-6.96170123515061));
#11565=CARTESIAN_POINT('Ctrl Pts',(81.4867256385136,-21.3006760442876,-7.07283435314217));
#11566=CARTESIAN_POINT('Ctrl Pts',(83.606885923895,-20.8069713148532,-7.18396747113373));
#11567=CARTESIAN_POINT('Ctrl Pts',(85.1715999777499,-22.3204078177676,-7.29510058912529));
#11568=CARTESIAN_POINT('Ctrl Pts',(84.7487804327262,-24.4558363101326,-7.40623370711685));
#11569=CARTESIAN_POINT('Ctrl Pts',(82.7254081170385,-25.2588248687773,-7.51736682510841));
#11570=CARTESIAN_POINT('Ctrl Pts',(80.9533531442496,-23.9944486236241,-7.62849994309997));
#11571=CARTESIAN_POINT('Ctrl Pts',(81.0544699071237,-21.8199135448055,-7.73963306109153));
#11572=CARTESIAN_POINT('Ctrl Pts',(82.9362123973263,-20.7254401940938,-7.85076617908308));
#11573=CARTESIAN_POINT('Ctrl Pts',(84.8763358066303,-21.7127334250377,-7.96189929707464));
#11574=CARTESIAN_POINT('Ctrl Pts',(85.0991628366174,-23.8781837310767,-8.0730324150662));
#11575=CARTESIAN_POINT('Ctrl Pts',(83.4007534148994,-25.2398857017161,-8.18416553305776));
#11576=CARTESIAN_POINT('Ctrl Pts',(81.3355586950615,-24.5515561270035,-8.29529865104933));
#11577=CARTESIAN_POINT('Ctrl Pts',(80.7937261689251,-22.4431813112383,-8.40643176904087));
#11578=CARTESIAN_POINT('Ctrl Pts',(82.2711622912557,-20.8444288780876,-8.51756488703244));
#11579=CARTESIAN_POINT('Ctrl Pts',(84.4156593713139,-21.2185399769152,-8.628698005024));
#11580=CARTESIAN_POINT('Ctrl Pts',(85.2644892749797,-23.2231134070794,-8.73983112301555));
#11581=CARTESIAN_POINT('Ctrl Pts',(84.0407694647329,-25.0234846651124,-8.85096424100712));
#11582=CARTESIAN_POINT('Ctrl Pts',(81.8644964760864,-24.9718831142117,-8.96209735899868));
#11583=CARTESIAN_POINT('Ctrl Pts',(80.7274810055036,-23.1155365245424,-9.07323047699023));
#11584=CARTESIAN_POINT('Ctrl Pts',(81.6703643641624,-21.1534463601782,-9.1843635949818));
#11585=CARTESIAN_POINT('Ctrl Pts',(83.8301825906873,-20.8813947666021,-9.29549671297334));
#11586=CARTESIAN_POINT('Ctrl Pts',(85.2301850345473,-22.5483740701311,-9.40662983096492));
#11587=CARTESIAN_POINT('Ctrl Pts',(84.5890343555619,-24.6286992004945,-9.51776294895647));
#11588=CARTESIAN_POINT('Ctrl Pts',(82.4935368905835,-25.218374717592,-9.62889606694802));
#11589=CARTESIAN_POINT('Ctrl Pts',(80.8615743975369,-23.77770637877,-9.7400291849396));
#11590=CARTESIAN_POINT('Ctrl Pts',(81.186783183476,-21.6252505518735,-9.85116230293115));
#11591=CARTESIAN_POINT('Ctrl Pts',(83.1715193674164,-20.7310195295131,-9.96229542092271));
#11592=CARTESIAN_POINT('Ctrl Pts',(84.9992742753607,-21.9134487399435,-10.0734285389143));
#11593=CARTESIAN_POINT('Ctrl Pts',(84.9972146758263,-24.0903324298184,-10.1845616569058));
#11594=CARTESIAN_POINT('Ctrl Pts',(83.167225595372,-25.2693009648573,-10.2956947748974));
#11595=CARTESIAN_POINT('Ctrl Pts',(81.1841850680979,-24.3713159380432,-10.4068278928889));
#11596=CARTESIAN_POINT('Ctrl Pts',(80.8630498362799,-22.2182485902626,-10.5179610108805));
#11597=CARTESIAN_POINT('Ctrl Pts',(82.4977355038374,-20.7806709021093,-10.6290941288721));
#11598=CARTESIAN_POINT('Ctrl Pts',(84.5921134072207,-21.3743105562877,-10.7402272468636));
#11599=CARTESIAN_POINT('Ctrl Pts',(85.2293264553427,-23.4558451758645,-10.8513603648552));
#11600=CARTESIAN_POINT('Ctrl Pts',(83.8261721861007,-25.1201723485988,-10.9624934828468));
#11601=CARTESIAN_POINT('Ctrl Pts',(81.666872614319,-24.8440343387251,-11.0736266008383));
#11602=CARTESIAN_POINT('Ctrl Pts',(80.7277036972952,-22.8801635215658,-11.1847597188299));
#11603=CARTESIAN_POINT('Ctrl Pts',(81.8682297932177,-21.0259717661873,-11.2958928368214));
#11604=CARTESIAN_POINT('Ctrl Pts',(84.0445965284286,-20.9784883473884,-11.407025954813));
#11605=CARTESIAN_POINT('Ctrl Pts',(85.264907405903,-22.7811719589829,-11.5181590728045));
#11606=CARTESIAN_POINT('Ctrl Pts',(84.4122858796081,-24.784135606704,-11.6292921907961));
#11607=CARTESIAN_POINT('Ctrl Pts',(82.2670847292654,-25.1541881242764,-11.7404253087876));
#11608=CARTESIAN_POINT('Ctrl Pts',(80.7926764819628,-23.5526428824927,-11.8515584267792));
#11609=CARTESIAN_POINT('Ctrl Pts',(81.3384975977751,-21.4452971228397,-11.9626915447708));
#11610=CARTESIAN_POINT('Ctrl Pts',(83.4049911082007,-20.7608766288728,-12.0738246627623));
#11611=CARTESIAN_POINT('Ctrl Pts',(85.1008208161065,-22.1257899751985,-12.1849577807539));
#11612=CARTESIAN_POINT('Ctrl Pts',(84.87389662561,-24.2908147447938,-12.2960908987455));
#11613=CARTESIAN_POINT('Ctrl Pts',(82.9319084875028,-25.2744350539806,-12.407224016737));
#11614=CARTESIAN_POINT('Ctrl Pts',(81.0522403816889,-24.1764028808729,-12.5183571347286));
#11615=CARTESIAN_POINT('Ctrl Pts',(80.9552385416248,-22.0016804884241,-12.6294902527201));
#11616=CARTESIAN_POINT('Ctrl Pts',(82.7296828692925,-20.7406594064427,-12.7406233707117));
#11617=CARTESIAN_POINT('Ctrl Pts',(84.7515320745623,-21.5474757624641,-12.8517564887033));
#11618=CARTESIAN_POINT('Ctrl Pts',(85.170310185562,-23.6836994714752,-12.9628896066948));
#11619=CARTESIAN_POINT('Ctrl Pts',(83.6027349921588,-25.1941745140432,-13.0740227246864));
#11620=CARTESIAN_POINT('Ctrl Pts',(81.483513010514,-24.6964546794916,-13.1851558426779));
#11621=CARTESIAN_POINT('Ctrl Pts',(80.7522396099925,-22.6460727504636,-13.2962889606695));
#11622=CARTESIAN_POINT('Ctrl Pts',(82.0782049893937,-20.9196189706525,-13.407422078661));
#11623=CARTESIAN_POINT('Ctrl Pts',(84.2478334439978,-21.0972117918987,-13.5185551966526));
#11624=CARTESIAN_POINT('Ctrl Pts',(85.2753956164136,-23.0163112742153,-13.6296883146442));
#11625=CARTESIAN_POINT('Ctrl Pts',(84.2204261619801,-24.9204820363604,-13.7408214326357));
#11626=CARTESIAN_POINT('Ctrl Pts',(82.0484746486146,-25.0669520494006,-13.8519545506273));
#11627=CARTESIAN_POINT('Ctrl Pts',(80.747396588474,-23.3216661923723,-13.9630876686188));
#11628=CARTESIAN_POINT('Ctrl Pts',(81.5079898322398,-21.2819787754613,-14.0742207866104));
#11629=CARTESIAN_POINT('Ctrl Pts',(83.6341295063454,-20.8146920038359,-14.1853539046019));
#11630=CARTESIAN_POINT('Ctrl Pts',(85.1798888974328,-22.3474851233215,-14.2964870225935));
#11631=CARTESIAN_POINT('Ctrl Pts',(84.730528169434,-24.4774855404051,-14.4076201405851));
#11632=CARTESIAN_POINT('Ctrl Pts',(82.6973199489705,-25.2552330381911,-14.5187532585766));
#11633=CARTESIAN_POINT('Ctrl Pts',(80.9411364223337,-23.9689024932297,-14.6298863765682));
#11634=CARTESIAN_POINT('Ctrl Pts',(81.0693058825373,-21.7957942530026,-14.7410194945597));
#11635=CARTESIAN_POINT('Ctrl Pts',(82.9645225814897,-20.7248225051793,-14.8521526125513));
#11636=CARTESIAN_POINT('Ctrl Pts',(84.8922096280545,-21.7361827593532,-14.9632857305429));
#11637=CARTESIAN_POINT('Ctrl Pts',(85.0880719108542,-23.9042382783319,-15.0744188485344));
#11638=CARTESIAN_POINT('Ctrl Pts',(83.3728486659716,-25.2446993688028,-15.185551966526));
#11639=CARTESIAN_POINT('Ctrl Pts',(81.3163795055442,-24.5307231780532,-15.2966850845175));
#11640=CARTESIAN_POINT('Ctrl Pts',(80.8008263700066,-22.4157690224434,-15.4078182025091));
#11641=CARTESIAN_POINT('Ctrl Pts',(82.2980429375056,-20.8355257806569,-15.5189513205006));
#11642=CARTESIAN_POINT('Ctrl Pts',(84.4377193575977,-21.2362950795827,-15.6300844384922));
#11643=CARTESIAN_POINT('Ctrl Pts',(85.2615361996211,-23.2512754590115,-15.7412175564838));
#11644=CARTESIAN_POINT('Ctrl Pts',(84.0155105532936,-25.0362808047369,-15.8523506744753));
#11645=CARTESIAN_POINT('Ctrl Pts',(81.8400407951012,-24.9575975103884,-15.9634837924669));
#11646=CARTESIAN_POINT('Ctrl Pts',(80.7262290715151,-23.0872524997498,-16.0746169104584));
#11647=CARTESIAN_POINT('Ctrl Pts',(81.6934266707275,-21.1370334663385,-16.18575002845));
#11648=CARTESIAN_POINT('Ctrl Pts',(83.8565220516287,-20.8919088315662,-16.2968831464416));
#11649=CARTESIAN_POINT('Ctrl Pts',(85.2355542616711,-22.5761242047825,-16.4080162644331));
#11650=CARTESIAN_POINT('Ctrl Pts',(84.5687993573514,-24.6484229971859,-16.5191493824247));
#11651=CARTESIAN_POINT('Ctrl Pts',(82.4656588285538,-25.2117497585901,-16.6302825004162));
#11652=CARTESIAN_POINT('Ctrl Pts',(80.8526834500174,-23.7513353678277,-16.7414156184078));
#11653=CARTESIAN_POINT('Ctrl Pts',(81.2027807728371,-21.6021937007821,-16.8525487363994));
#11654=CARTESIAN_POINT('Ctrl Pts',(83.2023707917161,-20.7345307207171,-16.9636818543909));
#11655=CARTESIAN_POINT('Ctrl Pts',(84.4041629509165,-21.5356340990305,-17.0377705997186));
#11656=CARTESIAN_POINT('Ctrl Pts',(84.7028113349605,-22.1018350641589,-17.0748149723825));
#11657=CARTESIAN_POINT('Ctrl Pts',(84.5652001142717,-21.6687801966678,-5.77555508285253));
#11658=CARTESIAN_POINT('Ctrl Pts',(85.0078433607487,-22.1892241220309,-5.81259945551639));
#11659=CARTESIAN_POINT('Ctrl Pts',(85.325147868964,-23.6977557984969,-5.88668820084409));
#11660=CARTESIAN_POINT('Ctrl Pts',(83.6724960207927,-25.3351547986483,-5.99782131883565));
#11661=CARTESIAN_POINT('Ctrl Pts',(81.4040442361811,-24.829910075192,-6.10895443682721));
#11662=CARTESIAN_POINT('Ctrl Pts',(80.5964532209291,-22.6525017334824,-6.22008755481877));
#11663=CARTESIAN_POINT('Ctrl Pts',(81.9885905792076,-20.7918186937154,-6.33122067281033));
#11664=CARTESIAN_POINT('Ctrl Pts',(84.3064560817636,-20.952810958716,-6.44235379080188));
#11665=CARTESIAN_POINT('Ctrl Pts',(85.4285782577618,-22.9871398469054,-6.55348690879345));
#11666=CARTESIAN_POINT('Ctrl Pts',(84.3279817091015,-25.0334050191953,-6.664620026785));
#11667=CARTESIAN_POINT('Ctrl Pts',(82.0119581717988,-25.218534557138,-6.77575314477657));
#11668=CARTESIAN_POINT('Ctrl Pts',(80.6002323430368,-23.3732157334538,-6.88688626276812));
#11669=CARTESIAN_POINT('Ctrl Pts',(81.3848668543341,-21.186294226647,-6.99801938075968));
#11670=CARTESIAN_POINT('Ctrl Pts',(83.6477355304943,-20.659358138271,-7.10915249875124));
#11671=CARTESIAN_POINT('Ctrl Pts',(85.3177707839745,-22.2746643391349,-7.2202856167428));
#11672=CARTESIAN_POINT('Ctrl Pts',(84.8664911752114,-24.5538289281854,-7.33141873473436));
#11673=CARTESIAN_POINT('Ctrl Pts',(82.7069252853353,-25.4108667989543,-7.44255185272592));
#11674=CARTESIAN_POINT('Ctrl Pts',(80.8155929563571,-24.0613851490217,-7.55368497071747));
#11675=CARTESIAN_POINT('Ctrl Pts',(80.9235159077116,-21.7404817017691,-7.66481808870904));
#11676=CARTESIAN_POINT('Ctrl Pts',(82.9319188416964,-20.5723391423155,-7.77595120670059));
#11677=CARTESIAN_POINT('Ctrl Pts',(85.0026323255168,-21.6260872678191,-7.88708432469216));
#11678=CARTESIAN_POINT('Ctrl Pts',(85.2404578851386,-23.9372944445138,-7.99821744268371));
#11679=CARTESIAN_POINT('Ctrl Pts',(83.4277282032368,-25.3906528329675,-8.10935056067527));
#11680=CARTESIAN_POINT('Ctrl Pts',(81.2235248352579,-24.6559916640778,-8.22048367866684));
#11681=CARTESIAN_POINT('Ctrl Pts',(80.6452214590593,-22.4057017397283,-8.33161679665839));
#11682=CARTESIAN_POINT('Ctrl Pts',(82.2221040868968,-20.6993369771883,-8.44274991464995));
#11683=CARTESIAN_POINT('Ctrl Pts',(84.5109476719975,-21.0986295650073,-8.55388303264151));
#11684=CARTESIAN_POINT('Ctrl Pts',(85.4169124774121,-23.2381312128108,-8.66501615063307));
#11685=CARTESIAN_POINT('Ctrl Pts',(84.1108238547277,-25.1596858015617,-8.77614926862463));
#11686=CARTESIAN_POINT('Ctrl Pts',(81.7880655186073,-25.1046109404864,-8.88728238661618));
#11687=CARTESIAN_POINT('Ctrl Pts',(80.5745173211281,-23.1233133099144,-8.99841550460776));
#11688=CARTESIAN_POINT('Ctrl Pts',(81.5808663374233,-21.0291544845863,-9.10954862259929));
#11689=CARTESIAN_POINT('Ctrl Pts',(83.886062338264,-20.7387910466673,-9.22068174059087));
#11690=CARTESIAN_POINT('Ctrl Pts',(85.3802992120524,-22.517975043166,-9.33181485858242));
#11691=CARTESIAN_POINT('Ctrl Pts',(84.695992559306,-24.7383272524714,-9.44294797657398));
#11692=CARTESIAN_POINT('Ctrl Pts',(82.4594467626664,-25.3676939404236,-9.55408109456554));
#11693=CARTESIAN_POINT('Ctrl Pts',(80.7176365648024,-23.8300539425735,-9.6652142125571));
#11694=CARTESIAN_POINT('Ctrl Pts',(81.0647352157808,-21.5327159058759,-9.77634733054867));
#11695=CARTESIAN_POINT('Ctrl Pts',(83.1830643685562,-20.5782940238596,-9.88748044854021));
#11696=CARTESIAN_POINT('Ctrl Pts',(85.1338458058857,-21.8403127686255,-9.99861356653179));
#11697=CARTESIAN_POINT('Ctrl Pts',(85.131647574316,-24.1637229123899,-10.1097466845233));
#11698=CARTESIAN_POINT('Ctrl Pts',(83.1784815819015,-25.4220480430476,-10.2208798025149));
#11699=CARTESIAN_POINT('Ctrl Pts',(81.061962220764,-24.4636194738261,-10.3320129205064));
#11700=CARTESIAN_POINT('Ctrl Pts',(80.7192113156071,-22.1656287546578,-10.443146038498));
#11701=CARTESIAN_POINT('Ctrl Pts',(82.4639279853743,-20.6312874397589,-10.5542791564896));
#11702=CARTESIAN_POINT('Ctrl Pts',(84.699278862516,-21.2648850916105,-10.6654122744811));
#11703=CARTESIAN_POINT('Ctrl Pts',(85.3793828417187,-23.4865282010775,-10.7765453924727));
#11704=CARTESIAN_POINT('Ctrl Pts',(83.8817819925845,-25.2628815513549,-10.8876785104643));
#11705=CARTESIAN_POINT('Ctrl Pts',(81.577139557236,-24.9681566396824,-10.9988116284558));
#11706=CARTESIAN_POINT('Ctrl Pts',(80.5747550023464,-22.8720973054821,-11.1099447464474));
#11707=CARTESIAN_POINT('Ctrl Pts',(81.7920501260224,-20.8930995515055,-11.2210778644389));
#11708=CARTESIAN_POINT('Ctrl Pts',(84.1149085188063,-20.8424200147847,-11.3322109824305));
#11709=CARTESIAN_POINT('Ctrl Pts',(85.4173587528071,-22.7664426020535,-11.443344100422));
#11710=CARTESIAN_POINT('Ctrl Pts',(84.5073471099255,-24.9042261126527,-11.5544772184136));
#11711=CARTESIAN_POINT('Ctrl Pts',(82.2177520634359,-25.2991869353425,-11.6656103364051));
#11712=CARTESIAN_POINT('Ctrl Pts',(80.6441011174686,-23.5898413796911,-11.7767434543967));
#11713=CARTESIAN_POINT('Ctrl Pts',(81.2266615560704,-21.3406497774158,-11.8878765723883));
#11714=CARTESIAN_POINT('Ctrl Pts',(83.4322511364777,-20.6101608102379,-11.9990096903798));
#11715=CARTESIAN_POINT('Ctrl Pts',(85.2422274635415,-22.0669467326842,-12.1101428083714));
#11716=CARTESIAN_POINT('Ctrl Pts',(85.0000289627594,-24.3776997299966,-12.221275926363));
#11717=CARTESIAN_POINT('Ctrl Pts',(82.9273252348868,-25.4275277086832,-12.3324090443545));
#11718=CARTESIAN_POINT('Ctrl Pts',(80.9211363124968,-24.2555867818233,-12.4435421623461));
#11719=CARTESIAN_POINT('Ctrl Pts',(80.8176052601872,-21.9344834128246,-12.5546752803376));
#11720=CARTESIAN_POINT('Ctrl Pts',(82.711487771974,-20.588582762733,-12.6658083983292));
#11721=CARTESIAN_POINT('Ctrl Pts',(84.869428030581,-21.4497060806457,-12.7769415163207));
#11722=CARTESIAN_POINT('Ctrl Pts',(85.3163941756299,-23.7297194125255,-12.8880746343123));
#11723=CARTESIAN_POINT('Ctrl Pts',(83.6433051987559,-25.3418648165858,-12.9992077523039));
#11724=CARTESIAN_POINT('Ctrl Pts',(81.3814379837349,-24.8106433656058,-13.1103408702954));
#11725=CARTESIAN_POINT('Ctrl Pts',(80.6009424319792,-22.6222498401948,-13.221473988287));
#11726=CARTESIAN_POINT('Ctrl Pts',(82.0161587924632,-20.7795881291394,-13.3326071062786));
#11727=CARTESIAN_POINT('Ctrl Pts',(84.3318253496949,-20.9691347568542,-13.4437402242701));
#11728=CARTESIAN_POINT('Ctrl Pts',(85.4285529267558,-23.0174091891753,-13.5548733422617));
#11729=CARTESIAN_POINT('Ctrl Pts',(84.3025732783284,-25.0497500463396,-13.6660064602532));
#11730=CARTESIAN_POINT('Ctrl Pts',(81.9844272968094,-25.2060789837275,-13.7771395782448));
#11731=CARTESIAN_POINT('Ctrl Pts',(80.5957734257642,-23.3433176047668,-13.8882726962363));
#11732=CARTESIAN_POINT('Ctrl Pts',(81.4075623449717,-21.1663384411112,-13.9994058142279));
#11733=CARTESIAN_POINT('Ctrl Pts',(83.6768128836446,-20.6675985082928,-14.1105389322194));
#11734=CARTESIAN_POINT('Ctrl Pts',(85.326617632413,-22.3035642232594,-14.221672050211));
#11735=CARTESIAN_POINT('Ctrl Pts',(84.8470103486162,-24.5769353722521,-14.3328051682026));
#11736=CARTESIAN_POINT('Ctrl Pts',(82.6769464973495,-25.4070332015704,-14.4439382861941));
#11737=CARTESIAN_POINT('Ctrl Pts',(80.8025539245727,-24.0341195037471,-14.5550714041857));
#11738=CARTESIAN_POINT('Ctrl Pts',(80.9393504954431,-21.714738935862,-14.6662045221772));
#11739=CARTESIAN_POINT('Ctrl Pts',(82.9621345897233,-20.571679876643,-14.7773376401688));
#11740=CARTESIAN_POINT('Ctrl Pts',(85.0195746168704,-21.6511149812732,-14.8884707581604));
#11741=CARTESIAN_POINT('Ctrl Pts',(85.2286204270596,-23.9651027282846,-14.9996038761519));
#11742=CARTESIAN_POINT('Ctrl Pts',(83.397945180368,-25.3957905088984,-15.1107369941435));
#11743=CARTESIAN_POINT('Ctrl Pts',(81.203054690858,-24.6337564453839,-15.221870112135));
#11744=CARTESIAN_POINT('Ctrl Pts',(80.6527995760217,-22.3764443245774,-15.3330032301266));
#11745=CARTESIAN_POINT('Ctrl Pts',(82.2507940745424,-20.6898346105816,-15.4441363481181));
#11746=CARTESIAN_POINT('Ctrl Pts',(84.5344925201404,-21.1175797670015,-15.5552694661097));
#11747=CARTESIAN_POINT('Ctrl Pts',(85.4137606299914,-23.2681888577979,-15.6664025841013));
#11748=CARTESIAN_POINT('Ctrl Pts',(84.0838647611703,-25.1733432517703,-15.7775357020929));
#11749=CARTESIAN_POINT('Ctrl Pts',(81.7619637210983,-25.0893637699614,-15.8886688200844));
#11750=CARTESIAN_POINT('Ctrl Pts',(80.5731811192254,-23.0931254820504,-15.999801938076));
#11751=CARTESIAN_POINT('Ctrl Pts',(81.6054809722158,-21.0116368357505,-16.1109350560675));
#11752=CARTESIAN_POINT('Ctrl Pts',(83.9141747133152,-20.7500128153374,-16.2220681740591));
#11753=CARTESIAN_POINT('Ctrl Pts',(85.3860298428717,-22.5475930446421,-16.3332012920507));
#11754=CARTESIAN_POINT('Ctrl Pts',(84.6743955395297,-24.7593786616575,-16.4443344100422));
#11755=CARTESIAN_POINT('Ctrl Pts',(82.4296922229958,-25.3606230541752,-16.5554675280338));
#11756=CARTESIAN_POINT('Ctrl Pts',(80.7081471659199,-23.8019078938848,-16.6666006460253));
#11757=CARTESIAN_POINT('Ctrl Pts',(81.0818096059147,-21.508107093766,-16.7777337640169));
#11758=CARTESIAN_POINT('Ctrl Pts',(83.2159924080748,-20.5820415540093,-16.8888668820084));
#11759=CARTESIAN_POINT('Ctrl Pts',(84.4986774253636,-21.4370673526013,-16.9629556273361));
#11760=CARTESIAN_POINT('Ctrl Pts',(84.8174278887595,-22.0413794120407,-17.));
#11761=CARTESIAN_POINT('Ctrl Pts',(84.2690708798524,-21.9206413469515,-6.));
#11762=CARTESIAN_POINT('Ctrl Pts',(84.31440005766,-21.9629286589163,-6.));
#11763=CARTESIAN_POINT('Ctrl Pts',(84.3569992287073,-22.0077850881403,-6.));
#11764=CARTESIAN_POINT('Ctrl Pts',(84.3968698737015,-22.0548656097299,-6.));
#11765=CARTESIAN_POINT('Ctrl Pts',(84.439372145716,-22.1050536399329,-6.));
#11766=CARTESIAN_POINT('Ctrl Pts',(84.4787745414504,-22.1577692838041,-6.));
#11767=CARTESIAN_POINT('Ctrl Pts',(84.5150500219472,-22.2126493042886,-6.));
#11768=CARTESIAN_POINT('Ctrl Pts',(84.5467910673818,-22.2606693222126,-6.));
#11769=CARTESIAN_POINT('Ctrl Pts',(84.5761378249178,-22.3103476665893,-6.));
#11770=CARTESIAN_POINT('Ctrl Pts',(84.6030492875067,-22.3614685512206,-6.));
#11771=CARTESIAN_POINT('Ctrl Pts',(84.6165495358461,-22.3871135579004,-6.));
#11772=CARTESIAN_POINT('Ctrl Pts',(84.6294365646594,-22.4131219455844,-6.));
#11773=CARTESIAN_POINT('Ctrl Pts',(84.6417028557084,-22.4394683134584,-6.));
#11774=CARTESIAN_POINT('Ctrl Pts',(84.6473118270288,-22.4515156406588,-6.));
#11775=CARTESIAN_POINT('Ctrl Pts',(84.6527915844349,-22.4636353215094,-6.));
#11776=CARTESIAN_POINT('Ctrl Pts',(84.6581328964447,-22.4758049682417,-6.));
#11777=CARTESIAN_POINT('Ctrl Pts',(84.6850518037078,-22.5371370138533,-6.));
#11778=CARTESIAN_POINT('Ctrl Pts',(84.7085095493669,-22.5998445222056,-6.));
#11779=CARTESIAN_POINT('Ctrl Pts',(84.7284826296036,-22.6635697254165,-6.));
#11780=CARTESIAN_POINT('Ctrl Pts',(84.7488100298177,-22.7284254058644,-6.));
#11781=CARTESIAN_POINT('Ctrl Pts',(84.7655285903436,-22.7943360504365,-6.));
#11782=CARTESIAN_POINT('Ctrl Pts',(84.7785742179873,-22.8609610235803,-6.));
#11783=CARTESIAN_POINT('Ctrl Pts',(84.7894854413479,-22.9166854381682,-6.));
#11784=CARTESIAN_POINT('Ctrl Pts',(84.7978267202991,-22.9729105003599,-6.));
#11785=CARTESIAN_POINT('Ctrl Pts',(84.8035357299874,-23.0294491921539,-6.));
#11786=CARTESIAN_POINT('Ctrl Pts',(84.8061653446974,-23.0554913577379,-6.));
#11787=CARTESIAN_POINT('Ctrl Pts',(84.8082361631249,-23.0816001759408,-6.));
#11788=CARTESIAN_POINT('Ctrl Pts',(84.8097402930293,-23.1077577720533,-6.));
#11789=CARTESIAN_POINT('Ctrl Pts',(84.8103976576895,-23.1191896831064,-6.));
#11790=CARTESIAN_POINT('Ctrl Pts',(84.810946665569,-23.1306307060492,-6.));
#11791=CARTESIAN_POINT('Ctrl Pts',(84.8113863231945,-23.1420652136516,-6.));
#11792=CARTESIAN_POINT('Ctrl Pts',(84.8140826819691,-23.2121914507941,-6.));
#11793=CARTESIAN_POINT('Ctrl Pts',(84.8126783065445,-23.2822039935574,-6.));
#11794=CARTESIAN_POINT('Ctrl Pts',(84.8071185682592,-23.3517420391025,-6.));
#11795=CARTESIAN_POINT('Ctrl Pts',(84.8021489988479,-23.4138985879056,-6.));
#11796=CARTESIAN_POINT('Ctrl Pts',(84.7938590814259,-23.4756769926154,-6.));
#11797=CARTESIAN_POINT('Ctrl Pts',(84.7821766931341,-23.5368317128957,-6.));
#11798=CARTESIAN_POINT('Ctrl Pts',(84.7694462372846,-23.6034728351621,-6.));
#11799=CARTESIAN_POINT('Ctrl Pts',(84.7526883937327,-23.6693741806892,-6.));
#11800=CARTESIAN_POINT('Ctrl Pts',(84.7321483928848,-23.7343221733006,-6.));
#11801=CARTESIAN_POINT('Ctrl Pts',(84.7242190379921,-23.7593949903273,-6.));
#11802=CARTESIAN_POINT('Ctrl Pts',(84.715725472557,-23.7843256816232,-6.));
#11803=CARTESIAN_POINT('Ctrl Pts',(84.7066797953178,-23.809101639147,-6.));
#11804=CARTESIAN_POINT('Ctrl Pts',(84.7027124228906,-23.8199682053687,-6.));
#11805=CARTESIAN_POINT('Ctrl Pts',(84.698638945642,-23.8308044388952,-6.));
#11806=CARTESIAN_POINT('Ctrl Pts',(84.6944654696784,-23.8415967394888,-6.));
#11807=CARTESIAN_POINT('Ctrl Pts',(84.6692426561464,-23.9068210723529,-6.));
#11808=CARTESIAN_POINT('Ctrl Pts',(84.6403290249097,-23.9705599886322,-6.));
#11809=CARTESIAN_POINT('Ctrl Pts',(84.6080372321188,-24.0325946845425,-6.));
#11810=CARTESIAN_POINT('Ctrl Pts',(84.5749974356073,-24.0960663456795,-6.));
#11811=CARTESIAN_POINT('Ctrl Pts',(84.5384208599741,-24.1577547385726,-6.));
#11812=CARTESIAN_POINT('Ctrl Pts',(84.4985862577967,-24.2174217857006,-6.));
#11813=CARTESIAN_POINT('Ctrl Pts',(84.4680936319117,-24.2630957687779,-6.));
#11814=CARTESIAN_POINT('Ctrl Pts',(84.4356907141024,-24.3075853544397,-6.));
#11815=CARTESIAN_POINT('Ctrl Pts',(84.4014829883928,-24.3507776514475,-6.));
#11816=CARTESIAN_POINT('Ctrl Pts',(84.3801864571408,-24.3776676619347,-6.));
#11817=CARTESIAN_POINT('Ctrl Pts',(84.3581900818954,-24.4040547371998,-6.));
#11818=CARTESIAN_POINT('Ctrl Pts',(84.3355164080287,-24.4299099472039,-6.));
#11819=CARTESIAN_POINT('Ctrl Pts',(84.3228383139497,-24.444367012556,-6.));
#11820=CARTESIAN_POINT('Ctrl Pts',(84.3099439935595,-24.458662320114,-6.));
#11821=CARTESIAN_POINT('Ctrl Pts',(84.2968610717558,-24.4727654072714,-6.));
#11822=CARTESIAN_POINT('Ctrl Pts',(84.2459898547062,-24.5276034028369,-6.));
#11823=CARTESIAN_POINT('Ctrl Pts',(84.192222096132,-24.5795964550668,-6.));
#11824=CARTESIAN_POINT('Ctrl Pts',(84.135842741352,-24.6284806457894,-6.));
#11825=CARTESIAN_POINT('Ctrl Pts',(84.0936831880685,-24.66503543879,-6.));
#11826=CARTESIAN_POINT('Ctrl Pts',(84.0500621252999,-24.6998516194455,-6.));
#11827=CARTESIAN_POINT('Ctrl Pts',(84.0050823134671,-24.7328090870297,-6.));
#11828=CARTESIAN_POINT('Ctrl Pts',(83.9910186700033,-24.7431137560509,-6.));
#11829=CARTESIAN_POINT('Ctrl Pts',(83.9768221028881,-24.7532366406933,-6.));
#11830=CARTESIAN_POINT('Ctrl Pts',(83.9624955117011,-24.7631738431009,-6.));
#11831=CARTESIAN_POINT('Ctrl Pts',(83.9487061657523,-24.7727384017579,-6.));
#11832=CARTESIAN_POINT('Ctrl Pts',(83.9348034056216,-24.782125996426,-6.));
#11833=CARTESIAN_POINT('Ctrl Pts',(83.9207951905357,-24.7913304106764,-6.));
#11834=CARTESIAN_POINT('Ctrl Pts',(83.8578415187256,-24.8326955432339,-6.));
#11835=CARTESIAN_POINT('Ctrl Pts',(83.7927303913155,-24.8703850018091,-6.));
#11836=CARTESIAN_POINT('Ctrl Pts',(83.7257230914976,-24.9041196200216,-6.));
#11837=CARTESIAN_POINT('Ctrl Pts',(83.6744957034376,-24.929909890379,-6.));
#11838=CARTESIAN_POINT('Ctrl Pts',(83.6221590906546,-24.9533882784112,-6.));
#11839=CARTESIAN_POINT('Ctrl Pts',(83.5688161346424,-24.9744147904526,-6.));
#11840=CARTESIAN_POINT('Ctrl Pts',(83.5563688919884,-24.9793211945425,-6.));
#11841=CARTESIAN_POINT('Ctrl Pts',(83.5438668104282,-24.9840940285375,-6.));
#11842=CARTESIAN_POINT('Ctrl Pts',(83.5313118283826,-24.9887338811667,-6.));
#11843=CARTESIAN_POINT('Ctrl Pts',(81.3326823670782,-23.0013023207031,-7.12851963660979));
#11844=CARTESIAN_POINT('Ctrl Pts',(81.3319480813151,-23.0867862355622,-7.12279015104505));
#11845=CARTESIAN_POINT('Ctrl Pts',(81.3379547004357,-23.1721666229398,-7.11706066548032));
#11846=CARTESIAN_POINT('Ctrl Pts',(81.351061266783,-23.2564427466052,-7.11133117991559));
#11847=CARTESIAN_POINT('Ctrl Pts',(81.4358026493434,-23.8013356687448,-7.07428680725173));
#11848=CARTESIAN_POINT('Ctrl Pts',(81.8173470757891,-24.3000664405756,-7.03724243458788));
#11849=CARTESIAN_POINT('Ctrl Pts',(82.3210929040621,-24.5244145242877,-7.00019806192403));
#11850=CARTESIAN_POINT('Ctrl Pts',(82.8248387323351,-24.7487626079999,-6.96315368926018));
#11851=CARTESIAN_POINT('Ctrl Pts',(83.4507859624355,-24.6987280035934,-6.92610931659633));
#11852=CARTESIAN_POINT('Ctrl Pts',(83.9124876344324,-24.3971906237623,-6.88906494393247));
#11853=CARTESIAN_POINT('Ctrl Pts',(84.3741893064293,-24.0956532439312,-6.85202057126862));
#11854=CARTESIAN_POINT('Ctrl Pts',(84.6716454203228,-23.5426130886755,-6.81497619860477));
#11855=CARTESIAN_POINT('Ctrl Pts',(84.6687365753584,-22.9911859317011,-6.77793182594091));
#11856=CARTESIAN_POINT('Ctrl Pts',(84.6658277303939,-22.4397587747268,-6.74088745327706));
#11857=CARTESIAN_POINT('Ctrl Pts',(84.3625539265714,-21.8899446160338,-6.70384308061321));
#11858=CARTESIAN_POINT('Ctrl Pts',(83.8976944974056,-21.5932820016675,-6.66679870794935));
#11859=CARTESIAN_POINT('Ctrl Pts',(83.4328350682397,-21.2966193873012,-6.6297543352855));
#11860=CARTESIAN_POINT('Ctrl Pts',(82.8063900137305,-21.2531083172617,-6.59270996262165));
#11861=CARTESIAN_POINT('Ctrl Pts',(82.3050423423877,-21.4827943967329,-6.5556655899578));
#11862=CARTESIAN_POINT('Ctrl Pts',(81.8036946710448,-21.7124804762041,-6.51862121729394));
#11863=CARTESIAN_POINT('Ctrl Pts',(81.4274443828683,-22.215363705186,-6.48157684463009));
#11864=CARTESIAN_POINT('Ctrl Pts',(81.3484522745435,-22.7610473034778,-6.44453247196624));
#11865=CARTESIAN_POINT('Ctrl Pts',(81.3370705402061,-22.8396732052259,-6.43919486018076));
#11866=CARTESIAN_POINT('Ctrl Pts',(81.3318602001293,-22.919187687916,-6.43385724839527));
#11867=CARTESIAN_POINT('Ctrl Pts',(81.3325225746862,-22.9987867636662,-6.42851963660979));
#11868=CARTESIAN_POINT('Ctrl Pts',(82.4698297828114,-24.9851743256717,-6.));
#11869=CARTESIAN_POINT('Ctrl Pts',(81.8097404375819,-24.8088876857537,-6.03704437266385));
#11870=CARTESIAN_POINT('Ctrl Pts',(80.6907280394499,-23.748620932819,-6.11113311799156));
#11871=CARTESIAN_POINT('Ctrl Pts',(81.1186741085106,-21.4618810792727,-6.22226623598312));
#11872=CARTESIAN_POINT('Ctrl Pts',(83.2718171975381,-20.587166548819,-6.33339935397468));
#11873=CARTESIAN_POINT('Ctrl Pts',(85.1745320976991,-21.9187032679059,-6.44453247196624));
#11874=CARTESIAN_POINT('Ctrl Pts',(85.0878555654783,-24.2409162559102,-6.55566558995779));
#11875=CARTESIAN_POINT('Ctrl Pts',(83.0898774551597,-25.4268774336938,-6.66679870794935));
#11876=CARTESIAN_POINT('Ctrl Pts',(81.0098475173314,-24.3919237452049,-6.77793182594092));
#11877=CARTESIAN_POINT('Ctrl Pts',(80.751179398391,-22.0828968633224,-6.88906494393247));
#11878=CARTESIAN_POINT('Ctrl Pts',(82.550772583103,-20.6133039463769,-7.00019806192403));
#11879=CARTESIAN_POINT('Ctrl Pts',(84.7614902208339,-21.3280765684321,-7.11133117991559));
#11880=CARTESIAN_POINT('Ctrl Pts',(85.3600357932379,-23.5730756808161,-7.22246429790715));
#11881=CARTESIAN_POINT('Ctrl Pts',(83.7985771412431,-25.2935651717014,-7.33359741589871));
#11882=CARTESIAN_POINT('Ctrl Pts',(81.5062325551516,-24.9148976561351,-7.44473053389026));
#11883=CARTESIAN_POINT('Ctrl Pts',(80.5810410755085,-22.7836383740802,-7.55586365188183));
#11884=CARTESIAN_POINT('Ctrl Pts',(81.8697768417376,-20.8504028018083,-7.66699676987338));
#11885=CARTESIAN_POINT('Ctrl Pts',(84.192936911971,-20.8845626742973,-7.77812988786495));
#11886=CARTESIAN_POINT('Ctrl Pts',(85.4242743751978,-22.854854309961,-7.8892630058565));
#11887=CARTESIAN_POINT('Ctrl Pts',(84.4368204072615,-24.9579888637226,-8.00039612384806));
#11888=CARTESIAN_POINT('Ctrl Pts',(82.1343319022801,-25.2690950090472,-8.11152924183961));
#11889=CARTESIAN_POINT('Ctrl Pts',(80.6241368864335,-23.5034360586258,-8.22266235983119));
#11890=CARTESIAN_POINT('Ctrl Pts',(81.2884253183515,-21.2770126287236,-8.33379547782273));
#11891=CARTESIAN_POINT('Ctrl Pts',(83.5192142592352,-20.6275350489011,-8.44492859581431));
#11892=CARTESIAN_POINT('Ctrl Pts',(85.2747978773029,-22.1494307757635,-8.55606171380584));
#11893=CARTESIAN_POINT('Ctrl Pts',(84.9483969412313,-24.4498009326555,-8.66719483179743));
#11894=CARTESIAN_POINT('Ctrl Pts',(82.8387464372207,-25.4232562134105,-8.77832794978897));
#11895=CARTESIAN_POINT('Ctrl Pts',(80.8766815403268,-24.1788520286966,-8.88946106778054));
#11896=CARTESIAN_POINT('Ctrl Pts',(80.8579612709353,-21.8555160684168,-9.00059418577209));
#11897=CARTESIAN_POINT('Ctrl Pts',(82.7997191561016,-20.5796568486397,-9.11172730376366));
#11898=CARTESIAN_POINT('Ctrl Pts',(84.9247819526336,-21.5189909448313,-9.22286042175521));
#11899=CARTESIAN_POINT('Ctrl Pts',(85.2882085474095,-23.8138028202287,-9.33399353974677));
#11900=CARTESIAN_POINT('Ctrl Pts',(83.5573766165987,-25.3637903236025,-9.44512665773833));
#11901=CARTESIAN_POINT('Ctrl Pts',(81.3164116681401,-24.7503438849264,-9.55625977572988));
#11902=CARTESIAN_POINT('Ctrl Pts',(80.6163330263943,-22.5349138299059,-9.66739289372145));
#11903=CARTESIAN_POINT('Ctrl Pts',(82.0978802191083,-20.7451489433667,-9.77852601171301));
#11904=CARTESIAN_POINT('Ctrl Pts',(84.4050829423841,-21.0191124939321,-9.88965912970458));
#11905=CARTESIAN_POINT('Ctrl Pts',(85.4262984532635,-23.1060622570228,-10.0007922476961));
#11906=CARTESIAN_POINT('Ctrl Pts',(84.2268701215403,-25.0959396679168,-10.1119253656877));
#11907=CARTESIAN_POINT('Ctrl Pts',(81.9045619654454,-25.1675305993517,-10.2230584836792));
#11908=CARTESIAN_POINT('Ctrl Pts',(80.5848418145963,-23.255312213087,-10.3341916016708));
#11909=CARTESIAN_POINT('Ctrl Pts',(81.4755694947281,-21.1094220404143,-10.4453247196624));
#11910=CARTESIAN_POINT('Ctrl Pts',(83.7615159742851,-20.6938632287777,-10.5564578376539));
#11911=CARTESIAN_POINT('Ctrl Pts',(85.3504930611994,-22.3889715588227,-10.6675909556455));
#11912=CARTESIAN_POINT('Ctrl Pts',(84.7882063839989,-24.6433171680781,-10.778724073637));
#11913=CARTESIAN_POINT('Ctrl Pts',(82.5892828410451,-25.3936342247751,-10.8898571916286));
#11914=CARTESIAN_POINT('Ctrl Pts',(80.7662638076366,-23.9532030264328,-11.0009903096202));
#11915=CARTESIAN_POINT('Ctrl Pts',(80.987648056479,-21.6403629005937,-11.1121234276117));
#11916=CARTESIAN_POINT('Ctrl Pts',(83.0508160094325,-20.571916162926,-11.2232565456033));
#11917=CARTESIAN_POINT('Ctrl Pts',(85.0674751504547,-21.7257473213969,-11.3343896635948));
#11918=CARTESIAN_POINT('Ctrl Pts',(85.1918996587519,-24.0458246854221,-11.4455227815864));
#11919=CARTESIAN_POINT('Ctrl Pts',(83.3102113270295,-25.4087221340905,-11.556655899578));
#11920=CARTESIAN_POINT('Ctrl Pts',(81.1446053790108,-24.5670622792599,-11.6677890175695));
#11921=CARTESIAN_POINT('Ctrl Pts',(80.6771296157422,-22.2911653474804,-11.7789221355611));
#11922=CARTESIAN_POINT('Ctrl Pts',(82.3356362554336,-20.6640217891469,-11.8900552535526));
#11923=CARTESIAN_POINT('Ctrl Pts',(84.6021947432545,-21.1748574325926,-12.0011883715442));
#11924=CARTESIAN_POINT('Ctrl Pts',(85.4023615402782,-23.356135390641,-12.1123214895358));
#11925=CARTESIAN_POINT('Ctrl Pts',(84.0037924996106,-25.2114642218224,-12.2234546075273));
#11926=CARTESIAN_POINT('Ctrl Pts',(81.6865130544115,-25.0427739548083,-12.3345877255189));
#11927=CARTESIAN_POINT('Ctrl Pts',(80.5713885601575,-23.0044565615544,-12.4457208435104));
#11928=CARTESIAN_POINT('Ctrl Pts',(81.6790248448622,-20.9620603477572,-12.556853961502));
#11929=CARTESIAN_POINT('Ctrl Pts',(83.9956695846244,-20.7848667162158,-12.6679870794935));
#11930=CARTESIAN_POINT('Ctrl Pts',(85.4010383313655,-22.6350502527901,-12.7791201974851));
#11931=CARTESIAN_POINT('Ctrl Pts',(84.6088822932929,-24.819250162293,-12.8902533154767));
#11932=CARTESIAN_POINT('Ctrl Pts',(82.3442138554089,-25.3384007182767,-13.0013864334682));
#11933=CARTESIAN_POINT('Ctrl Pts',(80.6797467085456,-23.7173548983382,-13.1125195514598));
#11934=CARTESIAN_POINT('Ctrl Pts',(81.1388666983012,-21.4397576406269,-13.2236526694513));
#11935=CARTESIAN_POINT('Ctrl Pts',(83.301369139264,-20.5901556007548,-13.3347857874429));
#11936=CARTESIAN_POINT('Ctrl Pts',(85.1880466821996,-21.946138005623,-13.4459189054345));
#11937=CARTESIAN_POINT('Ctrl Pts',(85.0721377809063,-24.2666563873492,-13.557052023426));
#11938=CARTESIAN_POINT('Ctrl Pts',(83.0597268239821,-25.4278809882634,-13.6681851414176));
#11939=CARTESIAN_POINT('Ctrl Pts',(80.9926515269193,-24.3670133482552,-13.7793182594091));
#11940=CARTESIAN_POINT('Ctrl Pts',(80.7627805608964,-22.0550012868012,-13.8904513774007));
#11941=CARTESIAN_POINT('Ctrl Pts',(82.5805008816194,-20.6078892424568,-14.0015844953923));
#11942=CARTESIAN_POINT('Ctrl Pts',(84.7821633068503,-21.3501311159715,-14.1127176133838));
#11943=CARTESIAN_POINT('Ctrl Pts',(85.3527197283046,-23.6023979303683,-14.2238507313754));
#11944=CARTESIAN_POINT('Ctrl Pts',(83.769974452434,-25.3033264487149,-14.3349838493669));
#11945=CARTESIAN_POINT('Ctrl Pts',(81.4825182514663,-24.8961599432032,-14.4461169673585));
#11946=CARTESIAN_POINT('Ctrl Pts',(80.5839210749153,-22.7535532254418,-14.55725008535));
#11947=CARTESIAN_POINT('Ctrl Pts',(81.896614425227,-20.83650429601,-14.6683832033416));
#11948=CARTESIAN_POINT('Ctrl Pts',(84.2191696850261,-20.8995717888251,-14.7795163213332));
#11949=CARTESIAN_POINT('Ctrl Pts',(85.4258928578083,-22.8850338533659,-14.8906494393247));
#11950=CARTESIAN_POINT('Ctrl Pts',(84.4123434153425,-24.9757174587147,-15.0017825573163));
#11951=CARTESIAN_POINT('Ctrl Pts',(82.1061616690569,-25.2581466855875,-15.1129156753078));
#11952=CARTESIAN_POINT('Ctrl Pts',(80.6180559858753,-23.4738311795988,-15.2240487932994));
#11953=CARTESIAN_POINT('Ctrl Pts',(81.3099991340711,-21.2558467410411,-15.335181911291));
#11954=CARTESIAN_POINT('Ctrl Pts',(83.5486977575985,-20.6341799887301,-15.4463150292825));
#11955=CARTESIAN_POINT('Ctrl Pts',(85.2852062676543,-22.1778048794721,-15.5574481472741));
#11956=CARTESIAN_POINT('Ctrl Pts',(84.9302047132626,-24.4739350041461,-15.6685812652656));
#11957=CARTESIAN_POINT('Ctrl Pts',(82.8086025236948,-25.4210620022677,-15.7797143832572));
#11958=CARTESIAN_POINT('Ctrl Pts',(80.8621774495091,-24.1523373594438,-15.8908475012488));
#11959=CARTESIAN_POINT('Ctrl Pts',(80.8723665083473,-21.8289490162655,-16.0019806192403));
#11960=CARTESIAN_POINT('Ctrl Pts',(82.8298598709625,-20.5773510168392,-16.1131137372319));
#11961=CARTESIAN_POINT('Ctrl Pts',(84.9430514548956,-21.5430599298187,-16.2242468552234));
#11962=CARTESIAN_POINT('Ctrl Pts',(85.2779271980639,-23.842211340369,-16.335379973215));
#11963=CARTESIAN_POINT('Ctrl Pts',(83.5278718822138,-25.37055054633,-16.4465130912065));
#11964=CARTESIAN_POINT('Ctrl Pts',(81.2948518464886,-24.7292431320363,-16.5576462091981));
#11965=CARTESIAN_POINT('Ctrl Pts',(80.6221226098858,-22.5053151163976,-16.6687793271897));
#11966=CARTESIAN_POINT('Ctrl Pts',(82.1263744182192,-20.7340408632062,-16.7799124451812));
#11967=CARTESIAN_POINT('Ctrl Pts',(84.4288973912168,-21.0368642183003,-16.8910455631728));
#11968=CARTESIAN_POINT('Ctrl Pts',(85.4262515865763,-23.1360153040043,-17.0021786811644));
#11969=CARTESIAN_POINT('Ctrl Pts',(84.1976570595988,-25.1115842053849,-17.1133117991559));
#11970=CARTESIAN_POINT('Ctrl Pts',(82.656339145916,-25.1379171412778,-17.1874005444836));
#11971=CARTESIAN_POINT('Ctrl Pts',(82.0504464477385,-24.8221815534923,-17.2244449171475));
#11972=CARTESIAN_POINT('Ctrl Pts',(82.5032651029123,-24.8599788000028,-5.92518502761751));
#11973=CARTESIAN_POINT('Ctrl Pts',(81.8848044607624,-24.6948097220376,-5.96222940028136));
#11974=CARTESIAN_POINT('Ctrl Pts',(80.8363628652054,-23.7014089625658,-6.03631814560907));
#11975=CARTESIAN_POINT('Ctrl Pts',(81.2373204061652,-21.5588829416944,-6.14745126360063));
#11976=CARTESIAN_POINT('Ctrl Pts',(83.2546749765797,-20.7393325064207,-6.25858438159218));
#11977=CARTESIAN_POINT('Ctrl Pts',(85.0373946757938,-21.9868955223735,-6.36971749958375));
#11978=CARTESIAN_POINT('Ctrl Pts',(84.9561844212062,-24.1626575554218,-6.4808506175753));
#11979=CARTESIAN_POINT('Ctrl Pts',(83.084209310504,-25.2738257887494,-6.59198373556687));
#11980=CARTESIAN_POINT('Ctrl Pts',(81.1353569917424,-24.3041417188516,-6.70311685355843));
#11981=CARTESIAN_POINT('Ctrl Pts',(80.8930018437615,-22.1407342067759,-6.81424997154998));
#11982=CARTESIAN_POINT('Ctrl Pts',(82.5791032248387,-20.7638215423288,-6.92538308954155));
#11983=CARTESIAN_POINT('Ctrl Pts',(84.6504013903435,-21.4335168464905,-7.0365162075331));
#11984=CARTESIAN_POINT('Ctrl Pts',(85.211199533414,-23.5369345166976,-7.14764932552466));
#11985=CARTESIAN_POINT('Ctrl Pts',(83.7482146699515,-25.1489208985946,-7.25878244351622));
#11986=CARTESIAN_POINT('Ctrl Pts',(81.600437380424,-24.7941341465723,-7.36991556150778));
#11987=CARTESIAN_POINT('Ctrl Pts',(80.7335933376483,-22.7972832752565,-7.48104867949935));
#11988=CARTESIAN_POINT('Ctrl Pts',(81.9410546537625,-20.9859676979103,-7.59218179749089));
#11989=CARTESIAN_POINT('Ctrl Pts',(84.1177040410574,-21.0179732693197,-7.70331491548246));
#11990=CARTESIAN_POINT('Ctrl Pts',(85.271386892802,-22.8640079599594,-7.81444803347401));
#11991=CARTESIAN_POINT('Ctrl Pts',(84.3462069614533,-24.834507796152,-7.92558115146557));
#11992=CARTESIAN_POINT('Ctrl Pts',(82.1889254818703,-25.1259939529954,-8.03671426945713));
#11993=CARTESIAN_POINT('Ctrl Pts',(80.7739713002549,-23.47168673506,-8.14784738744869));
#11994=CARTESIAN_POINT('Ctrl Pts',(81.3963662126195,-21.3856732671765,-8.25898050544025));
#11995=CARTESIAN_POINT('Ctrl Pts',(83.4864698794196,-20.777155156739,-8.3701136234318));
#11996=CARTESIAN_POINT('Ctrl Pts',(85.1313371684087,-22.2030721410426,-8.48124674142337));
#11997=CARTESIAN_POINT('Ctrl Pts',(84.8255207907014,-24.3583688666995,-8.59237985941493));
#11998=CARTESIAN_POINT('Ctrl Pts',(82.8489159343259,-25.2704329416477,-8.70351297740649));
#11999=CARTESIAN_POINT('Ctrl Pts',(81.0105891610751,-24.1045074245427,-8.81464609539804));
#12000=CARTESIAN_POINT('Ctrl Pts',(80.9930494902522,-21.927693239752,-8.92577921338961));
#12001=CARTESIAN_POINT('Ctrl Pts',(82.8123499186543,-20.7322964074005,-9.03691233138116));
#12002=CARTESIAN_POINT('Ctrl Pts',(84.8033950873886,-21.6123911590012,-9.14804544937273));
#12003=CARTESIAN_POINT('Ctrl Pts',(85.1439020911812,-23.7624801376049,-9.25917856736428));
#12004=CARTESIAN_POINT('Ctrl Pts',(83.522225517973,-25.2147172833623,-9.37031168535584));
#12005=CARTESIAN_POINT('Ctrl Pts',(81.4225875961138,-24.6399580009559,-9.4814448033474));
#12006=CARTESIAN_POINT('Ctrl Pts',(80.7666595926412,-22.5642446079607,-9.59257792133896));
#12007=CARTESIAN_POINT('Ctrl Pts',(82.1547726334041,-20.887351700923,-9.70371103933052));
#12008=CARTESIAN_POINT('Ctrl Pts',(84.3164710279009,-21.1440376702283,-9.81484415732208));
#12009=CARTESIAN_POINT('Ctrl Pts',(85.2732833218679,-23.0993734137057,-9.92597727531363));
#12010=CARTESIAN_POINT('Ctrl Pts',(84.1494972441019,-24.9637586976604,-10.0371103933052));
#12011=CARTESIAN_POINT('Ctrl Pts',(81.9736460447631,-25.0308347287271,-10.1482435112968));
#12012=CARTESIAN_POINT('Ctrl Pts',(80.7371543821552,-23.2392108831868,-10.2593766292883));
#12013=CARTESIAN_POINT('Ctrl Pts',(81.5717080937345,-21.2286518221053,-10.3705097472799));
#12014=CARTESIAN_POINT('Ctrl Pts',(83.7134907749496,-20.8393003330179,-10.4816428652714));
#12015=CARTESIAN_POINT('Ctrl Pts',(85.2022586162076,-22.4275062234627,-10.592775983263));
#12016=CARTESIAN_POINT('Ctrl Pts',(84.675432691858,-24.5396809513299,-10.7039091012545));
#12017=CARTESIAN_POINT('Ctrl Pts',(82.6151848235318,-25.2426790712883,-10.8150422192461));
#12018=CARTESIAN_POINT('Ctrl Pts',(80.907134950887,-23.8930890342155,-10.9261753372377));
#12019=CARTESIAN_POINT('Ctrl Pts',(81.1145575455562,-21.7261087613869,-11.0373084552292));
#12020=CARTESIAN_POINT('Ctrl Pts',(83.0476112848241,-20.7250438900076,-11.1484415732208));
#12021=CARTESIAN_POINT('Ctrl Pts',(84.9370893022592,-21.8061083918933,-11.2595746912123));
#12022=CARTESIAN_POINT('Ctrl Pts',(85.0536669471746,-23.979869484634,-11.3707078092039));
#12023=CARTESIAN_POINT('Ctrl Pts',(83.2906477704926,-25.2568154577507,-11.4818409271955));
#12024=CARTESIAN_POINT('Ctrl Pts',(81.2616163144708,-24.468235096543,-11.592974045187));
#12025=CARTESIAN_POINT('Ctrl Pts',(80.8236220295607,-22.335868185809,-11.7041071631786));
#12026=CARTESIAN_POINT('Ctrl Pts',(82.3775345245986,-20.811340851396,-11.8152402811701));
#12027=CARTESIAN_POINT('Ctrl Pts',(84.5011519227265,-21.2899605145701,-11.9263733991617));
#12028=CARTESIAN_POINT('Ctrl Pts',(85.2508559964109,-23.3336756213079,-12.0375065171533));
#12029=CARTESIAN_POINT('Ctrl Pts',(83.9404880693515,-25.0719976660802,-12.1486396351448));
#12030=CARTESIAN_POINT('Ctrl Pts',(81.769348443972,-24.9139458938225,-12.2597727531364));
#12031=CARTESIAN_POINT('Ctrl Pts',(80.7245495606423,-23.0041755073622,-12.3709058711279));
#12032=CARTESIAN_POINT('Ctrl Pts',(81.7623324802696,-21.0905835322176,-12.4820389891195));
#12033=CARTESIAN_POINT('Ctrl Pts',(83.9328774280728,-20.9245646622873,-12.593172107111));
#12034=CARTESIAN_POINT('Ctrl Pts',(85.2496162360062,-22.6580659017705,-12.7043052251026));
#12035=CARTESIAN_POINT('Ctrl Pts',(84.5074177207144,-24.7045186863484,-12.8154383430942));
#12036=CARTESIAN_POINT('Ctrl Pts',(82.3855711760416,-25.1909288799784,-12.9265714610857));
#12037=CARTESIAN_POINT('Ctrl Pts',(80.8260740747382,-23.6721147285318,-13.0377045790773));
#12038=CARTESIAN_POINT('Ctrl Pts',(81.2562395451253,-21.5381547233549,-13.1488376970688));
#12039=CARTESIAN_POINT('Ctrl Pts',(83.282363217556,-20.7421330530331,-13.2599708150604));
#12040=CARTESIAN_POINT('Ctrl Pts',(85.0500569595722,-22.0126000813523,-13.371103933052));
#12041=CARTESIAN_POINT('Ctrl Pts',(84.941457882731,-24.1867743789001,-13.4822370510435));
#12042=CARTESIAN_POINT('Ctrl Pts',(83.0559601365792,-25.2747660538938,-13.5933701690351));
#12043=CARTESIAN_POINT('Ctrl Pts',(81.1192454708557,-24.2808023024453,-13.7045032870266));
#12044=CARTESIAN_POINT('Ctrl Pts',(80.9038713759918,-22.1145978719098,-13.8156364050182));
#12045=CARTESIAN_POINT('Ctrl Pts',(82.6069567006193,-20.7587483180938,-13.9267695230098));
#12046=CARTESIAN_POINT('Ctrl Pts',(84.6697707229126,-21.4541805183588,-14.0379026410013));
#12047=CARTESIAN_POINT('Ctrl Pts',(85.2043448579832,-23.5644075510958,-14.1490357589929));
#12048=CARTESIAN_POINT('Ctrl Pts',(83.7214158170148,-25.1580665781811,-14.2601688769844));
#12049=CARTESIAN_POINT('Ctrl Pts',(81.5782186253548,-24.7765781322903,-14.371301994976));
#12050=CARTESIAN_POINT('Ctrl Pts',(80.7362917091574,-22.7690954541978,-14.4824351129676));
#12051=CARTESIAN_POINT('Ctrl Pts',(81.9661997181974,-20.9729457049286,-14.5935682309591));
#12052=CARTESIAN_POINT('Ctrl Pts',(84.1422824375826,-21.0320358302079,-14.7047013489507));
#12053=CARTESIAN_POINT('Ctrl Pts',(85.2729033053935,-22.8922842227546,-14.8158344669423));
#12054=CARTESIAN_POINT('Ctrl Pts',(84.3232736172787,-24.8511183327747,-14.9269675849338));
#12055=CARTESIAN_POINT('Ctrl Pts',(82.1625318115973,-25.1157360883498,-15.0381007029254));
#12056=CARTESIAN_POINT('Ctrl Pts',(80.768273893243,-23.443948895287,-15.1492338209169));
#12057=CARTESIAN_POINT('Ctrl Pts',(81.4165794701427,-21.3658422116044,-15.2603669389085));
#12058=CARTESIAN_POINT('Ctrl Pts',(83.5140939934316,-20.7833810317412,-15.3715000569));
#12059=CARTESIAN_POINT('Ctrl Pts',(85.1410891509651,-22.2296568246568,-15.4826331748916));
#12060=CARTESIAN_POINT('Ctrl Pts',(84.8084758602341,-24.38098091681,-15.5937662928831));
#12061=CARTESIAN_POINT('Ctrl Pts',(82.8206730544022,-25.2683771089908,-15.7048994108747));
#12062=CARTESIAN_POINT('Ctrl Pts',(80.9969997744478,-24.0796649096756,-15.8160325288663));
#12063=CARTESIAN_POINT('Ctrl Pts',(81.0065462576891,-21.9028016455272,-15.9271656468578));
#12064=CARTESIAN_POINT('Ctrl Pts',(82.8405898016374,-20.7301359934712,-16.0382987648494));
#12065=CARTESIAN_POINT('Ctrl Pts',(84.8205124188263,-21.6349422273054,-16.1494318828409));
#12066=CARTESIAN_POINT('Ctrl Pts',(85.1342691377567,-23.7890970671697,-16.2605650008325));
#12067=CARTESIAN_POINT('Ctrl Pts',(83.494581507195,-25.2210511709176,-16.371698118824));
#12068=CARTESIAN_POINT('Ctrl Pts',(81.4023874501187,-24.6201879724339,-16.4828312368156));
#12069=CARTESIAN_POINT('Ctrl Pts',(80.7720840545721,-22.5365125448765,-16.5939643548072));
#12070=CARTESIAN_POINT('Ctrl Pts',(82.1814698385731,-20.8769441546737,-16.7050974727988));
#12071=CARTESIAN_POINT('Ctrl Pts',(84.3387836124383,-21.1606698775672,-16.8162305907903));
#12072=CARTESIAN_POINT('Ctrl Pts',(85.27323941084,-23.1274374641322,-16.9273637087819));
#12073=CARTESIAN_POINT('Ctrl Pts',(84.1221265113701,-24.9784166083791,-17.0384968267734));
#12074=CARTESIAN_POINT('Ctrl Pts',(82.6780122054164,-25.003088850947,-17.1125855721011));
#12075=CARTESIAN_POINT('Ctrl Pts',(82.1103302849355,-24.7072652086133,-17.149629944765));
#12076=CARTESIAN_POINT('Ctrl Pts',(82.5367004230132,-24.7347832743338,-5.85037005523502));
#12077=CARTESIAN_POINT('Ctrl Pts',(81.9598684839428,-24.5807317583216,-5.88741442789887));
#12078=CARTESIAN_POINT('Ctrl Pts',(80.9819976909611,-23.6541969923126,-5.96150317322658));
#12079=CARTESIAN_POINT('Ctrl Pts',(81.3559667038196,-21.6558848041161,-6.07263629121814));
#12080=CARTESIAN_POINT('Ctrl Pts',(83.2375327556212,-20.8914984640225,-6.1837694092097));
#12081=CARTESIAN_POINT('Ctrl Pts',(84.9002572538884,-22.0550877768411,-6.29490252720125));
#12082=CARTESIAN_POINT('Ctrl Pts',(84.8245132769339,-24.0843988549335,-6.40603564519282));
#12083=CARTESIAN_POINT('Ctrl Pts',(83.0785411658485,-25.120774143805,-6.51716876318437));
#12084=CARTESIAN_POINT('Ctrl Pts',(81.2608664661531,-24.2163596924983,-6.62830188117594));
#12085=CARTESIAN_POINT('Ctrl Pts',(81.0348242891322,-22.1985715502295,-6.73943499916749));
#12086=CARTESIAN_POINT('Ctrl Pts',(82.6074338665743,-20.9143391382806,-6.85056811715906));
#12087=CARTESIAN_POINT('Ctrl Pts',(84.5393125598535,-21.5389571245491,-6.9617012351506));
#12088=CARTESIAN_POINT('Ctrl Pts',(85.0623632735896,-23.5007933525791,-7.07283435314218));
#12089=CARTESIAN_POINT('Ctrl Pts',(83.6978521986601,-25.0042766254877,-7.18396747113372));
#12090=CARTESIAN_POINT('Ctrl Pts',(81.6946422056962,-24.6733706370095,-7.29510058912529));
#12091=CARTESIAN_POINT('Ctrl Pts',(80.8861455997883,-22.8109281764329,-7.40623370711685));
#12092=CARTESIAN_POINT('Ctrl Pts',(82.0123324657874,-21.1215325940124,-7.5173668251084));
#12093=CARTESIAN_POINT('Ctrl Pts',(84.0424711701439,-21.1513838643421,-7.62849994309997));
#12094=CARTESIAN_POINT('Ctrl Pts',(85.1184994104062,-22.8731616099578,-7.73963306109152));
#12095=CARTESIAN_POINT('Ctrl Pts',(84.2555935156453,-24.7110267285814,-7.85076617908309));
#12096=CARTESIAN_POINT('Ctrl Pts',(82.2435190614604,-24.9828928969436,-7.96189929707464));
#12097=CARTESIAN_POINT('Ctrl Pts',(80.9238057140765,-23.4399374114941,-8.0730324150662));
#12098=CARTESIAN_POINT('Ctrl Pts',(81.5043071068873,-21.4943339056295,-8.18416553305776));
#12099=CARTESIAN_POINT('Ctrl Pts',(83.4537254996042,-20.9267752645769,-8.29529865104932));
#12100=CARTESIAN_POINT('Ctrl Pts',(84.9878764595144,-22.2567135063218,-8.40643176904088));
#12101=CARTESIAN_POINT('Ctrl Pts',(84.7026446401716,-24.2669368007434,-8.51756488703244));
#12102=CARTESIAN_POINT('Ctrl Pts',(82.859085431431,-25.117609669885,-8.628698005024));
#12103=CARTESIAN_POINT('Ctrl Pts',(81.1444967818236,-24.0301628203888,-8.73983112301555));
#12104=CARTESIAN_POINT('Ctrl Pts',(81.1281377095688,-21.9998704110872,-8.85096424100712));
#12105=CARTESIAN_POINT('Ctrl Pts',(82.8249806812072,-20.8849359661613,-8.96209735899867));
#12106=CARTESIAN_POINT('Ctrl Pts',(84.6820082221436,-21.7057913731711,-9.07323047699025));
#12107=CARTESIAN_POINT('Ctrl Pts',(84.9995956349529,-23.7111574549811,-9.18436359498178));
#12108=CARTESIAN_POINT('Ctrl Pts',(83.4870744193475,-25.0656442431221,-9.29549671297336));
#12109=CARTESIAN_POINT('Ctrl Pts',(81.5287635240873,-24.5295721169854,-9.40662983096491));
#12110=CARTESIAN_POINT('Ctrl Pts',(80.9169861588886,-22.5935753860154,-9.51776294895647));
#12111=CARTESIAN_POINT('Ctrl Pts',(82.2116650476995,-21.0295544584792,-9.62889606694803));
#12112=CARTESIAN_POINT('Ctrl Pts',(84.227859113418,-21.2689628465245,-9.74002918493959));
#12113=CARTESIAN_POINT('Ctrl Pts',(85.1202681904721,-23.0926845703885,-9.85116230293114));
#12114=CARTESIAN_POINT('Ctrl Pts',(84.0721243666637,-24.8315777274041,-9.96229542092271));
#12115=CARTESIAN_POINT('Ctrl Pts',(82.0427301240806,-24.8941388581025,-10.0734285389143));
#12116=CARTESIAN_POINT('Ctrl Pts',(80.8894669497142,-23.2231095532865,-10.1845616569058));
#12117=CARTESIAN_POINT('Ctrl Pts',(81.6678466927408,-21.3478816037963,-10.2956947748974));
#12118=CARTESIAN_POINT('Ctrl Pts',(83.6654655756142,-20.9847374372581,-10.4068278928889));
#12119=CARTESIAN_POINT('Ctrl Pts',(85.0540241712157,-22.4660408881028,-10.5179610108805));
#12120=CARTESIAN_POINT('Ctrl Pts',(84.5626589997171,-24.4360447345817,-10.629094128872));
#12121=CARTESIAN_POINT('Ctrl Pts',(82.6410868060184,-25.0917239178013,-10.7402272468636));
#12122=CARTESIAN_POINT('Ctrl Pts',(81.0480060941376,-23.8329750419982,-10.8513603648552));
#12123=CARTESIAN_POINT('Ctrl Pts',(81.2414670346331,-21.81185462218,-10.9624934828467));
#12124=CARTESIAN_POINT('Ctrl Pts',(83.0444065602159,-20.8781716170892,-11.0736266008383));
#12125=CARTESIAN_POINT('Ctrl Pts',(84.8067034540636,-21.8864694623896,-11.1847597188299));
#12126=CARTESIAN_POINT('Ctrl Pts',(84.9154342355974,-23.913914283846,-11.2958928368214));
#12127=CARTESIAN_POINT('Ctrl Pts',(83.2710842139556,-25.1049087814108,-11.407025954813));
#12128=CARTESIAN_POINT('Ctrl Pts',(81.3786272499309,-24.3694079138262,-11.5181590728045));
#12129=CARTESIAN_POINT('Ctrl Pts',(80.9701144433791,-22.3805710241376,-11.6292921907961));
#12130=CARTESIAN_POINT('Ctrl Pts',(82.4194327937636,-20.9586599136451,-11.7404253087876));
#12131=CARTESIAN_POINT('Ctrl Pts',(84.4001091021983,-21.4050635965476,-11.8515584267792));
#12132=CARTESIAN_POINT('Ctrl Pts',(85.0993504525439,-23.3112158519747,-11.9626915447708));
#12133=CARTESIAN_POINT('Ctrl Pts',(83.8771836390926,-24.9325311103381,-12.0738246627623));
#12134=CARTESIAN_POINT('Ctrl Pts',(81.8521838335323,-24.7851178328367,-12.1849577807539));
#12135=CARTESIAN_POINT('Ctrl Pts',(80.8777105611273,-23.00389445317,-12.2960908987455));
#12136=CARTESIAN_POINT('Ctrl Pts',(81.8456401156769,-21.2191067166779,-12.407224016737));
#12137=CARTESIAN_POINT('Ctrl Pts',(83.8700852715213,-21.0642626083588,-12.5183571347286));
#12138=CARTESIAN_POINT('Ctrl Pts',(85.0981941406469,-22.681081550751,-12.6294902527201));
#12139=CARTESIAN_POINT('Ctrl Pts',(84.4059531481358,-24.5897872104038,-12.7406233707117));
#12140=CARTESIAN_POINT('Ctrl Pts',(82.4269284966742,-25.0434570416802,-12.8517564887032));
#12141=CARTESIAN_POINT('Ctrl Pts',(80.9724014409309,-23.6268745587255,-12.9628896066948));
#12142=CARTESIAN_POINT('Ctrl Pts',(81.3736123919494,-21.636551806083,-13.0740227246864));
#12143=CARTESIAN_POINT('Ctrl Pts',(83.263357295848,-20.8941105053114,-13.1851558426779));
#12144=CARTESIAN_POINT('Ctrl Pts',(84.912067236945,-22.0790621570815,-13.2962889606695));
#12145=CARTESIAN_POINT('Ctrl Pts',(84.8107779845556,-24.1068923704511,-13.407422078661));
#12146=CARTESIAN_POINT('Ctrl Pts',(83.0521934491764,-25.1216511195243,-13.5185551966526));
#12147=CARTESIAN_POINT('Ctrl Pts',(81.2458394147922,-24.1945912566353,-13.6296883146442));
#12148=CARTESIAN_POINT('Ctrl Pts',(81.0449621910871,-22.1741944570185,-13.7408214326357));
#12149=CARTESIAN_POINT('Ctrl Pts',(82.6334125196193,-20.9096073937307,-13.8519545506273));
#12150=CARTESIAN_POINT('Ctrl Pts',(84.5573781389748,-21.5582299207461,-13.9630876686188));
#12151=CARTESIAN_POINT('Ctrl Pts',(85.055969987662,-23.5264171718233,-14.0742207866104));
#12152=CARTESIAN_POINT('Ctrl Pts',(83.6728571815953,-25.0128067076473,-14.1853539046019));
#12153=CARTESIAN_POINT('Ctrl Pts',(81.6739189992434,-24.6569963213773,-14.2964870225935));
#12154=CARTESIAN_POINT('Ctrl Pts',(80.8886623433994,-22.7846376829539,-14.4076201405851));
#12155=CARTESIAN_POINT('Ctrl Pts',(82.0357850111679,-21.1093871138471,-14.5187532585766));
#12156=CARTESIAN_POINT('Ctrl Pts',(84.0653951901389,-21.1644998715908,-14.6298863765682));
#12157=CARTESIAN_POINT('Ctrl Pts',(85.1199137529788,-22.8995345921432,-14.7410194945598));
#12158=CARTESIAN_POINT('Ctrl Pts',(84.234203819215,-24.7265192068348,-14.8521526125513));
#12159=CARTESIAN_POINT('Ctrl Pts',(82.2189019541376,-24.9733254911122,-14.9632857305429));
#12160=CARTESIAN_POINT('Ctrl Pts',(80.9184918006105,-23.4140666109752,-15.0744188485344));
#12161=CARTESIAN_POINT('Ctrl Pts',(81.5231598062145,-21.4758376821678,-15.185551966526));
#12162=CARTESIAN_POINT('Ctrl Pts',(83.4794902292645,-20.9325820747523,-15.2966850845175));
#12163=CARTESIAN_POINT('Ctrl Pts',(84.9969720342762,-22.2815087698416,-15.4078182025091));
#12164=CARTESIAN_POINT('Ctrl Pts',(84.6867470072055,-24.2880268294738,-15.5189513205007));
#12165=CARTESIAN_POINT('Ctrl Pts',(82.8327435851099,-25.1156922157141,-15.6300844384922));
#12166=CARTESIAN_POINT('Ctrl Pts',(81.1318220993863,-24.0069924599074,-15.7412175564838));
#12167=CARTESIAN_POINT('Ctrl Pts',(81.140726007031,-21.976654274789,-15.8523506744753));
#12168=CARTESIAN_POINT('Ctrl Pts',(82.8513197323124,-20.8829209701032,-15.9634837924669));
#12169=CARTESIAN_POINT('Ctrl Pts',(84.6979733827568,-21.7268245247922,-16.0746169104585));
#12170=CARTESIAN_POINT('Ctrl Pts',(84.9906110774499,-23.7359827939705,-16.18575002845));
#12171=CARTESIAN_POINT('Ctrl Pts',(83.4612911321759,-25.0715517955052,-16.2968831464416));
#12172=CARTESIAN_POINT('Ctrl Pts',(81.5099230537491,-24.5111328128315,-16.4080162644331));
#12173=CARTESIAN_POINT('Ctrl Pts',(80.9220454992582,-22.5677099733552,-16.5191493824247));
#12174=CARTESIAN_POINT('Ctrl Pts',(82.2365652589273,-21.0198474461412,-16.6302825004163));
#12175=CARTESIAN_POINT('Ctrl Pts',(84.2486698336597,-21.2844755368341,-16.7414156184078));
#12176=CARTESIAN_POINT('Ctrl Pts',(85.120227235104,-23.1188596242601,-16.8525487363994));
#12177=CARTESIAN_POINT('Ctrl Pts',(84.0465959631413,-24.8452490113732,-16.9636818543909));
#12178=CARTESIAN_POINT('Ctrl Pts',(82.6996852649168,-24.8682605606161,-17.0377705997186));
#12179=CARTESIAN_POINT('Ctrl Pts',(82.1702141221325,-24.5923488637344,-17.0748149723825));
#12180=CARTESIAN_POINT('Ctrl Pts',(82.5701357431142,-24.6095877486648,-5.77555508285253));
#12181=CARTESIAN_POINT('Ctrl Pts',(82.0349325071233,-24.4666537946055,-5.81259945551638));
#12182=CARTESIAN_POINT('Ctrl Pts',(81.1276325167165,-23.6069850220594,-5.88668820084409));
#12183=CARTESIAN_POINT('Ctrl Pts',(81.4746130014742,-21.7528866665377,-5.99782131883565));
#12184=CARTESIAN_POINT('Ctrl Pts',(83.2203905346628,-21.0436644216242,-6.10895443682721));
#12185=CARTESIAN_POINT('Ctrl Pts',(84.7631198319829,-22.1232800313086,-6.22008755481877));
#12186=CARTESIAN_POINT('Ctrl Pts',(84.6928421326618,-24.0061401544452,-6.33122067281032));
#12187=CARTESIAN_POINT('Ctrl Pts',(83.0728730211929,-24.9677224988606,-6.44235379080189));
#12188=CARTESIAN_POINT('Ctrl Pts',(81.3863759405641,-24.1285776661449,-6.55348690879345));
#12189=CARTESIAN_POINT('Ctrl Pts',(81.1766467345028,-22.256408893683,-6.66462002678501));
#12190=CARTESIAN_POINT('Ctrl Pts',(82.6357645083098,-21.0648567342324,-6.77575314477657));
#12191=CARTESIAN_POINT('Ctrl Pts',(84.4282237293633,-21.6443974026076,-6.88688626276812));
#12192=CARTESIAN_POINT('Ctrl Pts',(84.9135270137654,-23.4646521884607,-6.99801938075969));
#12193=CARTESIAN_POINT('Ctrl Pts',(83.6474897273688,-24.8596323523809,-7.10915249875124));
#12194=CARTESIAN_POINT('Ctrl Pts',(81.7888470309685,-24.5526071274467,-7.2202856167428));
#12195=CARTESIAN_POINT('Ctrl Pts',(81.0386978619283,-22.8245730776092,-7.33141873473436));
#12196=CARTESIAN_POINT('Ctrl Pts',(82.0836102778123,-21.2570974901144,-7.44255185272592));
#12197=CARTESIAN_POINT('Ctrl Pts',(83.9672382992303,-21.2847944593645,-7.55368497071748));
#12198=CARTESIAN_POINT('Ctrl Pts',(84.9656119280105,-22.8823152599562,-7.66481808870903));
#12199=CARTESIAN_POINT('Ctrl Pts',(84.164980069837,-24.5875456610108,-7.7759512067006));
#12200=CARTESIAN_POINT('Ctrl Pts',(82.2981126410506,-24.8397918408919,-7.88708432469216));
#12201=CARTESIAN_POINT('Ctrl Pts',(81.0736401278978,-23.4081880879282,-7.99821744268371));
#12202=CARTESIAN_POINT('Ctrl Pts',(81.6122480011553,-21.6029945440825,-8.10935056067529));
#12203=CARTESIAN_POINT('Ctrl Pts',(83.4209811197886,-21.0763953724148,-8.22048367866682));
#12204=CARTESIAN_POINT('Ctrl Pts',(84.8444157506201,-22.3103548716009,-8.3316167966584));
#12205=CARTESIAN_POINT('Ctrl Pts',(84.5797684896418,-24.1755047347873,-8.44274991464994));
#12206=CARTESIAN_POINT('Ctrl Pts',(82.8692549285362,-24.9647863981223,-8.55388303264151));
#12207=CARTESIAN_POINT('Ctrl Pts',(81.2784044025718,-23.9558182162349,-8.66501615063306));
#12208=CARTESIAN_POINT('Ctrl Pts',(81.2632259288858,-22.0720475824224,-8.77614926862463));
#12209=CARTESIAN_POINT('Ctrl Pts',(82.8376114437597,-21.0375755249222,-8.88728238661619));
#12210=CARTESIAN_POINT('Ctrl Pts',(84.5606213568987,-21.799191587341,-8.99841550460775));
#12211=CARTESIAN_POINT('Ctrl Pts',(84.8552891787246,-23.6598347723572,-9.10954862259931));
#12212=CARTESIAN_POINT('Ctrl Pts',(83.4519233207219,-24.9165712028819,-9.22068174059086));
#12213=CARTESIAN_POINT('Ctrl Pts',(81.6349394520607,-24.419186233015,-9.33181485858243));
#12214=CARTESIAN_POINT('Ctrl Pts',(81.0673127251357,-22.6229061640702,-9.44294797657398));
#12215=CARTESIAN_POINT('Ctrl Pts',(82.2685574619953,-21.1717572160355,-9.55408109456555));
#12216=CARTESIAN_POINT('Ctrl Pts',(84.139247198935,-21.3938880228207,-9.66521421255709));
#12217=CARTESIAN_POINT('Ctrl Pts',(84.9672530590764,-23.0859957270714,-9.77634733054866));
#12218=CARTESIAN_POINT('Ctrl Pts',(83.9947514892254,-24.6993967571477,-9.88748044854022));
#12219=CARTESIAN_POINT('Ctrl Pts',(82.1118142033981,-24.7574429874778,-9.99861356653178));
#12220=CARTESIAN_POINT('Ctrl Pts',(81.0417795172734,-23.2070082233863,-10.1097466845233));
#12221=CARTESIAN_POINT('Ctrl Pts',(81.7639852917469,-21.4671113854874,-10.2208798025149));
#12222=CARTESIAN_POINT('Ctrl Pts',(83.6174403762788,-21.1301745414983,-10.3320129205065));
#12223=CARTESIAN_POINT('Ctrl Pts',(84.9057897262238,-22.5045755527429,-10.443146038498));
#12224=CARTESIAN_POINT('Ctrl Pts',(84.4498853075762,-24.3324085178334,-10.5542791564896));
#12225=CARTESIAN_POINT('Ctrl Pts',(82.6669887885052,-24.9407687643145,-10.6654122744811));
#12226=CARTESIAN_POINT('Ctrl Pts',(81.1888772373878,-23.7728610497808,-10.7765453924727));
#12227=CARTESIAN_POINT('Ctrl Pts',(81.3683765237105,-21.8976004829732,-10.8876785104643));
#12228=CARTESIAN_POINT('Ctrl Pts',(83.0412018356075,-21.0312993441707,-10.9988116284558));
#12229=CARTESIAN_POINT('Ctrl Pts',(84.6763176058681,-21.9668305328859,-11.1099447464474));
#12230=CARTESIAN_POINT('Ctrl Pts',(84.7772015240203,-23.8479590830579,-11.2210778644389));
#12231=CARTESIAN_POINT('Ctrl Pts',(83.2515206574186,-24.953002105071,-11.3322109824305));
#12232=CARTESIAN_POINT('Ctrl Pts',(81.495638185391,-24.2705807311094,-11.443344100422));
#12233=CARTESIAN_POINT('Ctrl Pts',(81.1166068571975,-22.4252738624662,-11.5544772184136));
#12234=CARTESIAN_POINT('Ctrl Pts',(82.4613310629286,-21.1059789758943,-11.6656103364052));
#12235=CARTESIAN_POINT('Ctrl Pts',(84.2990662816703,-21.520166678525,-11.7767434543967));
#12236=CARTESIAN_POINT('Ctrl Pts',(84.9478449086767,-23.2887560826416,-11.8878765723883));
#12237=CARTESIAN_POINT('Ctrl Pts',(83.8138792088337,-24.793064554596,-11.9990096903798));
#12238=CARTESIAN_POINT('Ctrl Pts',(81.9350192230927,-24.6562897718509,-12.1101428083714));
#12239=CARTESIAN_POINT('Ctrl Pts',(81.0308715616122,-23.0036133989778,-12.221275926363));
#12240=CARTESIAN_POINT('Ctrl Pts',(81.9289477510842,-21.3476299011382,-12.3324090443545));
#12241=CARTESIAN_POINT('Ctrl Pts',(83.8072931149699,-21.2039605544302,-12.4435421623461));
#12242=CARTESIAN_POINT('Ctrl Pts',(84.9467720452876,-22.7040971997315,-12.5546752803376));
#12243=CARTESIAN_POINT('Ctrl Pts',(84.3044885755572,-24.4750557344592,-12.6658083983292));
#12244=CARTESIAN_POINT('Ctrl Pts',(82.4682858173069,-24.8959852033819,-12.7769415163208));
#12245=CARTESIAN_POINT('Ctrl Pts',(81.1187288071235,-23.5816343889191,-12.8880746343123));
#12246=CARTESIAN_POINT('Ctrl Pts',(81.4909852387734,-21.734948888811,-12.9992077523039));
#12247=CARTESIAN_POINT('Ctrl Pts',(83.24435137414,-21.0460879575897,-13.1103408702954));
#12248=CARTESIAN_POINT('Ctrl Pts',(84.7740775143177,-22.1455242328108,-13.221473988287));
#12249=CARTESIAN_POINT('Ctrl Pts',(84.6800980863804,-24.027010362002,-13.3326071062785));
#12250=CARTESIAN_POINT('Ctrl Pts',(83.0484267617735,-24.9685361851548,-13.4437402242701));
#12251=CARTESIAN_POINT('Ctrl Pts',(81.3724333587286,-24.1083802108253,-13.5548733422617));
#12252=CARTESIAN_POINT('Ctrl Pts',(81.1860530061824,-22.2337910421272,-13.6660064602532));
#12253=CARTESIAN_POINT('Ctrl Pts',(82.6598683386192,-21.0604664693676,-13.7771395782448));
#12254=CARTESIAN_POINT('Ctrl Pts',(84.4449855550371,-21.6622793231335,-13.8882726962364));
#12255=CARTESIAN_POINT('Ctrl Pts',(84.9075951173406,-23.4884267925507,-13.9994058142279));
#12256=CARTESIAN_POINT('Ctrl Pts',(83.6242985461759,-24.8675468371136,-14.1105389322195));
#12257=CARTESIAN_POINT('Ctrl Pts',(81.769619373132,-24.5374145104643,-14.221672050211));
#12258=CARTESIAN_POINT('Ctrl Pts',(81.0410329776415,-22.80017991171,-14.3328051682026));
#12259=CARTESIAN_POINT('Ctrl Pts',(82.1053703041383,-21.2458285227657,-14.4439382861941));
#12260=CARTESIAN_POINT('Ctrl Pts',(83.9885079426954,-21.2969639129736,-14.5550714041857));
#12261=CARTESIAN_POINT('Ctrl Pts',(84.9669242005639,-22.9067849615319,-14.6662045221773));
#12262=CARTESIAN_POINT('Ctrl Pts',(84.1451340211513,-24.6019200808948,-14.7773376401688));
#12263=CARTESIAN_POINT('Ctrl Pts',(82.275272096678,-24.8309148938745,-14.8884707581604));
#12264=CARTESIAN_POINT('Ctrl Pts',(81.0687097079781,-23.3841843266634,-14.9996038761519));
#12265=CARTESIAN_POINT('Ctrl Pts',(81.6297401422862,-21.5858331527312,-15.1107369941435));
#12266=CARTESIAN_POINT('Ctrl Pts',(83.4448864650975,-21.0817831177634,-15.221870112135));
#12267=CARTESIAN_POINT('Ctrl Pts',(84.8528549175871,-22.3333607150264,-15.3330032301266));
#12268=CARTESIAN_POINT('Ctrl Pts',(84.565018154177,-24.1950727421377,-15.4441363481182));
#12269=CARTESIAN_POINT('Ctrl Pts',(82.8448141158174,-24.9630073224372,-15.5552694661097));
#12270=CARTESIAN_POINT('Ctrl Pts',(81.2666444243251,-23.9343200101391,-15.6664025841013));
#12271=CARTESIAN_POINT('Ctrl Pts',(81.2749057563727,-22.0505069040507,-15.7775357020928));
#12272=CARTESIAN_POINT('Ctrl Pts',(82.8620496629874,-21.0357059467352,-15.8886688200844));
#12273=CARTESIAN_POINT('Ctrl Pts',(84.5754343466875,-21.818706822279,-15.999801938076));
#12274=CARTESIAN_POINT('Ctrl Pts',(84.8469530171428,-23.6828685207713,-16.1109350560675));
#12275=CARTESIAN_POINT('Ctrl Pts',(83.428000757157,-24.9220524200928,-16.2220681740591));
#12276=CARTESIAN_POINT('Ctrl Pts',(81.6174586573793,-24.4020776532291,-16.3332012920507));
#12277=CARTESIAN_POINT('Ctrl Pts',(81.0720069439444,-22.598907401834,-16.4443344100422));
#12278=CARTESIAN_POINT('Ctrl Pts',(82.2916606792813,-21.1627507376087,-16.5554675280338));
#12279=CARTESIAN_POINT('Ctrl Pts',(84.1585560548812,-21.4082811961009,-16.6666006460253));
#12280=CARTESIAN_POINT('Ctrl Pts',(84.9672150593679,-23.1102817843879,-16.7777337640169));
#12281=CARTESIAN_POINT('Ctrl Pts',(83.9710654149125,-24.7120814143673,-16.8888668820084));
#12282=CARTESIAN_POINT('Ctrl Pts',(82.7213583244171,-24.7334322702853,-16.9629556273361));
#12283=CARTESIAN_POINT('Ctrl Pts',(82.2300979593295,-24.4774325188554,-17.));
#12284=CARTESIAN_POINT('Ctrl Pts',(81.3361555725406,-22.9990558295284,-6.62148036339021));
#12285=CARTESIAN_POINT('Ctrl Pts',(81.3350366720467,-22.7833631289824,-6.63586025118848));
#12286=CARTESIAN_POINT('Ctrl Pts',(81.3739566040229,-22.5680575720948,-6.65024013898675));
#12287=CARTESIAN_POINT('Ctrl Pts',(81.4547878978142,-22.3698449958516,-6.66462002678502));
#12288=CARTESIAN_POINT('Ctrl Pts',(81.6630193257718,-21.8592248405328,-6.70166439944887));
#12289=CARTESIAN_POINT('Ctrl Pts',(82.1493919170408,-21.4620407873826,-6.73870877211272));
#12290=CARTESIAN_POINT('Ctrl Pts',(82.6913214161842,-21.3600388722033,-6.77575314477657));
#12291=CARTESIAN_POINT('Ctrl Pts',(83.2332509153276,-21.2580369570241,-6.81279751744043));
#12292=CARTESIAN_POINT('Ctrl Pts',(83.8307373223455,-21.4512171798158,-6.84984189010428));
#12293=CARTESIAN_POINT('Ctrl Pts',(84.2103644065881,-21.8511830888539,-6.88688626276813));
#12294=CARTESIAN_POINT('Ctrl Pts',(84.5899914908307,-22.2511489978919,-6.92393063543198));
#12295=CARTESIAN_POINT('Ctrl Pts',(84.751759252298,-22.8579005931763,-6.96097500809584));
#12296=CARTESIAN_POINT('Ctrl Pts',(84.6216369186323,-23.3937730848052,-6.99801938075969));
#12297=CARTESIAN_POINT('Ctrl Pts',(84.4915145849665,-23.9296455764341,-7.03506375342355));
#12298=CARTESIAN_POINT('Ctrl Pts',(84.0695021561676,-24.3946389644075,-7.0721081260874));
#12299=CARTESIAN_POINT('Ctrl Pts',(83.5487221590348,-24.5759647875718,-7.10915249875125));
#12300=CARTESIAN_POINT('Ctrl Pts',(83.027942161902,-24.7572906107362,-7.1461968714151));
#12301=CARTESIAN_POINT('Ctrl Pts',(82.4083945964353,-24.6549488690914,-7.18324124407896));
#12302=CARTESIAN_POINT('Ctrl Pts',(81.9735959521952,-24.3157723232961,-7.22028561674281));
#12303=CARTESIAN_POINT('Ctrl Pts',(81.5776803201884,-24.0069275321053,-7.25401719895861));
#12304=CARTESIAN_POINT('Ctrl Pts',(81.3349477858388,-23.5017130479715,-7.28774878117441));
#12305=CARTESIAN_POINT('Ctrl Pts',(81.3317907907837,-22.9991411291167,-7.32148036339021));
#12306=CARTESIAN_POINT('Ctrl Pts',(82.4698297828114,-24.9851743256717,-6.));
#12307=CARTESIAN_POINT('Ctrl Pts',(82.4011651403016,-24.9597503542562,-6.));
#12308=CARTESIAN_POINT('Ctrl Pts',(82.3342038415895,-24.9304366816692,-6.));
#12309=CARTESIAN_POINT('Ctrl Pts',(82.2691348210017,-24.897527340086,-6.));
#12310=CARTESIAN_POINT('Ctrl Pts',(82.2022547374464,-24.8637020343576,-6.));
#12311=CARTESIAN_POINT('Ctrl Pts',(82.1373729617415,-24.826077429436,-6.));
#12312=CARTESIAN_POINT('Ctrl Pts',(82.0747258622901,-24.7849281529323,-6.));
#12313=CARTESIAN_POINT('Ctrl Pts',(82.0217931318391,-24.7501596867064,-6.));
#12314=CARTESIAN_POINT('Ctrl Pts',(81.9704561050628,-24.7128738527553,-6.));
#12315=CARTESIAN_POINT('Ctrl Pts',(81.9208801018963,-24.6732182969939,-6.));
#12316=CARTESIAN_POINT('Ctrl Pts',(81.8988503779666,-24.6555968493195,-6.));
#12317=CARTESIAN_POINT('Ctrl Pts',(81.877168685752,-24.6375073018008,-6.));
#12318=CARTESIAN_POINT('Ctrl Pts',(81.8558510844111,-24.6189618853867,-6.));
#12319=CARTESIAN_POINT('Ctrl Pts',(81.8441385439209,-24.6087724678633,-6.));
#12320=CARTESIAN_POINT('Ctrl Pts',(81.8325359306331,-24.5984454288214,-6.));
#12321=CARTESIAN_POINT('Ctrl Pts',(81.8210460423394,-24.5879827552104,-6.));
#12322=CARTESIAN_POINT('Ctrl Pts',(81.8104524505223,-24.5783362477147,-6.));
#12323=CARTESIAN_POINT('Ctrl Pts',(81.7999532489741,-24.5685729257818,-6.));
#12324=CARTESIAN_POINT('Ctrl Pts',(81.7895665184221,-24.5587098024996,-6.));
#12325=CARTESIAN_POINT('Ctrl Pts',(81.7364817644389,-24.5083011132282,-6.));
#12326=CARTESIAN_POINT('Ctrl Pts',(81.6862370051735,-24.4552040168816,-6.));
#12327=CARTESIAN_POINT('Ctrl Pts',(81.6390509066064,-24.3996779857533,-6.));
#12328=CARTESIAN_POINT('Ctrl Pts',(81.5922309432753,-24.3445828026317,-6.));
#12329=CARTESIAN_POINT('Ctrl Pts',(81.5484218497577,-24.2870953491844,-6.));
#12330=CARTESIAN_POINT('Ctrl Pts',(81.5078820330439,-24.2274448646231,-6.));
#12331=CARTESIAN_POINT('Ctrl Pts',(81.4741936202512,-24.1778755692962,-6.));
#12332=CARTESIAN_POINT('Ctrl Pts',(81.4427634629306,-24.1268119328391,-6.));
#12333=CARTESIAN_POINT('Ctrl Pts',(81.4137674499962,-24.0743790286647,-6.));
#12334=CARTESIAN_POINT('Ctrl Pts',(81.4016612987905,-24.052487720107,-6.));
#12335=CARTESIAN_POINT('Ctrl Pts',(81.3899797780391,-24.0303576880886,-6.));
#12336=CARTESIAN_POINT('Ctrl Pts',(81.3787371301748,-24.0079979523352,-6.));
#12337=CARTESIAN_POINT('Ctrl Pts',(81.3735363240541,-23.9976544236606,-6.));
#12338=CARTESIAN_POINT('Ctrl Pts',(81.3684294470406,-23.9872617395261,-6.));
#12339=CARTESIAN_POINT('Ctrl Pts',(81.3634179742616,-23.9768207948056,-6.));
#12340=CARTESIAN_POINT('Ctrl Pts',(81.358185972138,-23.9659203973858,-6.));
#12341=CARTESIAN_POINT('Ctrl Pts',(81.3530615649057,-23.9549748511129,-6.));
#12342=CARTESIAN_POINT('Ctrl Pts',(81.3480478111895,-23.9439894637078,-6.));
#12343=CARTESIAN_POINT('Ctrl Pts',(81.3195074050713,-23.881455993647,-6.));
#12344=CARTESIAN_POINT('Ctrl Pts',(81.2945279707571,-23.8175894738114,-6.));
#12345=CARTESIAN_POINT('Ctrl Pts',(81.273332967452,-23.7525943637814,-6.));
#12346=CARTESIAN_POINT('Ctrl Pts',(81.2541305056381,-23.6937094416857,-6.));
#12347=CARTESIAN_POINT('Ctrl Pts',(81.238034694834,-23.6338975545441,-6.));
#12348=CARTESIAN_POINT('Ctrl Pts',(81.2252484092018,-23.5733059254121,-6.));
#12349=CARTESIAN_POINT('Ctrl Pts',(81.2101158950681,-23.5015959925516,-6.));
#12350=CARTESIAN_POINT('Ctrl Pts',(81.199618304078,-23.4287923860598,-6.));
#12351=CARTESIAN_POINT('Ctrl Pts',(81.1936804986385,-23.3553182001535,-6.));
#12352=CARTESIAN_POINT('Ctrl Pts',(81.1923736703968,-23.3391475556011,-6.));
#12353=CARTESIAN_POINT('Ctrl Pts',(81.1912879323035,-23.3229445113856,-6.));
#12354=CARTESIAN_POINT('Ctrl Pts',(81.1904228526274,-23.3067137422975,-6.));
#12355=CARTESIAN_POINT('Ctrl Pts',(81.189527519046,-23.2899153443931,-6.));
#12356=CARTESIAN_POINT('Ctrl Pts',(81.1888685376905,-23.2730810540116,-6.));
#12357=CARTESIAN_POINT('Ctrl Pts',(81.1884459909198,-23.2562503281413,-6.));
#12358=CARTESIAN_POINT('Ctrl Pts',(81.1867247251221,-23.1876895088514,-6.));
#12359=CARTESIAN_POINT('Ctrl Pts',(81.1889150608861,-23.1191011358685,-6.));
#12360=CARTESIAN_POINT('Ctrl Pts',(81.1948964151315,-23.0508235285529,-6.));
#12361=CARTESIAN_POINT('Ctrl Pts',(81.2008765342427,-22.9825600203863,-6.));
#12362=CARTESIAN_POINT('Ctrl Pts',(81.2106465599838,-22.9146060779743,-6.));
#12363=CARTESIAN_POINT('Ctrl Pts',(81.2241355890059,-22.847314844313,-6.));
#12364=CARTESIAN_POINT('Ctrl Pts',(81.2338955811021,-22.79862624652,-6.));
#12365=CARTESIAN_POINT('Ctrl Pts',(81.2456036149723,-22.7502848589497,-6.));
#12366=CARTESIAN_POINT('Ctrl Pts',(81.2592470358225,-22.7024341008059,-6.));
#12367=CARTESIAN_POINT('Ctrl Pts',(81.2694833999489,-22.6665327099841,-6.));
#12368=CARTESIAN_POINT('Ctrl Pts',(81.2808094768484,-22.6309076580324,-6.));
#12369=CARTESIAN_POINT('Ctrl Pts',(81.2932238368812,-22.5956236937823,-6.));
#12370=CARTESIAN_POINT('Ctrl Pts',(81.297353318441,-22.5838869244811,-6.));
#12371=CARTESIAN_POINT('Ctrl Pts',(81.3016000214654,-22.5721970897154,-6.));
#12372=CARTESIAN_POINT('Ctrl Pts',(81.3059633013415,-22.5605567493468,-6.));
#12373=CARTESIAN_POINT('Ctrl Pts',(81.3290872411027,-22.498866796576,-6.));
#12374=CARTESIAN_POINT('Ctrl Pts',(81.3554837726698,-22.4385603794557,-6.));
#12375=CARTESIAN_POINT('Ctrl Pts',(81.3851029023407,-22.3799715846882,-6.));
#12376=CARTESIAN_POINT('Ctrl Pts',(81.4059352506056,-22.3387636832211,-6.));
#12377=CARTESIAN_POINT('Ctrl Pts',(81.4283626361963,-22.2984059990452,-6.));
#12378=CARTESIAN_POINT('Ctrl Pts',(81.4523780657584,-22.2590261197136,-6.));
#12379=CARTESIAN_POINT('Ctrl Pts',(81.460091074361,-22.2463785279948,-6.));
#12380=CARTESIAN_POINT('Ctrl Pts',(81.4679690461019,-22.233830189719,-6.));
#12381=CARTESIAN_POINT('Ctrl Pts',(81.4760084245406,-22.2213909668549,-6.));
#12382=CARTESIAN_POINT('Ctrl Pts',(81.5102529655807,-22.1684048459597,-6.));
#12383=CARTESIAN_POINT('Ctrl Pts',(81.547353278539,-22.1175025084971,-6.));
#12384=CARTESIAN_POINT('Ctrl Pts',(81.5872751269259,-22.0689991728902,-6.));
#12385=CARTESIAN_POINT('Ctrl Pts',(81.6240617830979,-22.0243049615181,-6.));
#12386=CARTESIAN_POINT('Ctrl Pts',(81.6632447942969,-21.9816476511376,-6.));
#12387=CARTESIAN_POINT('Ctrl Pts',(81.7048188123851,-21.9413067695052,-6.));
#12388=CARTESIAN_POINT('Ctrl Pts',(81.7126371595806,-21.9337203240935,-6.));
#12389=CARTESIAN_POINT('Ctrl Pts',(81.720540120158,-21.9262159047748,-6.));
#12390=CARTESIAN_POINT('Ctrl Pts',(81.7285261019851,-21.9187941775198,-6.));
#12391=CARTESIAN_POINT('Origin',(83.,-23.,-12.));
#12392=CARTESIAN_POINT('Origin',(83.,23.,-17.));
#12393=CARTESIAN_POINT('Ctrl Pts',(82.2300979593296,21.5225674811446,-17.));
#12394=CARTESIAN_POINT('Ctrl Pts',(82.2818391122695,21.4874949137045,-17.));
#12395=CARTESIAN_POINT('Ctrl Pts',(82.3355567543514,21.4556774402474,-17.));
#12396=CARTESIAN_POINT('Ctrl Pts',(82.3909195853492,21.4270510150662,-17.));
#12397=CARTESIAN_POINT('Ctrl Pts',(82.4260296219145,21.4088966899218,-17.));
#12398=CARTESIAN_POINT('Ctrl Pts',(82.4618022221282,21.3920264043057,-17.));
#12399=CARTESIAN_POINT('Ctrl Pts',(82.4981604879293,21.3764310360441,-17.));
#12400=CARTESIAN_POINT('Ctrl Pts',(82.5229436776791,21.3658006343369,-17.));
#12401=CARTESIAN_POINT('Ctrl Pts',(82.5479991038361,21.3557627158986,-17.));
#12402=CARTESIAN_POINT('Ctrl Pts',(82.5733036534702,21.3463159755545,-17.));
#12403=CARTESIAN_POINT('Ctrl Pts',(82.5867940813383,21.3412797045659,-17.));
#12404=CARTESIAN_POINT('Ctrl Pts',(82.6003552710179,21.3364116315714,-17.));
#12405=CARTESIAN_POINT('Ctrl Pts',(82.6139700106875,21.3317160828494,-17.));
#12406=CARTESIAN_POINT('Ctrl Pts',(82.6763343043471,21.3102074395331,-17.));
#12407=CARTESIAN_POINT('Ctrl Pts',(82.7398899091068,21.2922884683847,-17.));
#12408=CARTESIAN_POINT('Ctrl Pts',(82.8042869308727,21.2779126212872,-17.));
#12409=CARTESIAN_POINT('Ctrl Pts',(82.850739552613,21.2675426419139,-17.));
#12410=CARTESIAN_POINT('Ctrl Pts',(82.8976308987338,21.2590171252843,-17.));
#12411=CARTESIAN_POINT('Ctrl Pts',(82.9448387498772,21.252332630243,-17.));
#12412=CARTESIAN_POINT('Ctrl Pts',(82.9577364929077,21.2505063471726,-17.));
#12413=CARTESIAN_POINT('Ctrl Pts',(82.9706578945276,21.2488175569436,-17.));
#12414=CARTESIAN_POINT('Ctrl Pts',(82.9836005288407,21.2472663500385,-17.));
#12415=CARTESIAN_POINT('Ctrl Pts',(82.9969336049753,21.2456683477103,-17.));
#12416=CARTESIAN_POINT('Ctrl Pts',(83.010281297855,21.2442173442006,-17.));
#12417=CARTESIAN_POINT('Ctrl Pts',(83.0236353363373,21.2429134174335,-17.));
#12418=CARTESIAN_POINT('Ctrl Pts',(83.0911664964694,21.236319480519,-17.));
#12419=CARTESIAN_POINT('Ctrl Pts',(83.1589013412011,21.2334779274394,-17.));
#12420=CARTESIAN_POINT('Ctrl Pts',(83.2264851933794,21.2343408033929,-17.));
#12421=CARTESIAN_POINT('Ctrl Pts',(83.295047717335,21.2352161745257,-17.));
#12422=CARTESIAN_POINT('Ctrl Pts',(83.3634558539945,21.2399037043402,-17.));
#12423=CARTESIAN_POINT('Ctrl Pts',(83.4313607857131,21.2484016191192,-17.));
#12424=CARTESIAN_POINT('Ctrl Pts',(83.4734288208429,21.2536661937003,-17.));
#12425=CARTESIAN_POINT('Ctrl Pts',(83.5153040946816,21.2603941539428,-17.));
#12426=CARTESIAN_POINT('Ctrl Pts',(83.556905046585,21.2685950224746,-17.));
#12427=CARTESIAN_POINT('Ctrl Pts',(83.5909685001726,21.2753100107581,-17.));
#12428=CARTESIAN_POINT('Ctrl Pts',(83.6248480727517,21.2830126560453,-17.));
#12429=CARTESIAN_POINT('Ctrl Pts',(83.658498645678,21.2917121682308,-17.));
#12430=CARTESIAN_POINT('Ctrl Pts',(83.6722821813049,21.2952755558857,-17.));
#12431=CARTESIAN_POINT('Ctrl Pts',(83.686029760402,21.2990070804481,-17.));
#12432=CARTESIAN_POINT('Ctrl Pts',(83.6997150233873,21.3029005333424,-17.));
#12433=CARTESIAN_POINT('Ctrl Pts',(83.7675103738305,21.3221882886225,-17.));
#12434=CARTESIAN_POINT('Ctrl Pts',(83.833896115477,21.3454752233121,-17.));
#12435=CARTESIAN_POINT('Ctrl Pts',(83.8985095148681,21.372742621713,-17.));
#12436=CARTESIAN_POINT('Ctrl Pts',(83.905676412587,21.3757671128749,-17.));
#12437=CARTESIAN_POINT('Ctrl Pts',(83.912821512826,21.3788406285709,-17.));
#12438=CARTESIAN_POINT('Ctrl Pts',(83.9199443247218,21.3819631826297,-17.));
#12439=CARTESIAN_POINT('Ctrl Pts',(83.9816969964304,21.4090348024489,-17.));
#12440=CARTESIAN_POINT('Ctrl Pts',(84.0417752134862,21.4397880070069,-17.));
#12441=CARTESIAN_POINT('Ctrl Pts',(84.1000370416108,21.4739125980637,-17.));
#12442=CARTESIAN_POINT('Ctrl Pts',(84.1627128975786,21.5106225335889,-17.));
#12443=CARTESIAN_POINT('Ctrl Pts',(84.2232877181478,21.5512340617636,-17.));
#12444=CARTESIAN_POINT('Ctrl Pts',(84.2815649194341,21.595422083472,-17.));
#12445=CARTESIAN_POINT('Ctrl Pts',(84.2920904904965,21.6034029774122,-17.));
#12446=CARTESIAN_POINT('Ctrl Pts',(84.3025410380364,21.6115006876682,-17.));
#12447=CARTESIAN_POINT('Ctrl Pts',(84.3129152988056,21.619713487774,-17.));
#12448=CARTESIAN_POINT('Ctrl Pts',(84.3220910240519,21.626977465319,-17.));
#12449=CARTESIAN_POINT('Ctrl Pts',(84.3312000707531,21.6343259558301,-17.));
#12450=CARTESIAN_POINT('Ctrl Pts',(84.3402397897604,21.6417556641301,-17.));
#12451=CARTESIAN_POINT('Ctrl Pts',(84.3951430096276,21.6868803973225,-17.));
#12452=CARTESIAN_POINT('Ctrl Pts',(84.4475140924687,21.7350158683439,-17.));
#12453=CARTESIAN_POINT('Ctrl Pts',(84.4972030228202,21.7858120772864,-17.));
#12454=CARTESIAN_POINT('Ctrl Pts',(84.5479396850435,21.8376793659784,-17.));
#12455=CARTESIAN_POINT('Ctrl Pts',(84.595880656229,21.892321324379,-17.));
#12456=CARTESIAN_POINT('Ctrl Pts',(84.6408460217217,21.9494166317566,-17.));
#12457=CARTESIAN_POINT('Ctrl Pts',(84.6860841326239,22.0068582608603,-17.));
#12458=CARTESIAN_POINT('Ctrl Pts',(84.728311217856,22.0667838205659,-17.));
#12459=CARTESIAN_POINT('Ctrl Pts',(84.7673121163611,22.1289076492861,-17.));
#12460=CARTESIAN_POINT('Ctrl Pts',(84.7769392049,22.1442424652105,-17.));
#12461=CARTESIAN_POINT('Ctrl Pts',(84.7863695336446,22.1597113916503,-17.));
#12462=CARTESIAN_POINT('Ctrl Pts',(84.7955994818445,22.1753104375009,-17.));
#12463=CARTESIAN_POINT('Ctrl Pts',(84.8028490082894,22.1875624775946,-17.));
#12464=CARTESIAN_POINT('Ctrl Pts',(84.8099756566119,22.1998963399229,-17.));
#12465=CARTESIAN_POINT('Ctrl Pts',(84.8169672073596,22.2122910124967,-17.));
#12466=CARTESIAN_POINT('Ctrl Pts',(84.8539823502387,22.2779117299617,-17.));
#12467=CARTESIAN_POINT('Ctrl Pts',(84.8872834125653,22.3453494005186,-17.));
#12468=CARTESIAN_POINT('Ctrl Pts',(84.9166896640119,22.414257705163,-17.));
#12469=CARTESIAN_POINT('Ctrl Pts',(84.946127984178,22.4832411571309,-17.));
#12470=CARTESIAN_POINT('Ctrl Pts',(84.9716637589054,22.5536992817437,-17.));
#12471=CARTESIAN_POINT('Ctrl Pts',(84.9930799285708,22.6253223370055,-17.));
#12472=CARTESIAN_POINT('Ctrl Pts',(85.014008872031,22.6953159398509,-17.));
#12473=CARTESIAN_POINT('Ctrl Pts',(85.0310040806236,22.7664229483095,-17.));
#12474=CARTESIAN_POINT('Ctrl Pts',(85.0438193705755,22.8383774944687,-17.));
#12475=CARTESIAN_POINT('Ctrl Pts',(85.0465681840663,22.8538113729024,-17.));
#12476=CARTESIAN_POINT('Ctrl Pts',(85.0491245073901,22.8692843043202,-17.));
#12477=CARTESIAN_POINT('Ctrl Pts',(85.0514856033279,22.8847937492575,-17.));
#12478=CARTESIAN_POINT('Ctrl Pts',(85.0534987896279,22.8980178633515,-17.));
#12479=CARTESIAN_POINT('Ctrl Pts',(85.0553700412629,22.9112685237034,-17.));
#12480=CARTESIAN_POINT('Ctrl Pts',(85.0571001857713,22.9245440319506,-17.));
#12481=CARTESIAN_POINT('Ctrl Pts',(84.8174278887595,23.9586205879593,-17.));
#12482=CARTESIAN_POINT('Ctrl Pts',(84.7765814369624,24.021100311179,-17.));
#12483=CARTESIAN_POINT('Ctrl Pts',(84.7321382857191,24.0810293094923,-17.));
#12484=CARTESIAN_POINT('Ctrl Pts',(84.6844272864798,24.1382578115838,-17.));
#12485=CARTESIAN_POINT('Ctrl Pts',(84.6379676938528,24.1939852735153,-17.));
#12486=CARTESIAN_POINT('Ctrl Pts',(84.5884084330975,24.2471522504166,-17.));
#12487=CARTESIAN_POINT('Ctrl Pts',(84.5360270889349,24.2975827793496,-17.));
#12488=CARTESIAN_POINT('Ctrl Pts',(84.524335411062,24.3088390292354,-17.));
#12489=CARTESIAN_POINT('Ctrl Pts',(84.5125014719912,24.3199602485304,-17.));
#12490=CARTESIAN_POINT('Ctrl Pts',(84.5005333434906,24.3309395401516,-17.));
#12491=CARTESIAN_POINT('Ctrl Pts',(84.4456121081234,24.3813230449125,-17.));
#12492=CARTESIAN_POINT('Ctrl Pts',(84.3879771334341,24.4286220664064,-17.));
#12493=CARTESIAN_POINT('Ctrl Pts',(84.3279445697082,24.4726641188265,-17.));
#12494=CARTESIAN_POINT('Ctrl Pts',(84.2858000274712,24.5035828739691,-17.));
#12495=CARTESIAN_POINT('Ctrl Pts',(84.2424731669021,24.5328955590232,-17.));
#12496=CARTESIAN_POINT('Ctrl Pts',(84.1980680473418,24.5605280932164,-17.));
#12497=CARTESIAN_POINT('Ctrl Pts',(84.1811926620229,24.5710293522259,-17.));
#12498=CARTESIAN_POINT('Ctrl Pts',(84.1641615210443,24.5812878268755,-17.));
#12499=CARTESIAN_POINT('Ctrl Pts',(84.1469802604654,24.5912989639673,-17.));
#12500=CARTESIAN_POINT('Ctrl Pts',(84.1305954137665,24.6008460484653,-17.));
#12501=CARTESIAN_POINT('Ctrl Pts',(84.1140687260479,24.6101709300663,-17.));
#12502=CARTESIAN_POINT('Ctrl Pts',(84.0974346776955,24.6192537517685,-17.));
#12503=CARTESIAN_POINT('Ctrl Pts',(84.0337176308478,24.6540456775616,-17.));
#12504=CARTESIAN_POINT('Ctrl Pts',(83.968361627354,24.6853304511806,-17.));
#12505=CARTESIAN_POINT('Ctrl Pts',(83.9016583718977,24.7129464384693,-17.));
#12506=CARTESIAN_POINT('Ctrl Pts',(83.8363874432689,24.7399694244241,-17.));
#12507=CARTESIAN_POINT('Ctrl Pts',(83.7698255763795,24.7634796468367,-17.));
#12508=CARTESIAN_POINT('Ctrl Pts',(83.7022374818724,24.7832774030826,-17.));
#12509=CARTESIAN_POINT('Ctrl Pts',(83.6361317195128,24.8026409578506,-17.));
#12510=CARTESIAN_POINT('Ctrl Pts',(83.5690434882077,24.818453214359,-17.));
#12511=CARTESIAN_POINT('Ctrl Pts',(83.501224394617,24.8304787382213,-17.));
#12512=CARTESIAN_POINT('Ctrl Pts',(83.4791642918285,24.8343903843144,-17.));
#12513=CARTESIAN_POINT('Ctrl Pts',(83.4570269381163,24.8379009736306,-17.));
#12514=CARTESIAN_POINT('Ctrl Pts',(83.4348212870326,24.8410012299466,-17.));
#12515=CARTESIAN_POINT('Ctrl Pts',(83.4223367367169,24.8427442685012,-17.));
#12516=CARTESIAN_POINT('Ctrl Pts',(83.4098293128072,24.8443576459882,-17.));
#12517=CARTESIAN_POINT('Ctrl Pts',(83.3973183107669,24.8458378344555,-17.));
#12518=CARTESIAN_POINT('Ctrl Pts',(83.3294876076222,24.8538629490063,-17.));
#12519=CARTESIAN_POINT('Ctrl Pts',(83.2614333839518,24.857994846758,-17.));
#12520=CARTESIAN_POINT('Ctrl Pts',(83.1934013670207,24.8580554883464,-17.));
#12521=CARTESIAN_POINT('Ctrl Pts',(83.1836044640327,24.8580642209959,-17.));
#12522=CARTESIAN_POINT('Ctrl Pts',(83.1738080277562,24.8579884388901,-17.));
#12523=CARTESIAN_POINT('Ctrl Pts',(83.1640128014146,24.8578275203802,-17.));
#12524=CARTESIAN_POINT('Ctrl Pts',(83.0946485636743,24.8566879867553,-17.));
#12525=CARTESIAN_POINT('Ctrl Pts',(83.0253435429726,24.8512831792143,-17.));
#12526=CARTESIAN_POINT('Ctrl Pts',(82.9564227427862,24.8417863242814,-17.));
#12527=CARTESIAN_POINT('Ctrl Pts',(82.892127503802,24.8329268427337,-17.));
#12528=CARTESIAN_POINT('Ctrl Pts',(82.8281661293059,24.8205052274388,-17.));
#12529=CARTESIAN_POINT('Ctrl Pts',(82.7648229902021,24.8046276724132,-17.));
#12530=CARTESIAN_POINT('Ctrl Pts',(82.7509583247458,24.8011523632982,-17.));
#12531=CARTESIAN_POINT('Ctrl Pts',(82.7371233769276,24.7975113717667,-17.));
#12532=CARTESIAN_POINT('Ctrl Pts',(82.7233213065985,24.7937056333022,-17.));
#12533=CARTESIAN_POINT('Ctrl Pts',(82.712260901116,24.7906558726812,-17.));
#12534=CARTESIAN_POINT('Ctrl Pts',(82.7012221546017,24.7875003763038,-17.));
#12535=CARTESIAN_POINT('Ctrl Pts',(82.6902197481713,24.7842437511852,-17.));
#12536=CARTESIAN_POINT('Ctrl Pts',(82.6246575930502,24.7648378727943,-17.));
#12537=CARTESIAN_POINT('Ctrl Pts',(82.5602618201431,24.7418119987196,-17.));
#12538=CARTESIAN_POINT('Ctrl Pts',(82.4973348852617,24.715348146897,-17.));
#12539=CARTESIAN_POINT('Ctrl Pts',(82.4346992973391,24.6890068207108,-17.));
#12540=CARTESIAN_POINT('Ctrl Pts',(82.3735180853771,24.6592585759547,-17.));
#12541=CARTESIAN_POINT('Ctrl Pts',(82.3141193166054,24.626241363502,-17.));
#12542=CARTESIAN_POINT('Ctrl Pts',(82.2559932421632,24.5939315869093,-17.));
#12543=CARTESIAN_POINT('Ctrl Pts',(82.1995733746079,24.5584907230117,-17.));
#12544=CARTESIAN_POINT('Ctrl Pts',(82.1452070792864,24.5200186444709,-17.));
#12545=CARTESIAN_POINT('Ctrl Pts',(82.1337105081942,24.5118831446471,-17.));
#12546=CARTESIAN_POINT('Ctrl Pts',(82.1223059328567,24.5036120109462,-17.));
#12547=CARTESIAN_POINT('Ctrl Pts',(82.1109969163345,24.4952060590793,-17.));
#12548=CARTESIAN_POINT('Ctrl Pts',(82.1003659149212,24.4873040734378,-17.));
#12549=CARTESIAN_POINT('Ctrl Pts',(82.0898181260854,24.4792818391566,-17.));
#12550=CARTESIAN_POINT('Ctrl Pts',(82.0793730883428,24.4711532945118,-17.));
#12551=CARTESIAN_POINT('Ctrl Pts',(82.0278057382619,24.4310225149325,-17.));
#12552=CARTESIAN_POINT('Ctrl Pts',(81.9786449613375,24.388234245707,-17.));
#12553=CARTESIAN_POINT('Ctrl Pts',(81.9321818346833,24.3429204973124,-17.));
#12554=CARTESIAN_POINT('Ctrl Pts',(81.8866023381703,24.2984685203218,-17.));
#12555=CARTESIAN_POINT('Ctrl Pts',(81.8436182780009,24.2515855470076,-17.));
#12556=CARTESIAN_POINT('Ctrl Pts',(81.8035469551829,24.2023704370989,-17.));
#12557=CARTESIAN_POINT('Ctrl Pts',(81.7647767394068,24.1547533309887,-17.));
#12558=CARTESIAN_POINT('Ctrl Pts',(81.7287328388918,24.1049525046523,-17.));
#12559=CARTESIAN_POINT('Ctrl Pts',(81.6957493048722,24.0530421344184,-17.));
#12560=CARTESIAN_POINT('Ctrl Pts',(81.6902970764157,24.0444612710819,-17.));
#12561=CARTESIAN_POINT('Ctrl Pts',(81.6849285841721,24.035822741006,-17.));
#12562=CARTESIAN_POINT('Ctrl Pts',(81.6796454747864,24.0271268532951,-17.));
#12563=CARTESIAN_POINT('Ctrl Pts',(81.6739898969948,24.0178178903669,-17.));
#12564=CARTESIAN_POINT('Ctrl Pts',(81.6684321663704,24.0084431960771,-17.));
#12565=CARTESIAN_POINT('Ctrl Pts',(81.6629726863575,23.9990044309052,-17.));
#12566=CARTESIAN_POINT('Origin',(83.,23.,-4.45407471946233));
#12567=CARTESIAN_POINT('Ctrl Pts',(80.9434277056327,23.0014963838888,-6.20407471946233));
#12568=CARTESIAN_POINT('Ctrl Pts',(80.942610779565,23.0996693924379,-6.20941233124781));
#12569=CARTESIAN_POINT('Ctrl Pts',(80.9936360048529,23.8783594097717,-6.25179431569715));
#12570=CARTESIAN_POINT('Ctrl Pts',(81.9885904398633,25.2081812989956,-6.33122067281032));
#12571=CARTESIAN_POINT('Ctrl Pts',(84.3064562032972,25.0471892646279,-6.44235379080189));
#12572=CARTESIAN_POINT('Ctrl Pts',(85.4285783999577,23.0128601032299,-6.55348690879345));
#12573=CARTESIAN_POINT('Ctrl Pts',(84.3279818049202,20.9665948756778,-6.664620026785));
#12574=CARTESIAN_POINT('Ctrl Pts',(82.0119581026862,20.781465281165,-6.77575314477657));
#12575=CARTESIAN_POINT('Ctrl Pts',(80.9980257384601,22.1068136403803,-6.855571375669));
#12576=CARTESIAN_POINT('Ctrl Pts',(80.9427191451532,22.892962770366,-6.89834523389759));
#12577=CARTESIAN_POINT('Ctrl Pts',(80.943624771683,22.9983937941554,-6.90407471946232));
#12578=CARTESIAN_POINT('Ctrl Pts',(80.9473274657881,22.9976809234163,-6.14592528053767));
#12579=CARTESIAN_POINT('Ctrl Pts',(80.9508754982181,23.4678290021184,-6.17137226568616));
#12580=CARTESIAN_POINT('Ctrl Pts',(81.3433671991295,24.6294006980789,-6.23386362349849));
#12581=CARTESIAN_POINT('Ctrl Pts',(83.2718171861771,25.4128332182024,-6.33339935397467));
#12582=CARTESIAN_POINT('Ctrl Pts',(85.1745320403748,24.0812968093214,-6.44453247196624));
#12583=CARTESIAN_POINT('Ctrl Pts',(85.0878555272437,21.7590837146758,-6.55566558995779));
#12584=CARTESIAN_POINT('Ctrl Pts',(83.0898774457969,20.5731226537472,-6.66679870794935));
#12585=CARTESIAN_POINT('Ctrl Pts',(81.2789896272084,21.4741601405839,-6.76355193814265));
#12586=CARTESIAN_POINT('Ctrl Pts',(80.9500836416261,22.5818790379909,-6.82326079567209));
#12587=CARTESIAN_POINT('Ctrl Pts',(80.9479086080167,23.0011644845222,-6.84592528053768));
#12588=CARTESIAN_POINT('Ctrl Pts',(84.2690708798524,24.0793586530485,-6.));
#12589=CARTESIAN_POINT('Ctrl Pts',(84.627967898288,23.6573805147568,-6.03704437266385));
#12590=CARTESIAN_POINT('Ctrl Pts',(84.8852386427553,22.4342554940614,-6.11113311799156));
#12591=CARTESIAN_POINT('Ctrl Pts',(83.5452631709912,21.1066470201579,-6.22226623598311));
#12592=CARTESIAN_POINT('Ctrl Pts',(81.705991976553,21.516300728788,-6.33339935397468));
#12593=CARTESIAN_POINT('Ctrl Pts',(81.0511940873356,23.2817532913239,-6.44453247196623));
#12594=CARTESIAN_POINT('Ctrl Pts',(82.1799448462403,24.7904027468678,-6.5556655899578));
#12595=CARTESIAN_POINT('Ctrl Pts',(84.0592802212889,24.6598697237475,-6.66679870794935));
#12596=CARTESIAN_POINT('Ctrl Pts',(84.9691016495094,23.0104270261496,-6.77793182594091));
#12597=CARTESIAN_POINT('Ctrl Pts',(84.0767332702261,21.3513065155757,-6.88906494393247));
#12598=CARTESIAN_POINT('Ctrl Pts',(82.1988914461979,21.201202656489,-7.00019806192403));
#12599=CARTESIAN_POINT('Ctrl Pts',(81.0542580966476,22.697395090279,-7.11133117991559));
#12600=CARTESIAN_POINT('Ctrl Pts',(81.6904431199867,24.4705604132256,-7.22246429790715));
#12601=CARTESIAN_POINT('Ctrl Pts',(83.5251867456106,24.8978024588301,-7.33359741589872));
#12602=CARTESIAN_POINT('Ctrl Pts',(84.8792584886388,23.5881052624922,-7.44473053389026));
#12603=CARTESIAN_POINT('Ctrl Pts',(84.5133590473266,21.7401488437674,-7.55586365188183));
#12604=CARTESIAN_POINT('Ctrl Pts',(82.7623737647797,21.0452588627609,-7.66699676987339));
#12605=CARTESIAN_POINT('Ctrl Pts',(81.2288734036351,22.139424370776,-7.77812988786495));
#12606=CARTESIAN_POINT('Ctrl Pts',(81.3163777952684,24.0212228361577,-7.8892630058565));
#12607=CARTESIAN_POINT('Ctrl Pts',(82.9447995049623,24.9683578317838,-8.00039612384807));
#12608=CARTESIAN_POINT('Ctrl Pts',(84.6237428755888,24.113974333724,-8.11152924183962));
#12609=CARTESIAN_POINT('Ctrl Pts',(84.8165728589842,22.2400376458565,-8.22266235983118));
#12610=CARTESIAN_POINT('Ctrl Pts',(83.3468038610209,21.061648433366,-8.33379547782274));
#12611=CARTESIAN_POINT('Ctrl Pts',(81.5596263199885,21.6573148588903,-8.4449285958143));
#12612=CARTESIAN_POINT('Ctrl Pts',(81.0907354631553,23.4818595774137,-8.55606171380585));
#12613=CARTESIAN_POINT('Ctrl Pts',(82.3692786585142,24.8653874427323,-8.66719483179742));
#12614=CARTESIAN_POINT('Ctrl Pts',(84.2250828504748,24.5416393006048,-8.77832794978898));
#12615=CARTESIAN_POINT('Ctrl Pts',(84.959642998928,22.8069221916923,-8.88946106778053));
#12616=CARTESIAN_POINT('Ctrl Pts',(83.9006607439461,21.2489174926821,-9.00059418577209));
#12617=CARTESIAN_POINT('Ctrl Pts',(82.0173583264533,21.2935724261695,-9.11172730376366));
#12618=CARTESIAN_POINT('Ctrl Pts',(81.0334082449847,22.9000170396293,-9.22286042175521));
#12619=CARTESIAN_POINT('Ctrl Pts',(81.8493603420058,24.5979699936773,-9.33399353974677));
#12620=CARTESIAN_POINT('Ctrl Pts',(83.7184231427578,24.8333979140429,-9.44512665773834));
#12621=CARTESIAN_POINT('Ctrl Pts',(84.9299568063988,23.3908279016291,-9.55625977572989));
#12622=CARTESIAN_POINT('Ctrl Pts',(84.375118038464,21.5905568108124,-9.66739289372145));
#12623=CARTESIAN_POINT('Ctrl Pts',(82.5617171176083,21.0802636018814,-9.77852601171301));
#12624=CARTESIAN_POINT('Ctrl Pts',(81.1494499413637,22.3269887045979,-9.88965912970457));
#12625=CARTESIAN_POINT('Ctrl Pts',(81.4308790157235,24.1896802343324,-10.0007922476961));
#12626=CARTESIAN_POINT('Ctrl Pts',(83.1484293748935,24.9635295882484,-10.1119253656877));
#12627=CARTESIAN_POINT('Ctrl Pts',(84.7301313280375,23.9402793792279,-10.2230584836792));
#12628=CARTESIAN_POINT('Ctrl Pts',(84.7283489924563,22.0564484733023,-10.3341916016708));
#12629=CARTESIAN_POINT('Ctrl Pts',(83.1447136318255,21.0361930624367,-10.4453247196624));
#12630=CARTESIAN_POINT('Ctrl Pts',(81.4286306594752,21.8132910555169,-10.5564578376539));
#12631=CARTESIAN_POINT('Ctrl Pts',(81.1507267560675,23.6765117829969,-10.6675909556455));
#12632=CARTESIAN_POINT('Ctrl Pts',(82.5653505121927,24.9205622994339,-10.778724073637));
#12633=CARTESIAN_POINT('Ctrl Pts',(84.3777825871961,24.4068386068335,-10.8898571916286));
#12634=CARTESIAN_POINT('Ctrl Pts',(84.9292138094035,22.6055208486311,-11.0009903096202));
#12635=CARTESIAN_POINT('Ctrl Pts',(83.7149526201293,21.1652459363096,-11.1121234276117));
#12636=CARTESIAN_POINT('Ctrl Pts',(81.8463386526518,21.4042101582938,-11.2232565456033));
#12637=CARTESIAN_POINT('Ctrl Pts',(81.0336009579355,23.1037040530836,-11.3343896635948));
#12638=CARTESIAN_POINT('Ctrl Pts',(82.0205890632288,24.7082839167396,-11.4455227815864));
#12639=CARTESIAN_POINT('Ctrl Pts',(83.9039726070939,24.7493751023956,-11.5566558995779));
#12640=CARTESIAN_POINT('Ctrl Pts',(84.9600048409316,23.1893693396062,-11.6677890175695));
#12641=CARTESIAN_POINT('Ctrl Pts',(84.2221634993099,21.4560453037046,-11.7789221355611));
#12642=CARTESIAN_POINT('Ctrl Pts',(82.3657500192332,21.1358093753172,-11.8900552535526));
#12643=CARTESIAN_POINT('Ctrl Pts',(81.0898270853904,22.5217540804675,-12.0011883715442));
#12644=CARTESIAN_POINT('Ctrl Pts',(81.5621695866715,24.3454082747499,-12.1123214895357));
#12645=CARTESIAN_POINT('Ctrl Pts',(83.3504710746846,24.9376918612276,-12.2234546075273));
#12646=CARTESIAN_POINT('Ctrl Pts',(84.8180076407391,23.7565235895013,-12.3345877255189));
#12647=CARTESIAN_POINT('Ctrl Pts',(84.621632057906,21.8829551521851,-12.4457208435104));
#12648=CARTESIAN_POINT('Ctrl Pts',(82.9410749888612,21.0317501260459,-12.556853961502));
#12649=CARTESIAN_POINT('Ctrl Pts',(81.3144484092768,21.9819648541096,-12.6679870794936));
#12650=CARTESIAN_POINT('Ctrl Pts',(81.2305049881862,23.8639254171651,-12.7791201974851));
#12651=CARTESIAN_POINT('Ctrl Pts',(82.7660730485526,24.955187434658,-12.8902533154767));
#12652=CARTESIAN_POINT('Ctrl Pts',(84.5157402621589,24.2569849565244,-13.0013864334682));
#12653=CARTESIAN_POINT('Ctrl Pts',(84.8781423288819,22.4083403717338,-13.1125195514598));
#12654=CARTESIAN_POINT('Ctrl Pts',(83.5215946132505,21.1012059662286,-13.2236526694514));
#12655=CARTESIAN_POINT('Ctrl Pts',(81.6876629778084,21.5319225962357,-13.3347857874429));
#12656=CARTESIAN_POINT('Ctrl Pts',(81.0548338381576,23.3062814491317,-13.4459189054345));
#12657=CARTESIAN_POINT('Ctrl Pts',(82.2022973308199,24.8003194646615,-13.557052023426));
#12658=CARTESIAN_POINT('Ctrl Pts',(84.079849703585,24.6466342462504,-13.6681851414176));
#12659=CARTESIAN_POINT('Ctrl Pts',(84.969081125163,22.9858845547767,-13.7793182594091));
#12660=CARTESIAN_POINT('Ctrl Pts',(84.056131998706,21.3380538743536,-13.8904513774007));
#12661=CARTESIAN_POINT('Ctrl Pts',(82.1765692980985,21.2113017016767,-14.0015844953923));
#12662=CARTESIAN_POINT('Ctrl Pts',(81.0506427857571,22.7216366141191,-14.1127176133838));
#12663=CARTESIAN_POINT('Ctrl Pts',(81.7088447219042,24.4867406535661,-14.2238507313754));
#12664=CARTESIAN_POINT('Ctrl Pts',(83.5487627878191,24.8911211293868,-14.3349838493669));
#12665=CARTESIAN_POINT('Ctrl Pts',(84.8864315514728,23.564673113672,-14.4461169673585));
#12666=CARTESIAN_POINT('Ctrl Pts',(84.4975639095097,21.7214140392435,-14.5572500853501));
#12667=CARTESIAN_POINT('Ctrl Pts',(82.7380668349932,21.0483671602815,-14.6683832033416));
#12668=CARTESIAN_POINT('Ctrl Pts',(81.2183013007427,22.161531472689,-14.7795163213332));
#12669=CARTESIAN_POINT('Ctrl Pts',(81.329216546894,24.0420951812183,-14.8906494393247));
#12670=CARTESIAN_POINT('Ctrl Pts',(82.9692985630169,24.9688923671652,-15.0017825573163));
#12671=CARTESIAN_POINT('Ctrl Pts',(84.6374797580343,24.0936817563847,-15.1129156753079));
#12672=CARTESIAN_POINT('Ctrl Pts',(84.806974997268,22.2174905701235,-15.2240487932994));
#12673=CARTESIAN_POINT('Ctrl Pts',(83.3226556582986,21.0574827837253,-15.335181911291));
#12674=CARTESIAN_POINT('Ctrl Pts',(81.5430290393143,21.6753432694906,-15.4463150292825));
#12675=CARTESIAN_POINT('Ctrl Pts',(81.0968798325604,23.5055816151367,-15.5574481472741));
#12676=CARTESIAN_POINT('Ctrl Pts',(82.3925406241014,24.8730920021767,-15.6685812652657));
#12677=CARTESIAN_POINT('Ctrl Pts',(84.2441731131724,24.526274395825,-15.7797143832572));
#12678=CARTESIAN_POINT('Ctrl Pts',(84.9570874696211,22.7825513238517,-15.8908475012488));
#12679=CARTESIAN_POINT('Ctrl Pts',(83.8788021914142,21.2378439741891,-16.0019806192403));
#12680=CARTESIAN_POINT('Ctrl Pts',(81.996194884314,21.3059348963008,-16.1131137372319));
#12681=CARTESIAN_POINT('Ctrl Pts',(81.0323248335547,22.9244934615319,-16.2242468552234));
#12682=CARTESIAN_POINT('Ctrl Pts',(81.8693180174765,24.6121733762817,-16.335379973215));
#12683=CARTESIAN_POINT('Ctrl Pts',(83.7412167335509,24.8242992580383,-16.4465130912066));
#12684=CARTESIAN_POINT('Ctrl Pts',(84.9346033040057,23.3668134991485,-16.5576462091981));
#12685=CARTESIAN_POINT('Ctrl Pts',(84.3576069455347,21.5734882290582,-16.6687793271897));
#12686=CARTESIAN_POINT('Ctrl Pts',(82.5375922462901,21.0859967419785,-16.7799124451812));
#12687=CARTESIAN_POINT('Ctrl Pts',(81.1417554914442,22.349809536703,-16.8910455631728));
#12688=CARTESIAN_POINT('Ctrl Pts',(81.4447236992157,24.2096334404004,-17.0021786811644));
#12689=CARTESIAN_POINT('Ctrl Pts',(83.1751260846232,24.9604903571868,-17.1133117991559));
#12690=CARTESIAN_POINT('Ctrl Pts',(84.2151340020225,24.2672324081111,-17.1874005444836));
#12691=CARTESIAN_POINT('Ctrl Pts',(84.4735782273626,23.7772536316049,-17.2244449171475));
#12692=CARTESIAN_POINT('Ctrl Pts',(84.3677806246588,24.1633123698098,-5.92518502761751));
#12693=CARTESIAN_POINT('Ctrl Pts',(84.7545930524416,23.7085123024942,-5.96222940028136));
#12694=CARTESIAN_POINT('Ctrl Pts',(85.0318746016131,22.3902512570299,-6.03631814560907));
#12695=CARTESIAN_POINT('Ctrl Pts',(83.5876743470062,20.9593799191348,-6.14745126360063));
#12696=CARTESIAN_POINT('Ctrl Pts',(81.6053425929765,21.4008969489394,-6.25858438159219));
#12697=CARTESIAN_POINT('Ctrl Pts',(80.8996137955093,23.3036683757581,-6.36971749958375));
#12698=CARTESIAN_POINT('Ctrl Pts',(82.1161600441146,24.9296622642438,-6.48085061757531));
#12699=CARTESIAN_POINT('Ctrl Pts',(84.1416722152917,24.7889762373743,-6.59198373556687));
#12700=CARTESIAN_POINT('Ctrl Pts',(85.1222605663254,23.011238051843,-6.70311685355843));
#12701=CARTESIAN_POINT('Ctrl Pts',(84.1604827817908,21.2230693022764,-6.81424997154998));
#12702=CARTESIAN_POINT('Ctrl Pts',(82.136580331694,21.0612901980477,-6.92538308954154));
#12703=CARTESIAN_POINT('Ctrl Pts',(80.9029161268739,22.6738581437696,-7.0365162075331));
#12704=CARTESIAN_POINT('Ctrl Pts',(81.5885843290494,24.5849422380838,-7.14764932552467));
#12705=CARTESIAN_POINT('Ctrl Pts',(83.5660363549255,25.0454156452787,-7.25878244351622));
#12706=CARTESIAN_POINT('Ctrl Pts',(85.0254293044568,23.6338487440436,-7.36991556150778));
#12707=CARTESIAN_POINT('Ctrl Pts',(84.6310697975563,21.6421562193206,-7.48104867949934));
#12708=CARTESIAN_POINT('Ctrl Pts',(82.7438909318581,20.8932169225645,-7.5921817974909));
#12709=CARTESIAN_POINT('Ctrl Pts',(81.091113206689,22.0724878409919,-7.70331491548246));
#12710=CARTESIAN_POINT('Ctrl Pts',(81.1854237872472,24.1006546844083,-7.81444803347401));
#12711=CARTESIAN_POINT('Ctrl Pts',(82.9405059490508,25.1214588936298,-7.92558115146558));
#12712=CARTESIAN_POINT('Ctrl Pts',(84.7500394027767,24.2006204966362,-8.03671426945713));
#12713=CARTESIAN_POINT('Ctrl Pts',(84.9578679167935,22.1809269285348,-8.14784738744869));
#12714=CARTESIAN_POINT('Ctrl Pts',(83.3737786511311,20.9108812922038,-8.25898050544026));
#12715=CARTESIAN_POINT('Ctrl Pts',(81.4475924528209,21.5528793149514,-8.37011362343181));
#12716=CARTESIAN_POINT('Ctrl Pts',(80.9422307435277,23.5193391513873,-8.48124674142336));
#12717=CARTESIAN_POINT('Ctrl Pts',(82.3202204509307,25.0104793531689,-8.59237985941493));
#12718=CARTESIAN_POINT('Ctrl Pts',(84.3203711574219,24.6615497203948,-8.70351297740649));
#12719=CARTESIAN_POINT('Ctrl Pts',(85.1120662113796,22.7919043849736,-8.81464609539804));
#12720=CARTESIAN_POINT('Ctrl Pts',(83.9707151385458,21.11271634728,-8.9257792133896));
#12721=CARTESIAN_POINT('Ctrl Pts',(81.94092736395,21.1608445911701,-9.03691233138117));
#12722=CARTESIAN_POINT('Ctrl Pts',(80.8804445505544,22.8922402537462,-9.14804544937273));
#12723=CARTESIAN_POINT('Ctrl Pts',(81.7598623093837,24.7222618774392,-9.25917856736428));
#12724=CARTESIAN_POINT('Ctrl Pts',(83.7743028940076,24.9760016433514,-9.37031168535585));
#12725=CARTESIAN_POINT('Ctrl Pts',(85.0800709937715,23.4212269305923,-9.4814448033474));
#12726=CARTESIAN_POINT('Ctrl Pts',(84.4820762492386,21.4809287516294,-9.59257792133897));
#12727=CARTESIAN_POINT('Ctrl Pts',(82.5276269874504,20.9309443692346,-9.70371103933052));
#12728=CARTESIAN_POINT('Ctrl Pts',(81.0055120991678,22.2746411373535,-9.81484415732209));
#12729=CARTESIAN_POINT('Ctrl Pts',(81.3088310400058,24.2822148864126,-9.92597727531363));
#12730=CARTESIAN_POINT('Ctrl Pts',(83.1599743767922,25.116255103941,-10.0371103933052));
#12731=CARTESIAN_POINT('Ctrl Pts',(84.8647028674081,24.0134153553533,-10.1482435112968));
#12732=CARTESIAN_POINT('Ctrl Pts',(84.8627818997827,21.9830579859066,-10.2593766292883));
#12733=CARTESIAN_POINT('Ctrl Pts',(83.1559696190948,20.8834459742058,-10.3705097472799));
#12734=CARTESIAN_POINT('Ctrl Pts',(81.3064078041073,21.7209875136666,-10.4816428652714));
#12735=CARTESIAN_POINT('Ctrl Pts',(81.0068882259397,23.7291316220605,-10.592775983263));
#12736=CARTESIAN_POINT('Ctrl Pts',(82.5315429915074,25.0699457716037,-10.7039091012546));
#12737=CARTESIAN_POINT('Ctrl Pts',(84.4849480495354,24.5162640787035,-10.8150422192461));
#12738=CARTESIAN_POINT('Ctrl Pts',(85.0792702056432,22.5748378214013,-10.9261753372377));
#12739=CARTESIAN_POINT('Ctrl Pts',(83.7705624302684,21.0225367241728,-11.0373084552292));
#12740=CARTESIAN_POINT('Ctrl Pts',(81.7566055896702,21.2800878491775,-11.1484415732208));
#12741=CARTESIAN_POINT('Ctrl Pts',(80.880652252933,23.1117702696975,-11.2595746912123));
#12742=CARTESIAN_POINT('Ctrl Pts',(81.944409391026,24.8411561401554,-11.3707078092039));
#12743=CARTESIAN_POINT('Ctrl Pts',(83.9742846020934,24.8854434439435,-11.4818409271955));
#12744=CARTESIAN_POINT('Ctrl Pts',(85.1124561978568,23.2040986975037,-11.592974045187));
#12745=CARTESIAN_POINT('Ctrl Pts',(84.3172247358758,21.3359547898621,-11.7041071631786));
#12746=CARTESIAN_POINT('Ctrl Pts',(82.3164173501609,20.9908105547198,-11.8152402811701));
#12747=CARTESIAN_POINT('Ctrl Pts',(80.9412517111298,22.484555580824,-11.9263733991617));
#12748=CARTESIAN_POINT('Ctrl Pts',(81.4503335376155,24.4500556270526,-12.0375065171532));
#12749=CARTESIAN_POINT('Ctrl Pts',(83.3777311047534,25.0884076897694,-12.1486396351448));
#12750=CARTESIAN_POINT('Ctrl Pts',(84.9594142974693,23.8153668358835,-12.2597727531364));
#12751=CARTESIAN_POINT('Ctrl Pts',(84.7477644033464,21.7960701612711,-12.3709058711279));
#12752=CARTESIAN_POINT('Ctrl Pts',(82.936491735944,20.8786574612801,-12.4820389891195));
#12753=CARTESIAN_POINT('Ctrl Pts',(81.1833443314669,21.9027809479542,-12.5931721071111));
#12754=CARTESIAN_POINT('Ctrl Pts',(81.0928716977014,23.9311224971817,-12.7043052251026));
#12755=CARTESIAN_POINT('Ctrl Pts',(82.7478779500382,25.1072640883641,-12.8154383430942));
#12756=CARTESIAN_POINT('Ctrl Pts',(84.6336362259272,24.3547546447695,-12.9265714610857));
#12757=CARTESIAN_POINT('Ctrl Pts',(85.0242263285524,22.3623204276585,-13.0377045790773));
#12758=CARTESIAN_POINT('Ctrl Pts',(83.5621648225144,20.953515653978,-13.1488376970689));
#12759=CARTESIAN_POINT('Ctrl Pts',(81.5855879443197,21.4177339026156,-13.2599708150604));
#12760=CARTESIAN_POINT('Ctrl Pts',(80.903536650199,23.3301043609664,-13.371103933052));
#12761=CARTESIAN_POINT('Ctrl Pts',(82.1402511298108,24.9403503153792,-13.4822370510435));
#12762=CARTESIAN_POINT('Ctrl Pts',(84.1638416148031,24.7747112897138,-13.5933701690351));
#12763=CARTESIAN_POINT('Ctrl Pts',(85.1222384455726,22.9847866397446,-13.7045032870266));
#12764=CARTESIAN_POINT('Ctrl Pts',(84.1382791204541,21.2087858558772,-13.8156364050182));
#12765=CARTESIAN_POINT('Ctrl Pts',(82.1125219420832,21.0721747582047,-13.9267695230098));
#12766=CARTESIAN_POINT('Ctrl Pts',(80.8990196130806,22.6999852003014,-14.0379026410013));
#12767=CARTESIAN_POINT('Ctrl Pts',(81.6084172280349,24.6023809955177,-14.1490357589929));
#12768=CARTESIAN_POINT('Ctrl Pts',(83.5914461679238,25.0382146345988,-14.2601688769844));
#12769=CARTESIAN_POINT('Ctrl Pts',(85.0331602960979,23.6085940166212,-14.371301994976));
#12770=CARTESIAN_POINT('Ctrl Pts',(84.6140460963486,21.6219642008593,-14.4824351129676));
#12771=CARTESIAN_POINT('Ctrl Pts',(82.7176933820329,20.896566986924,-14.5935682309591));
#12772=CARTESIAN_POINT('Ctrl Pts',(81.0797187938726,22.0963144578846,-14.7047013489507));
#12773=CARTESIAN_POINT('Ctrl Pts',(81.1992611512568,24.123150503687,-14.8158344669422));
#12774=CARTESIAN_POINT('Ctrl Pts',(82.9669105710946,25.1220350057677,-14.9269675849338));
#12775=CARTESIAN_POINT('Ctrl Pts',(84.7648447552206,24.1787495400571,-15.0381007029254));
#12776=CARTESIAN_POINT('Ctrl Pts',(84.9475235227155,22.156626116169,-15.1492338209169));
#12777=CARTESIAN_POINT('Ctrl Pts',(83.3477521743381,20.9063916337,-15.2603669389085));
#12778=CARTESIAN_POINT('Ctrl Pts',(81.4297042171919,21.5723099953839,-15.3715000569));
#12779=CARTESIAN_POINT('Ctrl Pts',(80.9488530288205,23.5449063155938,-15.4826331748916));
#12780=CARTESIAN_POINT('Ctrl Pts',(82.3452917580788,25.0187831818178,-15.5937662928831));
#12781=CARTESIAN_POINT('Ctrl Pts',(84.340946281989,24.6449897162286,-15.7048994108747));
#12782=CARTESIAN_POINT('Ctrl Pts',(85.1093119101604,22.7656379239212,-15.8160325288663));
#12783=CARTESIAN_POINT('Ctrl Pts',(83.9471564034816,21.1007815181999,-15.9271656468578));
#12784=CARTESIAN_POINT('Ctrl Pts',(81.9181178057378,21.1741686279808,-16.0382987648494));
#12785=CARTESIAN_POINT('Ctrl Pts',(80.8792768701784,22.9186204789729,-16.149431882841));
#12786=CARTESIAN_POINT('Ctrl Pts',(81.7813723150542,24.7375700149431,-16.2605650008325));
#12787=CARTESIAN_POINT('Ctrl Pts',(83.7988693956495,24.966195283761,-16.3716981188241));
#12788=CARTESIAN_POINT('Ctrl Pts',(85.0850789011309,23.3953446611721,-16.4828312368156));
#12789=CARTESIAN_POINT('Ctrl Pts',(84.4632031240215,21.4625325565985,-16.5939643548072));
#12790=CARTESIAN_POINT('Ctrl Pts',(82.5016256568034,20.9371234393463,-16.7050974727987));
#12791=CARTESIAN_POINT('Ctrl Pts',(80.9972191663739,22.2992369991667,-16.8162305907903));
#12792=CARTESIAN_POINT('Ctrl Pts',(81.3237525783814,24.3037200750453,-16.9273637087819));
#12793=CARTESIAN_POINT('Ctrl Pts',(83.1887475863033,25.1129794781064,-17.0384968267734));
#12794=CARTESIAN_POINT('Ctrl Pts',(84.3096484764695,24.3657991545403,-17.1125855721011));
#12795=CARTESIAN_POINT('Ctrl Pts',(84.5881947811615,23.837709283723,-17.149629944765));
#12796=CARTESIAN_POINT('Ctrl Pts',(84.4664903694652,24.247266086571,-5.85037005523502));
#12797=CARTESIAN_POINT('Ctrl Pts',(84.8812182065951,23.7596440902316,-5.88741442789887));
#12798=CARTESIAN_POINT('Ctrl Pts',(85.1785105604709,22.3462470199983,-5.96150317322658));
#12799=CARTESIAN_POINT('Ctrl Pts',(83.6300855230211,20.8121128181116,-6.07263629121815));
#12800=CARTESIAN_POINT('Ctrl Pts',(81.5046932094001,21.2854931690907,-6.18376940920969));
#12801=CARTESIAN_POINT('Ctrl Pts',(80.7480335036829,23.3255834601923,-6.29490252720126));
#12802=CARTESIAN_POINT('Ctrl Pts',(82.052375241989,25.0689217816197,-6.40603564519281));
#12803=CARTESIAN_POINT('Ctrl Pts',(84.2240642092945,24.9180827510011,-6.51716876318438));
#12804=CARTESIAN_POINT('Ctrl Pts',(85.2754194831416,23.0120490775365,-6.62830188117593));
#12805=CARTESIAN_POINT('Ctrl Pts',(84.2442322933555,21.0948320889771,-6.73943499916749));
#12806=CARTESIAN_POINT('Ctrl Pts',(82.0742692171901,20.9213777396063,-6.85056811715905));
#12807=CARTESIAN_POINT('Ctrl Pts',(80.7515741571003,22.6503211972602,-6.96170123515061));
#12808=CARTESIAN_POINT('Ctrl Pts',(81.4867255381121,24.699324062942,-7.07283435314218));
#12809=CARTESIAN_POINT('Ctrl Pts',(83.6068859642405,25.1930288317273,-7.18396747113373));
#12810=CARTESIAN_POINT('Ctrl Pts',(85.1716001202748,23.6795922255951,-7.29510058912529));
#12811=CARTESIAN_POINT('Ctrl Pts',(84.748780547786,21.5441635948737,-7.40623370711685));
#12812=CARTESIAN_POINT('Ctrl Pts',(82.7254080989366,20.7411749823681,-7.51736682510841));
#12813=CARTESIAN_POINT('Ctrl Pts',(80.9533530097428,22.0055513112078,-7.62849994309997));
#12814=CARTESIAN_POINT('Ctrl Pts',(81.0544697792261,24.1800865326589,-7.73963306109152));
#12815=CARTESIAN_POINT('Ctrl Pts',(82.9362123931393,25.2745599554757,-7.85076617908309));
#12816=CARTESIAN_POINT('Ctrl Pts',(84.8763359299646,24.2872666595484,-7.96189929707464));
#12817=CARTESIAN_POINT('Ctrl Pts',(85.0991629746026,22.1218162112133,-8.0730324150662));
#12818=CARTESIAN_POINT('Ctrl Pts',(83.4007534412416,20.7601141510415,-8.18416553305776));
#12819=CARTESIAN_POINT('Ctrl Pts',(81.3355585856531,21.4484437710125,-8.29529865104933));
#12820=CARTESIAN_POINT('Ctrl Pts',(80.7937260239002,23.5568187253608,-8.40643176904088));
#12821=CARTESIAN_POINT('Ctrl Pts',(82.2711622433471,25.1555712636055,-8.51756488703244));
#12822=CARTESIAN_POINT('Ctrl Pts',(84.4156594643692,24.7814601401847,-8.628698005024));
#12823=CARTESIAN_POINT('Ctrl Pts',(85.2644894238312,22.776886578255,-8.73983112301556));
#12824=CARTESIAN_POINT('Ctrl Pts',(84.0407695331455,20.9765152018779,-8.85096424100711));
#12825=CARTESIAN_POINT('Ctrl Pts',(81.8644964014467,21.0281167561708,-8.96209735899868));
#12826=CARTESIAN_POINT('Ctrl Pts',(80.7274808561243,22.884463467863,-9.07323047699024));
#12827=CARTESIAN_POINT('Ctrl Pts',(81.6703642767617,24.8465537612011,-9.18436359498179));
#12828=CARTESIAN_POINT('Ctrl Pts',(83.8301826452576,25.11860537266,-9.29549671297336));
#12829=CARTESIAN_POINT('Ctrl Pts',(85.2301851811438,23.4516259595556,-9.40662983096491));
#12830=CARTESIAN_POINT('Ctrl Pts',(84.5890344600137,21.3713006924463,-9.51776294895647));
#12831=CARTESIAN_POINT('Ctrl Pts',(82.4935368572922,20.7816251365878,-9.62889606694804));
#12832=CARTESIAN_POINT('Ctrl Pts',(80.861574256972,22.2222935701091,-9.74002918493958));
#12833=CARTESIAN_POINT('Ctrl Pts',(81.1867830642879,24.3747495384927,-9.85116230293116));
#12834=CARTESIAN_POINT('Ctrl Pts',(83.171519378691,25.2689806196336,-9.96229542092269));
#12835=CARTESIAN_POINT('Ctrl Pts',(84.9992744067787,24.0865513314787,-10.0734285389143));
#12836=CARTESIAN_POINT('Ctrl Pts',(84.9972148071091,21.9096674985109,-10.1845616569058));
#12837=CARTESIAN_POINT('Ctrl Pts',(83.1672256063643,20.730698885975,-10.2956947748974));
#12838=CARTESIAN_POINT('Ctrl Pts',(81.1841849487392,21.6286839718163,-10.4068278928889));
#12839=CARTESIAN_POINT('Ctrl Pts',(80.863049695812,23.7817514611242,-10.5179610108805));
#12840=CARTESIAN_POINT('Ctrl Pts',(82.497735470822,25.2193292437736,-10.6290941288721));
#12841=CARTESIAN_POINT('Ctrl Pts',(84.5921135118751,24.6256895505736,-10.7402272468636));
#12842=CARTESIAN_POINT('Ctrl Pts',(85.2293266018828,22.5441547941715,-10.8513603648552));
#12843=CARTESIAN_POINT('Ctrl Pts',(83.8261722404075,20.879827512036,-10.9624934828467));
#12844=CARTESIAN_POINT('Ctrl Pts',(81.6668725266888,21.1559655400612,-11.0736266008383));
#12845=CARTESIAN_POINT('Ctrl Pts',(80.7277035479304,23.1198364863114,-11.1847597188298));
#12846=CARTESIAN_POINT('Ctrl Pts',(81.8682297188232,24.9740283635713,-11.2958928368214));
#12847=CARTESIAN_POINT('Ctrl Pts',(84.044596597093,25.0215117854914,-11.407025954813));
#12848=CARTESIAN_POINT('Ctrl Pts',(85.2649075547819,23.2188280554013,-11.5181590728046));
#12849=CARTESIAN_POINT('Ctrl Pts',(84.4122859724418,21.2158642760196,-11.6292921907961));
#12850=CARTESIAN_POINT('Ctrl Pts',(82.2670846810887,20.8458117341225,-11.7404253087877));
#12851=CARTESIAN_POINT('Ctrl Pts',(80.7926763368691,22.4473570811805,-11.8515584267792));
#12852=CARTESIAN_POINT('Ctrl Pts',(81.3384974885596,24.5547029793554,-11.9626915447708));
#12853=CARTESIAN_POINT('Ctrl Pts',(83.4049911348221,25.2391235183113,-12.0738246627623));
#12854=CARTESIAN_POINT('Ctrl Pts',(85.1008209541995,23.8742100822658,-12.1849577807539));
#12855=CARTESIAN_POINT('Ctrl Pts',(84.8738967487866,21.7091851703571,-12.2960908987455));
#12856=CARTESIAN_POINT('Ctrl Pts',(82.9319084830269,20.7255647965142,-12.407224016737));
#12857=CARTESIAN_POINT('Ctrl Pts',(81.052240253657,21.8235970417987,-12.5183571347286));
#12858=CARTESIAN_POINT('Ctrl Pts',(80.9552384072167,23.9983195771983,-12.6294902527201));
#12859=CARTESIAN_POINT('Ctrl Pts',(82.7296828515237,25.2593407420703,-12.7406233707117));
#12860=CARTESIAN_POINT('Ctrl Pts',(84.7515321896956,24.4525243330146,-12.8517564887033));
#12861=CARTESIAN_POINT('Ctrl Pts',(85.1703103282228,22.3163004835832,-12.9628896066948));
#12862=CARTESIAN_POINT('Ctrl Pts',(83.6027350317784,20.8058253417273,-13.0740227246864));
#12863=CARTESIAN_POINT('Ctrl Pts',(81.4835129108309,21.3035452089955,-13.1851558426779));
#12864=CARTESIAN_POINT('Ctrl Pts',(80.7522394622406,23.3539272728011,-13.2962889606695));
#12865=CARTESIAN_POINT('Ctrl Pts',(82.0782049288016,25.080381166097,-13.407422078661));
#12866=CARTESIAN_POINT('Ctrl Pts',(84.2478335260214,24.9027883331771,-13.5185551966526));
#12867=CARTESIAN_POINT('Ctrl Pts',(85.2753957659822,22.9836887247125,-13.6296883146442));
#12868=CARTESIAN_POINT('Ctrl Pts',(84.2204262422021,21.0795178374008,-13.7408214326357));
#12869=CARTESIAN_POINT('Ctrl Pts',(82.0484745860681,20.9330478147326,-13.8519545506273));
#12870=CARTESIAN_POINT('Ctrl Pts',(80.7473964404041,22.6783337864837,-13.9630876686188));
#12871=CARTESIAN_POINT('Ctrl Pts',(81.5079897341654,24.7180213374692,-14.0742207866104));
#12872=CARTESIAN_POINT('Ctrl Pts',(83.6341295480289,25.1853081398107,-14.185353904602));
#12873=CARTESIAN_POINT('Ctrl Pts',(85.1798890407227,23.6525149195704,-14.2964870225935));
#12874=CARTESIAN_POINT('Ctrl Pts',(84.7305282831878,21.5225143624751,-14.4076201405851));
#12875=CARTESIAN_POINT('Ctrl Pts',(82.6973199290724,20.7447668135665,-14.5187532585766));
#12876=CARTESIAN_POINT('Ctrl Pts',(80.9411362870026,22.0310974430802,-14.6298863765682));
#12877=CARTESIAN_POINT('Ctrl Pts',(81.0693057556195,24.2042058261558,-14.7410194945597));
#12878=CARTESIAN_POINT('Ctrl Pts',(82.9645225791725,25.2751776443702,-14.8521526125513));
#12879=CARTESIAN_POINT('Ctrl Pts',(84.8922097524064,24.2638173237295,-14.9632857305429));
#12880=CARTESIAN_POINT('Ctrl Pts',(85.0880720481635,22.0957616622145,-15.0744188485344));
#12881=CARTESIAN_POINT('Ctrl Pts',(83.372848690377,20.7553004836746,-15.185551966526));
#12882=CARTESIAN_POINT('Ctrl Pts',(81.3163793950698,21.4692767212771,-15.2966850845175));
#12883=CARTESIAN_POINT('Ctrl Pts',(80.8008262250806,23.5842310160509,-15.4078182025091));
#12884=CARTESIAN_POINT('Ctrl Pts',(82.2980428920563,25.1644743614589,-15.5189513205007));
#12885=CARTESIAN_POINT('Ctrl Pts',(84.4377194508057,24.7637050366322,-15.6300844384922));
#12886=CARTESIAN_POINT('Ctrl Pts',(85.2615363506997,22.7487245239907,-15.7412175564838));
#12887=CARTESIAN_POINT('Ctrl Pts',(84.0155106155488,20.9637190622108,-15.8523506744753));
#12888=CARTESIAN_POINT('Ctrl Pts',(81.8400407271619,21.0424023596608,-15.9634837924669));
#12889=CARTESIAN_POINT('Ctrl Pts',(80.7262289068018,22.9127474964141,-16.0746169104585));
#12890=CARTESIAN_POINT('Ctrl Pts',(81.6934266126323,24.8629666536045,-16.18575002845));
#12891=CARTESIAN_POINT('Ctrl Pts',(83.8565220577477,25.1080913094838,-16.2968831464416));
#12892=CARTESIAN_POINT('Ctrl Pts',(85.2355544982563,23.4238758231957,-16.4080162644331));
#12893=CARTESIAN_POINT('Ctrl Pts',(84.5687993025081,21.3515768841388,-16.5191493824247));
#12894=CARTESIAN_POINT('Ctrl Pts',(82.4656590673167,20.7882501367141,-16.6302825004163));
#12895=CARTESIAN_POINT('Ctrl Pts',(80.8526828413037,22.2486644616303,-16.7414156184078));
#12896=CARTESIAN_POINT('Ctrl Pts',(81.2027814575469,24.3978067096903,-16.8525487363994));
#12897=CARTESIAN_POINT('Ctrl Pts',(83.2023690879836,25.2654685990261,-16.9636818543909));
#12898=CARTESIAN_POINT('Ctrl Pts',(84.4041629509165,24.4643659009695,-17.0377705997186));
#12899=CARTESIAN_POINT('Ctrl Pts',(84.7028113349605,23.8981649358411,-17.0748149723825));
#12900=CARTESIAN_POINT('Ctrl Pts',(84.5652001142717,24.3312198033322,-5.77555508285253));
#12901=CARTESIAN_POINT('Ctrl Pts',(85.0078433607487,23.8107758779691,-5.81259945551639));
#12902=CARTESIAN_POINT('Ctrl Pts',(85.3251465193287,22.3022427829668,-5.88668820084409));
#12903=CARTESIAN_POINT('Ctrl Pts',(83.6724966990361,20.6648457170885,-5.99782131883566));
#12904=CARTESIAN_POINT('Ctrl Pts',(81.4040438258236,21.170089389242,-6.1089544368272));
#12905=CARTESIAN_POINT('Ctrl Pts',(80.5964532118565,23.3474985446265,-6.22008755481878));
#12906=CARTESIAN_POINT('Ctrl Pts',(81.9885904398633,25.2081812989956,-6.33122067281032));
#12907=CARTESIAN_POINT('Ctrl Pts',(84.3064562032972,25.0471892646279,-6.44235379080189));
#12908=CARTESIAN_POINT('Ctrl Pts',(85.4285783999577,23.0128601032299,-6.55348690879345));
#12909=CARTESIAN_POINT('Ctrl Pts',(84.3279818049202,20.9665948756778,-6.664620026785));
#12910=CARTESIAN_POINT('Ctrl Pts',(82.0119581026862,20.781465281165,-6.77575314477657));
#12911=CARTESIAN_POINT('Ctrl Pts',(80.6002321873268,22.6267842507508,-6.88688626276812));
#12912=CARTESIAN_POINT('Ctrl Pts',(81.3848667471746,24.8137058878003,-6.99801938075968));
#12913=CARTESIAN_POINT('Ctrl Pts',(83.6477355735556,25.340642018176,-7.10915249875124));
#12914=CARTESIAN_POINT('Ctrl Pts',(85.3177709360927,23.7253357071464,-7.2202856167428));
#12915=CARTESIAN_POINT('Ctrl Pts',(84.8664912980158,21.4461709704268,-7.33141873473436));
#12916=CARTESIAN_POINT('Ctrl Pts',(82.706925266015,20.5891330421716,-7.44255185272592));
#12917=CARTESIAN_POINT('Ctrl Pts',(80.8155928127967,21.9386147814237,-7.55368497071748));
#12918=CARTESIAN_POINT('Ctrl Pts',(80.923515771205,24.2595183809094,-7.66481808870904));
#12919=CARTESIAN_POINT('Ctrl Pts',(82.9319188372278,25.4276610173216,-7.7759512067006));
#12920=CARTESIAN_POINT('Ctrl Pts',(85.0026324571524,24.3739128224606,-7.88708432469215));
#12921=CARTESIAN_POINT('Ctrl Pts',(85.2404580324118,22.0627054938917,-7.99821744268371));
#12922=CARTESIAN_POINT('Ctrl Pts',(83.427728231352,20.6093470098792,-8.10935056067528));
#12923=CARTESIAN_POINT('Ctrl Pts',(81.2235247184853,21.3440082270736,-8.22048367866683));
#12924=CARTESIAN_POINT('Ctrl Pts',(80.6452213042727,23.5942982993343,-8.33161679665839));
#12925=CARTESIAN_POINT('Ctrl Pts',(82.2221040357635,25.3006631740422,-8.44274991464995));
#12926=CARTESIAN_POINT('Ctrl Pts',(84.5109477713164,24.9013705599747,-8.55388303264151));
#12927=CARTESIAN_POINT('Ctrl Pts',(85.4169126362828,22.7618687715364,-8.66501615063307));
#12928=CARTESIAN_POINT('Ctrl Pts',(84.1108239277452,20.8403140564757,-8.77614926862462));
#12929=CARTESIAN_POINT('Ctrl Pts',(81.7880654389434,20.8953889211715,-8.88728238661619));
#12930=CARTESIAN_POINT('Ctrl Pts',(80.574517161694,22.8766866819798,-8.99841550460775));
#12931=CARTESIAN_POINT('Ctrl Pts',(81.5808662441396,24.9708456449631,-9.10954862259931));
#12932=CARTESIAN_POINT('Ctrl Pts',(83.8860623965075,25.2612091019686,-9.22068174059087));
#12933=CARTESIAN_POINT('Ctrl Pts',(85.3802993685163,23.4820249885188,-9.33181485858242));
#12934=CARTESIAN_POINT('Ctrl Pts',(84.6959926707885,21.2616726332633,-9.44294797657398));
#12935=CARTESIAN_POINT('Ctrl Pts',(82.4594467271343,20.632305903941,-9.55408109456555));
#12936=CARTESIAN_POINT('Ctrl Pts',(80.7176364147761,22.1699460028647,-9.66521421255709));
#12937=CARTESIAN_POINT('Ctrl Pts',(81.0647350885701,24.4672841905729,-9.77634733054866));
#12938=CARTESIAN_POINT('Ctrl Pts',(83.1830643805896,25.4217061353262,-9.88748044854022));
#12939=CARTESIAN_POINT('Ctrl Pts',(85.1338459461496,24.1596873076041,-9.99861356653177));
#12940=CARTESIAN_POINT('Ctrl Pts',(85.1316477144354,21.8362770111152,-10.1097466845233));
#12941=CARTESIAN_POINT('Ctrl Pts',(83.1784815936336,20.5779517977441,-10.2208798025149));
#12942=CARTESIAN_POINT('Ctrl Pts',(81.0619620933712,21.536380429966,-10.3320129205065));
#12943=CARTESIAN_POINT('Ctrl Pts',(80.7192111656842,23.8343713001878,-10.443146038498));
#12944=CARTESIAN_POINT('Ctrl Pts',(82.4639279501368,25.3687127159435,-10.5542791564896));
#12945=CARTESIAN_POINT('Ctrl Pts',(84.6992789742144,24.7351150224436,-10.6654122744811));
#12946=CARTESIAN_POINT('Ctrl Pts',(85.3793829981224,22.5134717669416,-10.7765453924727));
#12947=CARTESIAN_POINT('Ctrl Pts',(83.8817820505465,20.7371182998993,-10.8876785104642));
#12948=CARTESIAN_POINT('Ctrl Pts',(81.5771394637072,21.0318432309449,-10.9988116284558));
#12949=CARTESIAN_POINT('Ctrl Pts',(80.574754842928,23.1279027029253,-11.1099447464474));
#12950=CARTESIAN_POINT('Ctrl Pts',(81.7920500466204,25.1069005869871,-11.2210778644389));
#12951=CARTESIAN_POINT('Ctrl Pts',(84.1149085920925,25.1575801270393,-11.3322109824305));
#12952=CARTESIAN_POINT('Ctrl Pts',(85.4173589117072,23.2335574132988,-11.4433441004221));
#12953=CARTESIAN_POINT('Ctrl Pts',(84.5073472090078,21.0957737621771,-11.5544772184136));
#12954=CARTESIAN_POINT('Ctrl Pts',(82.2177520120164,20.7008129135252,-11.6656103364052));
#12955=CARTESIAN_POINT('Ctrl Pts',(80.6441009626085,22.410158581537,-11.7767434543967));
#12956=CARTESIAN_POINT('Ctrl Pts',(81.2266614395036,24.6593503316581,-11.8878765723883));
#12957=CARTESIAN_POINT('Ctrl Pts',(83.4322511648908,25.3898393468531,-11.9990096903799));
#12958=CARTESIAN_POINT('Ctrl Pts',(85.2422276109297,23.9330533286481,-12.1101428083714));
#12959=CARTESIAN_POINT('Ctrl Pts',(85.000029094227,21.6223001794432,-12.221275926363));
#12960=CARTESIAN_POINT('Ctrl Pts',(82.9273252301097,20.5724721317484,-12.3324090443545));
#12961=CARTESIAN_POINT('Ctrl Pts',(80.9211361758472,21.7444131356433,-12.4435421623461));
#12962=CARTESIAN_POINT('Ctrl Pts',(80.8176051167319,24.0655166572149,-12.5546752803376));
#12963=CARTESIAN_POINT('Ctrl Pts',(82.7114877530095,25.4114173957764,-12.6658083983292));
#12964=CARTESIAN_POINT('Ctrl Pts',(84.8694281534639,24.5502940212596,-12.7769415163208));
#12965=CARTESIAN_POINT('Ctrl Pts',(85.3163943278932,22.2702805395079,-12.8880746343123));
#12966=CARTESIAN_POINT('Ctrl Pts',(83.6433052410424,20.6581350294767,-12.9992077523039));
#12967=CARTESIAN_POINT('Ctrl Pts',(81.381437877342,21.1893565153754,-13.1103408702954));
#12968=CARTESIAN_POINT('Ctrl Pts',(80.6009422742822,23.3777501846358,-13.221473988287));
#12969=CARTESIAN_POINT('Ctrl Pts',(82.0161587277924,25.2204120168147,-13.3326071062785));
#12970=CARTESIAN_POINT('Ctrl Pts',(84.3318254372397,25.0308653766405,-13.4437402242701));
#12971=CARTESIAN_POINT('Ctrl Pts',(85.4285530863916,22.9825908096803,-13.5548733422617));
#12972=CARTESIAN_POINT('Ctrl Pts',(84.3025733639503,20.9502498189244,-13.6660064602532));
#12973=CARTESIAN_POINT('Ctrl Pts',(81.9844272300528,20.7939208712606,-13.7771395782448));
#12974=CARTESIAN_POINT('Ctrl Pts',(80.5957732677276,22.6566823726659,-13.8882726962363));
#12975=CARTESIAN_POINT('Ctrl Pts',(81.407562240296,24.8336616794208,-13.9994058142279));
#12976=CARTESIAN_POINT('Ctrl Pts',(83.6768129281338,25.3324016450226,-14.1105389322195));
#12977=CARTESIAN_POINT('Ctrl Pts',(85.3266177853476,23.6964358225195,-14.221672050211));
#12978=CARTESIAN_POINT('Ctrl Pts',(84.8470104700268,21.423064524091,-14.3328051682026));
#12979=CARTESIAN_POINT('Ctrl Pts',(82.676946476112,20.5929666402091,-14.4439382861941));
#12980=CARTESIAN_POINT('Ctrl Pts',(80.8025537801326,21.9658804282759,-14.5550714041857));
#12981=CARTESIAN_POINT('Ctrl Pts',(80.9393503599823,24.2852611486245,-14.6662045221773));
#12982=CARTESIAN_POINT('Ctrl Pts',(82.9621345872503,25.4283202829728,-14.7773376401688));
#12983=CARTESIAN_POINT('Ctrl Pts',(85.0195747495924,24.3488851074018,-14.8884707581604));
#12984=CARTESIAN_POINT('Ctrl Pts',(85.2286205736113,22.0348972082601,-14.9996038761519));
#12985=CARTESIAN_POINT('Ctrl Pts',(83.3979452064162,20.6042093336492,-15.1107369941435));
#12986=CARTESIAN_POINT('Ctrl Pts',(81.2030545729478,21.3662434471704,-15.221870112135));
#12987=CARTESIAN_POINT('Ctrl Pts',(80.6527994213405,23.6235557165079,-15.3330032301266));
#12988=CARTESIAN_POINT('Ctrl Pts',(82.2507940260338,25.3101655411,-15.4441363481181));
#12989=CARTESIAN_POINT('Ctrl Pts',(84.5344926196224,24.8824203570357,-15.5552694661097));
#12990=CARTESIAN_POINT('Ctrl Pts',(85.4137607912389,22.7318111240602,-15.6664025841013));
#12991=CARTESIAN_POINT('Ctrl Pts',(84.0838648276161,20.8266566062216,-15.7775357020929));
#12992=CARTESIAN_POINT('Ctrl Pts',(81.7619636485858,20.9106360913409,-15.8886688200844));
#12993=CARTESIAN_POINT('Ctrl Pts',(80.5731809434253,22.9068745138551,-15.999801938076));
#12994=CARTESIAN_POINT('Ctrl Pts',(81.60548091021,24.9883632922658,-16.1109350560675));
#12995=CARTESIAN_POINT('Ctrl Pts',(83.9141747198462,25.2499873352066,-16.2220681740591));
#12996=CARTESIAN_POINT('Ctrl Pts',(85.3860300953815,23.4524069852193,-16.3332012920506));
#12997=CARTESIAN_POINT('Ctrl Pts',(84.6743954809949,21.240621211679,-16.4443344100422));
#12998=CARTESIAN_POINT('Ctrl Pts',(82.4296924778299,20.6393768340819,-16.5554675280338));
#12999=CARTESIAN_POINT('Ctrl Pts',(80.7081465162334,22.1980919240939,-16.6666006460253));
#13000=CARTESIAN_POINT('Ctrl Pts',(81.0818103367127,24.4918933443353,-16.7777337640169));
#13001=CARTESIAN_POINT('Ctrl Pts',(83.2159905896636,25.4179577199457,-16.8888668820084));
#13002=CARTESIAN_POINT('Ctrl Pts',(84.4986774253636,24.5629326473987,-16.9629556273361));
#13003=CARTESIAN_POINT('Ctrl Pts',(84.8174278887595,23.9586205879593,-17.));
#13004=CARTESIAN_POINT('Ctrl Pts',(84.2690708798524,24.0793586530485,-6.));
#13005=CARTESIAN_POINT('Ctrl Pts',(84.31440001981,24.0370713763938,-6.));
#13006=CARTESIAN_POINT('Ctrl Pts',(84.3569991508135,23.9922149796692,-6.));
#13007=CARTESIAN_POINT('Ctrl Pts',(84.3968697551056,23.9451344884964,-6.));
#13008=CARTESIAN_POINT('Ctrl Pts',(84.4393720233826,23.8949464438965,-6.));
#13009=CARTESIAN_POINT('Ctrl Pts',(84.478774408848,23.8422307785529,-6.));
#13010=CARTESIAN_POINT('Ctrl Pts',(84.5150498742739,23.7873507314227,-6.));
#13011=CARTESIAN_POINT('Ctrl Pts',(84.5467909065216,23.7393306901838,-6.));
#13012=CARTESIAN_POINT('Ctrl Pts',(84.5761376471904,23.6896523185269,-6.));
#13013=CARTESIAN_POINT('Ctrl Pts',(84.6030490903269,23.6385314038462,-6.));
#13014=CARTESIAN_POINT('Ctrl Pts',(84.6165493141079,23.6128864102062,-6.));
#13015=CARTESIAN_POINT('Ctrl Pts',(84.6294363190557,23.5868780356607,-6.));
#13016=CARTESIAN_POINT('Ctrl Pts',(84.6417025870925,23.5605316810879,-6.));
#13017=CARTESIAN_POINT('Ctrl Pts',(84.647311574959,23.5484843018295,-6.));
#13018=CARTESIAN_POINT('Ctrl Pts',(84.652791347877,23.5363645681783,-6.));
#13019=CARTESIAN_POINT('Ctrl Pts',(84.6581326742843,23.5241948681676,-6.));
#13020=CARTESIAN_POINT('Ctrl Pts',(84.6850515361933,23.4628628227009,-6.));
#13021=CARTESIAN_POINT('Ctrl Pts',(84.7085092386931,23.400155314048,-6.));
#13022=CARTESIAN_POINT('Ctrl Pts',(84.7284822796849,23.3364301112262,-6.));
#13023=CARTESIAN_POINT('Ctrl Pts',(84.7488096464292,23.2715744105277,-6.));
#13024=CARTESIAN_POINT('Ctrl Pts',(84.7655281752392,23.2056637457477,-6.));
#13025=CARTESIAN_POINT('Ctrl Pts',(84.7785737746937,23.139038753957,-6.));
#13026=CARTESIAN_POINT('Ctrl Pts',(84.7894849804243,23.083314293401,-6.));
#13027=CARTESIAN_POINT('Ctrl Pts',(84.7978262414115,23.0270891857862,-6.));
#13028=CARTESIAN_POINT('Ctrl Pts',(84.8035352337538,22.9705504503036,-6.));
#13029=CARTESIAN_POINT('Ctrl Pts',(84.8061648366007,22.9445083029563,-6.));
#13030=CARTESIAN_POINT('Ctrl Pts',(84.8082356449419,22.9183995035543,-6.));
#13031=CARTESIAN_POINT('Ctrl Pts',(84.8097397666649,22.8922419268446,-6.));
#13032=CARTESIAN_POINT('Ctrl Pts',(84.8103971308092,22.8808099710605,-6.));
#13033=CARTESIAN_POINT('Ctrl Pts',(84.8109461375351,22.8693689032805,-6.));
#13034=CARTESIAN_POINT('Ctrl Pts',(84.8113857933626,22.8579343510023,-6.));
#13035=CARTESIAN_POINT('Ctrl Pts',(84.8140821318782,22.7878080799712,-6.));
#13036=CARTESIAN_POINT('Ctrl Pts',(84.8126777401308,22.7177955074969,-6.));
#13037=CARTESIAN_POINT('Ctrl Pts',(84.8071179912164,22.6482574382939,-6.));
#13038=CARTESIAN_POINT('Ctrl Pts',(84.8021484095824,22.5861008342993,-6.));
#13039=CARTESIAN_POINT('Ctrl Pts',(84.7938584808496,22.5243223796457,-6.));
#13040=CARTESIAN_POINT('Ctrl Pts',(84.7821760832888,22.4631676164083,-6.));
#13041=CARTESIAN_POINT('Ctrl Pts',(84.7694456203586,22.3965264631396,-6.));
#13042=CARTESIAN_POINT('Ctrl Pts',(84.7526877740569,22.3306250945486,-6.));
#13043=CARTESIAN_POINT('Ctrl Pts',(84.7321477736998,22.2656770857153,-6.));
#13044=CARTESIAN_POINT('Ctrl Pts',(84.7242184256731,22.2406042835379,-6.));
#13045=CARTESIAN_POINT('Ctrl Pts',(84.7157248685372,22.2156736078728,-6.));
#13046=CARTESIAN_POINT('Ctrl Pts',(84.7066792009377,22.1908976666699,-6.));
#13047=CARTESIAN_POINT('Ctrl Pts',(84.702711832254,22.1800311062797,-6.));
#13048=CARTESIAN_POINT('Ctrl Pts',(84.6986383589894,22.1691948787475,-6.));
#13049=CARTESIAN_POINT('Ctrl Pts',(84.6944648872271,22.158402584267,-6.));
#13050=CARTESIAN_POINT('Ctrl Pts',(84.6692420795077,22.093178237719,-6.));
#13051=CARTESIAN_POINT('Ctrl Pts',(84.6403284563561,22.0294393145623,-6.));
#13052=CARTESIAN_POINT('Ctrl Pts',(84.6080366728143,21.9674046173891,-6.));
#13053=CARTESIAN_POINT('Ctrl Pts',(84.5749968927465,21.9039329683697,-6.));
#13054=CARTESIAN_POINT('Ctrl Pts',(84.5384203362702,21.8422445927193,-6.));
#13055=CARTESIAN_POINT('Ctrl Pts',(84.4985857546133,21.7825775666462,-6.));
#13056=CARTESIAN_POINT('Ctrl Pts',(84.4680931898081,21.736903667647,-6.));
#13057=CARTESIAN_POINT('Ctrl Pts',(84.4356903395602,21.6924141647768,-6.));
#13058=CARTESIAN_POINT('Ctrl Pts',(84.4014826868376,21.6492219482087,-6.));
#13059=CARTESIAN_POINT('Ctrl Pts',(84.3801861847344,21.6223319672315,-6.));
#13060=CARTESIAN_POINT('Ctrl Pts',(84.3581898396724,21.5959449213339,-6.));
#13061=CARTESIAN_POINT('Ctrl Pts',(84.3355161968359,21.5700897403578,-6.));
#13062=CARTESIAN_POINT('Ctrl Pts',(84.3228380888485,21.5556326555914,-6.));
#13063=CARTESIAN_POINT('Ctrl Pts',(84.3099437537492,21.5413373293104,-6.));
#13064=CARTESIAN_POINT('Ctrl Pts',(84.2968608165032,21.5272342242042,-6.));
#13065=CARTESIAN_POINT('Ctrl Pts',(84.2459896381448,21.4723962652833,-6.));
#13066=CARTESIAN_POINT('Ctrl Pts',(84.1922219184366,21.4204032503112,-6.));
#13067=CARTESIAN_POINT('Ctrl Pts',(84.1358426011268,21.3715190959182,-6.));
#13068=CARTESIAN_POINT('Ctrl Pts',(84.0936830787195,21.3349643325611,-6.));
#13069=CARTESIAN_POINT('Ctrl Pts',(84.0500620462463,21.3001481807965,-6.));
#13070=CARTESIAN_POINT('Ctrl Pts',(84.0050822634579,21.2671907406919,-6.));
#13071=CARTESIAN_POINT('Ctrl Pts',(83.9910186215557,21.2568860747528,-6.));
#13072=CARTESIAN_POINT('Ctrl Pts',(83.9768220557377,21.2467631932491,-6.));
#13073=CARTESIAN_POINT('Ctrl Pts',(83.9624954655677,21.2368259940225,-6.));
#13074=CARTESIAN_POINT('Ctrl Pts',(83.9487061337562,21.2272614475543,-6.));
#13075=CARTESIAN_POINT('Ctrl Pts',(83.9348033877552,21.2178738647995,-6.));
#13076=CARTESIAN_POINT('Ctrl Pts',(83.9207951867164,21.2086694621281,-6.));
#13077=CARTESIAN_POINT('Ctrl Pts',(83.8578415491727,21.1673043626424,-6.));
#13078=CARTESIAN_POINT('Ctrl Pts',(83.7927304527034,21.1296149339887,-6.));
#13079=CARTESIAN_POINT('Ctrl Pts',(83.7257231789248,21.0958803410021,-6.));
#13080=CARTESIAN_POINT('Ctrl Pts',(83.6744958173968,21.0700900932652,-6.));
#13081=CARTESIAN_POINT('Ctrl Pts',(83.6221592285687,21.0466117245125,-6.));
#13082=CARTESIAN_POINT('Ctrl Pts',(83.5688162931808,21.0255852276549,-6.));
#13083=CARTESIAN_POINT('Ctrl Pts',(83.5563690536895,21.0206788264576,-6.));
#13084=CARTESIAN_POINT('Ctrl Pts',(83.5438669750959,21.0159059951676,-6.));
#13085=CARTESIAN_POINT('Ctrl Pts',(83.5313119958266,21.0112661450614,-6.));
#13086=CARTESIAN_POINT('Ctrl Pts',(81.3326822579993,22.9986976815004,-7.12851963660979));
#13087=CARTESIAN_POINT('Ctrl Pts',(81.3319479721743,22.9132137610073,-7.12279015104506));
#13088=CARTESIAN_POINT('Ctrl Pts',(81.3379545916533,22.8278333679087,-7.11706066548032));
#13089=CARTESIAN_POINT('Ctrl Pts',(81.3510611587958,22.7435572384718,-7.11133117991559));
#13090=CARTESIAN_POINT('Ctrl Pts',(81.4358025464977,22.1986642790157,-7.07428680725174));
#13091=CARTESIAN_POINT('Ctrl Pts',(81.8173469963478,21.6999334677524,-7.03724243458788));
#13092=CARTESIAN_POINT('Ctrl Pts',(82.3210928586109,21.4755853719685,-7.00019806192403));
#13093=CARTESIAN_POINT('Ctrl Pts',(82.824838720874,21.2512372761846,-6.96315368926018));
#13094=CARTESIAN_POINT('Ctrl Pts',(83.45078599555,21.3012718958802,-6.92610931659632));
#13095=CARTESIAN_POINT('Ctrl Pts',(83.9124876961019,21.6028092908236,-6.88906494393247));
#13096=CARTESIAN_POINT('Ctrl Pts',(84.3741893966538,21.904346685767,-6.85202057126862));
#13097=CARTESIAN_POINT('Ctrl Pts',(84.6716455230816,22.4573868559583,-6.81497619860477));
#13098=CARTESIAN_POINT('Ctrl Pts',(84.6687366815921,23.0088140573203,-6.77793182594091));
#13099=CARTESIAN_POINT('Ctrl Pts',(84.6658278401026,23.5602412586823,-6.74088745327706));
#13100=CARTESIAN_POINT('Ctrl Pts',(84.3625540306957,24.1100554912149,-6.70384308061321));
#13101=CARTESIAN_POINT('Ctrl Pts',(83.8976945634842,24.4067181113346,-6.66679870794935));
#13102=CARTESIAN_POINT('Ctrl Pts',(83.4328350962727,24.7033807314542,-6.6297543352855));
#13103=CARTESIAN_POINT('Ctrl Pts',(82.8063899712565,24.746891739161,-6.59270996262165));
#13104=CARTESIAN_POINT('Ctrl Pts',(82.3050422822643,24.5172056670904,-6.5556655899578));
#13105=CARTESIAN_POINT('Ctrl Pts',(81.8036945932721,24.2875195950198,-6.51862121729394));
#13106=CARTESIAN_POINT('Ctrl Pts',(81.4274443403038,23.7846364431718,-6.48157684463009));
#13107=CARTESIAN_POINT('Ctrl Pts',(81.3484521953559,23.2389527734919,-6.44453247196624));
#13108=CARTESIAN_POINT('Ctrl Pts',(81.3370704557417,23.1603268614577,-6.43919486018075));
#13109=CARTESIAN_POINT('Ctrl Pts',(81.3318601088966,23.080812365398,-6.43385724839527));
#13110=CARTESIAN_POINT('Ctrl Pts',(81.3325224760112,23.0012132743929,-6.42851963660979));
#13111=CARTESIAN_POINT('Ctrl Pts',(82.4698297828114,21.0148256743283,-6.));
#13112=CARTESIAN_POINT('Ctrl Pts',(81.8097404375819,21.1911123142463,-6.03704437266385));
#13113=CARTESIAN_POINT('Ctrl Pts',(80.6907279345985,22.2513783981503,-6.11113311799155));
#13114=CARTESIAN_POINT('Ctrl Pts',(81.1186741999742,24.5381192006252,-6.22226623598312));
#13115=CARTESIAN_POINT('Ctrl Pts',(83.2718171861771,25.4128332182024,-6.33339935397467));
#13116=CARTESIAN_POINT('Ctrl Pts',(85.1745320403748,24.0812968093214,-6.44453247196624));
#13117=CARTESIAN_POINT('Ctrl Pts',(85.0878555272437,21.7590837146758,-6.55566558995779));
#13118=CARTESIAN_POINT('Ctrl Pts',(83.0898774457969,20.5731226537472,-6.66679870794935));
#13119=CARTESIAN_POINT('Ctrl Pts',(81.0098475676149,21.6080762686228,-6.77793182594092));
#13120=CARTESIAN_POINT('Ctrl Pts',(80.7511794463617,23.9171031255975,-6.88906494393247));
#13121=CARTESIAN_POINT('Ctrl Pts',(82.5507725952567,25.3866959940047,-7.00019806192404));
#13122=CARTESIAN_POINT('Ctrl Pts',(84.7614901796242,24.6719233964163,-7.11133117991558));
#13123=CARTESIAN_POINT('Ctrl Pts',(85.3600357402078,22.4269243306697,-7.22246429790715));
#13124=CARTESIAN_POINT('Ctrl Pts',(83.7985771227055,20.7064348813032,-7.33359741589871));
#13125=CARTESIAN_POINT('Ctrl Pts',(81.5062325893395,21.0851023869821,-7.44473053389026));
#13126=CARTESIAN_POINT('Ctrl Pts',(80.5810411304203,23.2163616212335,-7.55586365188184));
#13127=CARTESIAN_POINT('Ctrl Pts',(81.8697768675109,25.1495971491679,-7.66699676987337));
#13128=CARTESIAN_POINT('Ctrl Pts',(84.1929368847996,25.1154372776465,-7.77812988786495));
#13129=CARTESIAN_POINT('Ctrl Pts',(85.4242743200689,23.1451456867025,-7.8892630058565));
#13130=CARTESIAN_POINT('Ctrl Pts',(84.4368203745666,21.042011180836,-8.00039612384806));
#13131=CARTESIAN_POINT('Ctrl Pts',(82.1343319219779,20.7309050425608,-8.11152924183962));
#13132=CARTESIAN_POINT('Ctrl Pts',(80.6241369404767,22.4965639528314,-8.22266235983118));
#13133=CARTESIAN_POINT('Ctrl Pts',(81.2884253572881,24.7229873320792,-8.33379547782273));
#13134=CARTESIAN_POINT('Ctrl Pts',(83.5192142474232,25.3724648971313,-8.44492859581431));
#13135=CARTESIAN_POINT('Ctrl Pts',(85.2747978255561,23.850569204887,-8.55606171380586));
#13136=CARTESIAN_POINT('Ctrl Pts',(84.9483968969088,21.5501991003249,-8.66719483179741));
#13137=CARTESIAN_POINT('Ctrl Pts',(82.8387464408891,20.5767438417137,-8.77832794978898));
#13138=CARTESIAN_POINT('Ctrl Pts',(80.8766815886281,21.8211479981201,-8.88946106778053));
#13139=CARTESIAN_POINT('Ctrl Pts',(80.8579613196625,24.1444839055483,-9.00059418577209));
#13140=CARTESIAN_POINT('Ctrl Pts',(82.7997191606577,25.4203430963022,-9.11172730376366));
#13141=CARTESIAN_POINT('Ctrl Pts',(84.9247819088485,24.4810090214786,-9.22286042175521));
#13142=CARTESIAN_POINT('Ctrl Pts',(85.2882084953573,22.1861971982837,-9.33399353974677));
#13143=CARTESIAN_POINT('Ctrl Pts',(83.5573766039194,20.6362097301691,-9.44512665773833));
#13144=CARTESIAN_POINT('Ctrl Pts',(81.3164117064387,21.2496561548905,-9.55625977572989));
#13145=CARTESIAN_POINT('Ctrl Pts',(80.6163330806179,23.4650861595143,-9.66739289372146));
#13146=CARTESIAN_POINT('Ctrl Pts',(82.0978802396299,25.2548510053398,-9.778526011713));
#13147=CARTESIAN_POINT('Ctrl Pts',(84.4050829104209,24.9808874610066,-9.88965912970457));
#13148=CARTESIAN_POINT('Ctrl Pts',(85.4262983980702,22.8939377453899,-10.0007922476961));
#13149=CARTESIAN_POINT('Ctrl Pts',(84.2268700936312,20.9040603797618,-10.1119253656877));
#13150=CARTESIAN_POINT('Ctrl Pts',(81.9045619903646,20.8324694499553,-10.2230584836792));
#13151=CARTESIAN_POINT('Ctrl Pts',(80.5848418695363,22.7446877927209,-10.3341916016708));
#13152=CARTESIAN_POINT('Ctrl Pts',(81.4755695294061,24.8905779165788,-10.4453247196624));
#13153=CARTESIAN_POINT('Ctrl Pts',(83.7615159569619,25.3061367187622,-10.5564578376539));
#13154=CARTESIAN_POINT('Ctrl Pts',(85.3504930077305,23.6110284272776,-10.6675909556455));
#13155=CARTESIAN_POINT('Ctrl Pts',(84.7882063433206,21.3566828693041,-10.778724073637));
#13156=CARTESIAN_POINT('Ctrl Pts',(82.5892828503881,20.6063658296754,-10.8898571916286));
#13157=CARTESIAN_POINT('Ctrl Pts',(80.7662638584498,22.0467969952507,-11.0009903096202));
#13158=CARTESIAN_POINT('Ctrl Pts',(80.987648102256,24.3596370684772,-11.1121234276117));
#13159=CARTESIAN_POINT('Ctrl Pts',(83.0508160082765,25.4280837818398,-11.2232565456033));
#13160=CARTESIAN_POINT('Ctrl Pts',(85.0674751034236,24.2742526496163,-11.3343896635948));
#13161=CARTESIAN_POINT('Ctrl Pts',(85.1918996088904,21.9541753383684,-11.4455227815864));
#13162=CARTESIAN_POINT('Ctrl Pts',(83.3102113199728,20.5912779207033,-11.5566558995779));
#13163=CARTESIAN_POINT('Ctrl Pts',(81.1446054212175,21.4329377563877,-11.6677890175695));
#13164=CARTESIAN_POINT('Ctrl Pts',(80.6771296685829,23.708834636395,-11.7789221355611));
#13165=CARTESIAN_POINT('Ctrl Pts',(82.3356362705467,25.3359781577142,-11.8900552535526));
#13166=CARTESIAN_POINT('Ctrl Pts',(84.6021947068076,24.825142525889,-12.0011883715442));
#13167=CARTESIAN_POINT('Ctrl Pts',(85.4023614856292,22.6438646174604,-12.1123214895358));
#13168=CARTESIAN_POINT('Ctrl Pts',(84.0037924767762,20.7885358284841,-12.2234546075273));
#13169=CARTESIAN_POINT('Ctrl Pts',(81.6865130842908,20.9572260916608,-12.3345877255189));
#13170=CARTESIAN_POINT('Ctrl Pts',(80.5713886154037,22.995543438547,-12.4457208435104));
#13171=CARTESIAN_POINT('Ctrl Pts',(81.6790248749117,25.0379396058836,-12.556853961502));
#13172=CARTESIAN_POINT('Ctrl Pts',(83.9956695619749,25.2151332333942,-12.6679870794935));
#13173=CARTESIAN_POINT('Ctrl Pts',(85.4010382767464,23.364949738908,-12.7791201974851));
#13174=CARTESIAN_POINT('Ctrl Pts',(84.6088822566941,21.1807498790914,-12.8902533154767));
#13175=CARTESIAN_POINT('Ctrl Pts',(82.3442138703267,20.6615993349174,-13.0013864334682));
#13176=CARTESIAN_POINT('Ctrl Pts',(80.6797467613269,22.2826451179802,-13.1125195514598));
#13177=CARTESIAN_POINT('Ctrl Pts',(81.1388667406383,24.5602423238806,-13.2236526694513));
#13178=CARTESIAN_POINT('Ctrl Pts',(83.3013691324087,25.409844344426,-13.3347857874429));
#13179=CARTESIAN_POINT('Ctrl Pts',(85.1880466324256,24.0538619704037,-13.4459189054344));
#13180=CARTESIAN_POINT('Ctrl Pts',(85.0721377337693,21.7333436414648,-13.557052023426));
#13181=CARTESIAN_POINT('Ctrl Pts',(83.0597268226234,20.5721190669662,-13.6681851414176));
#13182=CARTESIAN_POINT('Ctrl Pts',(80.9926515725825,21.6329866828416,-13.7793182594091));
#13183=CARTESIAN_POINT('Ctrl Pts',(80.7627806117888,23.9449986917019,-13.8904513774007));
#13184=CARTESIAN_POINT('Ctrl Pts',(82.5805008911621,25.3921107031273,-14.0015844953923));
#13185=CARTESIAN_POINT('Ctrl Pts',(84.7821632663096,24.6498688464973,-14.1127176133838));
#13186=CARTESIAN_POINT('Ctrl Pts',(85.3527196747847,22.397602083335,-14.2238507313754));
#13187=CARTESIAN_POINT('Ctrl Pts',(83.7699744349188,20.6966736036812,-14.3349838493669));
#13188=CARTESIAN_POINT('Ctrl Pts',(81.4825182859858,21.1038400999306,-14.4461169673585));
#13189=CARTESIAN_POINT('Ctrl Pts',(80.5839211298768,23.2464467689522,-14.5572500853501));
#13190=CARTESIAN_POINT('Ctrl Pts',(81.8966144503262,25.1634956547744,-14.6683832033416));
#13191=CARTESIAN_POINT('Ctrl Pts',(84.2191696572937,25.1004281633947,-14.7795163213332));
#13192=CARTESIAN_POINT('Ctrl Pts',(85.4258928026212,23.1149661440179,-14.8906494393247));
#13193=CARTESIAN_POINT('Ctrl Pts',(84.4123433832198,21.0242825862308,-15.0017825573163));
#13194=CARTESIAN_POINT('Ctrl Pts',(82.1061616893797,20.7418533657775,-15.1129156753078));
#13195=CARTESIAN_POINT('Ctrl Pts',(80.6180560400795,22.5261688311867,-15.2240487932994));
#13196=CARTESIAN_POINT('Ctrl Pts',(81.3099991724782,24.7441532192698,-15.335181911291));
#13197=CARTESIAN_POINT('Ctrl Pts',(83.5486977451864,25.3658199574776,-15.4463150292825));
#13198=CARTESIAN_POINT('Ctrl Pts',(85.2852062155397,23.822195101775,-15.5574481472741));
#13199=CARTESIAN_POINT('Ctrl Pts',(84.9302046695978,21.5260650294792,-15.6685812652657));
#13200=CARTESIAN_POINT('Ctrl Pts',(82.8086025275965,20.5789380526202,-15.7797143832572));
#13201=CARTESIAN_POINT('Ctrl Pts',(80.862177498975,21.8476626671313,-15.8908475012488));
#13202=CARTESIAN_POINT('Ctrl Pts',(80.8723665552161,24.1710509563948,-16.0019806192403));
#13203=CARTESIAN_POINT('Ctrl Pts',(82.8298598776186,25.4226489294061,-16.1131137372319));
#13204=CARTESIAN_POINT('Ctrl Pts',(84.9430514056717,24.4569400344173,-16.2242468552234));
#13205=CARTESIAN_POINT('Ctrl Pts',(85.2779271552008,22.1577886838534,-16.335379973215));
#13206=CARTESIAN_POINT('Ctrl Pts',(83.5278718544653,20.6294494978248,-16.4465130912065));
#13207=CARTESIAN_POINT('Ctrl Pts',(81.2948519124425,21.270756926133,-16.5576462091981));
#13208=CARTESIAN_POINT('Ctrl Pts',(80.6221226182225,23.4946848360884,-16.6687793271897));
#13209=CARTESIAN_POINT('Ctrl Pts',(82.12637451265,25.2659591550417,-16.7799124451812));
#13210=CARTESIAN_POINT('Ctrl Pts',(84.4288972422666,24.9631356021949,-16.8910455631728));
#13211=CARTESIAN_POINT('Ctrl Pts',(85.4262517081314,22.8639849641985,-17.0021786811644));
#13212=CARTESIAN_POINT('Ctrl Pts',(84.1976566851383,20.8884152303676,-17.1133117991559));
#13213=CARTESIAN_POINT('Ctrl Pts',(82.656339145916,20.8620828587222,-17.1874005444836));
#13214=CARTESIAN_POINT('Ctrl Pts',(82.0504464477385,21.1778184465077,-17.2244449171475));
#13215=CARTESIAN_POINT('Ctrl Pts',(82.5032651029123,21.1400211999972,-5.92518502761751));
#13216=CARTESIAN_POINT('Ctrl Pts',(81.8848044607624,21.3051902779624,-5.96222940028136));
#13217=CARTESIAN_POINT('Ctrl Pts',(80.8363627669665,22.2985904105961,-6.03631814560907));
#13218=CARTESIAN_POINT('Ctrl Pts',(81.2373204918605,24.4411173205517,-6.14745126360063));
#13219=CARTESIAN_POINT('Ctrl Pts',(83.2546749659352,25.2606672752935,-6.25858438159218));
#13220=CARTESIAN_POINT('Ctrl Pts',(85.0373946220844,24.0131045499835,-6.36971749958376));
#13221=CARTESIAN_POINT('Ctrl Pts',(84.9561843853828,21.8373424170191,-6.4808506175753));
#13222=CARTESIAN_POINT('Ctrl Pts',(83.0842093017319,20.7261742931771,-6.59198373556687));
#13223=CARTESIAN_POINT('Ctrl Pts',(81.1353570388546,21.6958582941041,-6.70311685355843));
#13224=CARTESIAN_POINT('Ctrl Pts',(80.8930018887069,23.8592657828428,-6.81424997154998));
#13225=CARTESIAN_POINT('Ctrl Pts',(82.5791032362258,25.2361784018127,-6.92538308954154));
#13226=CARTESIAN_POINT('Ctrl Pts',(84.6504013517329,24.5664831205747,-7.0365162075331));
#13227=CARTESIAN_POINT('Ctrl Pts',(85.211199483728,22.4630654940639,-7.14764932552466));
#13228=CARTESIAN_POINT('Ctrl Pts',(83.7482146525832,20.8510791510673,-7.25878244351622));
#13229=CARTESIAN_POINT('Ctrl Pts',(81.6004374124557,21.2058658938257,-7.36991556150778));
#13230=CARTESIAN_POINT('Ctrl Pts',(80.7335933890972,23.2027167203527,-7.48104867949935));
#13231=CARTESIAN_POINT('Ctrl Pts',(81.9410546779104,25.0140322561575,-7.59218179749089));
#13232=CARTESIAN_POINT('Ctrl Pts',(84.1177040155997,24.9820266856548,-7.70331491548246));
#13233=CARTESIAN_POINT('Ctrl Pts',(85.2713868411497,23.1359920369145,-7.81444803347401));
#13234=CARTESIAN_POINT('Ctrl Pts',(84.3462069308205,21.1654922455966,-7.92558115146558));
#13235=CARTESIAN_POINT('Ctrl Pts',(82.1889255003257,20.8740060953579,-8.03671426945714));
#13236=CARTESIAN_POINT('Ctrl Pts',(80.77397135089,22.5283132756747,-8.14784738744869));
#13237=CARTESIAN_POINT('Ctrl Pts',(81.3963662491004,24.6143266960982,-8.25898050544026));
#13238=CARTESIAN_POINT('Ctrl Pts',(83.4864698683528,25.2228447926969,-8.3701136234318));
#13239=CARTESIAN_POINT('Ctrl Pts',(85.1313371199251,23.7969278408281,-8.48124674142338));
#13240=CARTESIAN_POINT('Ctrl Pts',(84.8255207491744,21.6416311642011,-8.59237985941492));
#13241=CARTESIAN_POINT('Ctrl Pts',(82.8489159377628,20.72956711,-8.70351297740649));
#13242=CARTESIAN_POINT('Ctrl Pts',(81.0105892063304,21.8954926005828,-8.81464609539804));
#13243=CARTESIAN_POINT('Ctrl Pts',(80.9930495359063,24.0723067358551,-8.92577921338961));
#13244=CARTESIAN_POINT('Ctrl Pts',(82.812349922923,25.2677035410137,-9.03691233138117));
#13245=CARTESIAN_POINT('Ctrl Pts',(84.8033950463649,24.3876088094334,-9.14804544937272));
#13246=CARTESIAN_POINT('Ctrl Pts',(85.1439020424116,22.23751987974,-9.25917856736428));
#13247=CARTESIAN_POINT('Ctrl Pts',(83.5222255060935,20.7852827670182,-9.37031168535585));
#13248=CARTESIAN_POINT('Ctrl Pts',(81.4225876319967,21.3600420363499,-9.48144480334739));
#13249=CARTESIAN_POINT('Ctrl Pts',(80.7666596434456,23.4357553821267,-9.59257792133896));
#13250=CARTESIAN_POINT('Ctrl Pts',(82.1547726526311,25.1126482510184,-9.70371103933051));
#13251=CARTESIAN_POINT('Ctrl Pts',(84.3164709979538,24.8559622875522,-9.81484415732209));
#13252=CARTESIAN_POINT('Ctrl Pts',(85.2732832701551,22.9006265885549,-9.92597727531363));
#13253=CARTESIAN_POINT('Ctrl Pts',(84.1494972179531,21.0362413470112,-10.0371103933052));
#13254=CARTESIAN_POINT('Ctrl Pts',(81.9736460681105,20.9691653174705,-10.1482435112967));
#13255=CARTESIAN_POINT('Ctrl Pts',(80.7371544336306,22.7607891222548,-10.2593766292883));
#13256=CARTESIAN_POINT('Ctrl Pts',(81.5717081262252,24.7713481376,-10.3705097472799));
#13257=CARTESIAN_POINT('Ctrl Pts',(83.7134907587191,25.1606996178304,-10.4816428652715));
#13258=CARTESIAN_POINT('Ctrl Pts',(85.2022585661105,23.5724937635141,-10.592775983263));
#13259=CARTESIAN_POINT('Ctrl Pts',(84.6754326537451,21.4603190836949,-10.7039091012546));
#13260=CARTESIAN_POINT('Ctrl Pts',(82.6151848322855,20.7573209797283,-10.8150422192461));
#13261=CARTESIAN_POINT('Ctrl Pts',(80.9071349984957,22.1069109861005,-10.9261753372377));
#13262=CARTESIAN_POINT('Ctrl Pts',(81.1145575884463,24.2738912096346,-11.0373084552292));
#13263=CARTESIAN_POINT('Ctrl Pts',(83.047611283741,25.2749560582416,-11.1484415732208));
#13264=CARTESIAN_POINT('Ctrl Pts',(84.9370892581942,24.1938915809481,-11.2595746912123));
#13265=CARTESIAN_POINT('Ctrl Pts',(85.0536669004577,22.0201305376561,-11.3707078092039));
#13266=CARTESIAN_POINT('Ctrl Pts',(83.2906477638809,20.7431845935875,-11.4818409271955));
#13267=CARTESIAN_POINT('Ctrl Pts',(81.2616163540157,21.5317649368565,-11.592974045187));
#13268=CARTESIAN_POINT('Ctrl Pts',(80.823622079069,23.6641317990833,-11.7041071631786));
#13269=CARTESIAN_POINT('Ctrl Pts',(82.3775345387585,25.1886590988163,-11.8152402811702));
#13270=CARTESIAN_POINT('Ctrl Pts',(84.5011518885781,24.7100394465299,-11.9263733991617));
#13271=CARTESIAN_POINT('Ctrl Pts',(85.2508559452084,22.6663243862826,-12.0375065171533));
#13272=CARTESIAN_POINT('Ctrl Pts',(83.9404880479573,20.9280023810537,-12.1486396351448));
#13273=CARTESIAN_POINT('Ctrl Pts',(81.7693484719668,21.086054149716,-12.2597727531364));
#13274=CARTESIAN_POINT('Ctrl Pts',(80.7245496124044,22.9958244927328,-12.3709058711279));
#13275=CARTESIAN_POINT('Ctrl Pts',(81.762332508424,24.9094164243469,-12.4820389891195));
#13276=CARTESIAN_POINT('Ctrl Pts',(83.9328774068518,25.0754352905006,-12.593172107111));
#13277=CARTESIAN_POINT('Ctrl Pts',(85.2496161848318,23.3419340904511,-12.7043052251026));
#13278=CARTESIAN_POINT('Ctrl Pts',(84.5074176864236,21.2954813524261,-12.8154383430942));
#13279=CARTESIAN_POINT('Ctrl Pts',(82.3855711900186,20.8090711698609,-12.9265714610857));
#13280=CARTESIAN_POINT('Ctrl Pts',(80.8260741241908,22.3278852867575,-13.0377045790773));
#13281=CARTESIAN_POINT('Ctrl Pts',(81.2562395847924,24.4618452433909,-13.1488376970688));
#13282=CARTESIAN_POINT('Ctrl Pts',(83.2823632111329,25.2578668956049,-13.2599708150604));
#13283=CARTESIAN_POINT('Ctrl Pts',(85.0500569129374,23.9873998961863,-13.371103933052));
#13284=CARTESIAN_POINT('Ctrl Pts',(84.9414578385667,21.8132256480966,-13.4822370510435));
#13285=CARTESIAN_POINT('Ctrl Pts',(83.0559601353062,20.7252339978527,-13.5933701690351));
#13286=CARTESIAN_POINT('Ctrl Pts',(81.1192455136393,21.7191977266905,-13.7045032870266));
#13287=CARTESIAN_POINT('Ctrl Pts',(80.9038714236746,23.885402107949,-13.8156364050182));
#13288=CARTESIAN_POINT('Ctrl Pts',(82.6069567095603,25.2412516309221,-13.9267695230098));
#13289=CARTESIAN_POINT('Ctrl Pts',(84.6697706849286,24.5458194464769,-14.0379026410013));
#13290=CARTESIAN_POINT('Ctrl Pts',(85.2043448078386,22.4355924617434,-14.1490357589929));
#13291=CARTESIAN_POINT('Ctrl Pts',(83.721415800604,20.8419334709107,-14.2601688769844));
#13292=CARTESIAN_POINT('Ctrl Pts',(81.5782186576973,21.2234219081233,-14.371301994976));
#13293=CARTESIAN_POINT('Ctrl Pts',(80.7362917606528,23.2309045405497,-14.4824351129676));
#13294=CARTESIAN_POINT('Ctrl Pts',(81.9661997417136,25.0270542489596,-14.5935682309591));
#13295=CARTESIAN_POINT('Ctrl Pts',(84.1422824115993,24.9679641250252,-14.7047013489507));
#13296=CARTESIAN_POINT('Ctrl Pts',(85.2729032536867,23.1077157747943,-14.8158344669422));
#13297=CARTESIAN_POINT('Ctrl Pts',(84.3232735871819,21.1488817093362,-14.9269675849338));
#13298=CARTESIAN_POINT('Ctrl Pts',(82.1625318306384,20.8842639597758,-15.0381007029254));
#13299=CARTESIAN_POINT('Ctrl Pts',(80.7682739440287,22.5560511148183,-15.1492338209169));
#13300=CARTESIAN_POINT('Ctrl Pts',(81.4165795061277,24.6341577512094,-15.2603669389085));
#13301=CARTESIAN_POINT('Ctrl Pts',(83.5140939818022,25.216618917859,-15.3715000569));
#13302=CARTESIAN_POINT('Ctrl Pts',(85.1410891021372,23.7703431577729,-15.4826331748916));
#13303=CARTESIAN_POINT('Ctrl Pts',(84.8084758193231,21.6190191146948,-15.5937662928831));
#13304=CARTESIAN_POINT('Ctrl Pts',(82.8206730580578,20.7316229424355,-15.7048994108747));
#13305=CARTESIAN_POINT('Ctrl Pts',(80.9969998207942,21.9203351152235,-15.8160325288663));
#13306=CARTESIAN_POINT('Ctrl Pts',(81.006546301602,24.0971983288573,-15.9271656468579));
#13307=CARTESIAN_POINT('Ctrl Pts',(82.840589807874,25.2698639561642,-16.0382987648494));
#13308=CARTESIAN_POINT('Ctrl Pts',(84.8205123727065,24.365057739186,-16.1494318828409));
#13309=CARTESIAN_POINT('Ctrl Pts',(85.1342690975971,22.210902955525,-16.2605650008325));
#13310=CARTESIAN_POINT('Ctrl Pts',(83.4945814811962,20.7789488704525,-16.371698118824));
#13311=CARTESIAN_POINT('Ctrl Pts',(81.4023875119133,21.379812082067,-16.4828312368156));
#13312=CARTESIAN_POINT('Ctrl Pts',(80.7720840623829,23.4634874106061,-16.5939643548072));
#13313=CARTESIAN_POINT('Ctrl Pts',(82.1814699270488,25.1230558624233,-16.7050974727988));
#13314=CARTESIAN_POINT('Ctrl Pts',(84.3387834728816,24.8393299542485,-16.8162305907903));
#13315=CARTESIAN_POINT('Ctrl Pts',(85.2732395247293,22.8725627871564,-16.9273637087819));
#13316=CARTESIAN_POINT('Ctrl Pts',(84.122126160525,21.0215828629579,-17.0384968267734));
#13317=CARTESIAN_POINT('Ctrl Pts',(82.6780122054164,20.996911149053,-17.1125855721011));
#13318=CARTESIAN_POINT('Ctrl Pts',(82.1103302849355,21.2927347913867,-17.149629944765));
#13319=CARTESIAN_POINT('Ctrl Pts',(82.5367004230132,21.2652167256662,-5.85037005523502));
#13320=CARTESIAN_POINT('Ctrl Pts',(81.9598684839428,21.4192682416784,-5.88741442789887));
#13321=CARTESIAN_POINT('Ctrl Pts',(80.9819975993346,22.3458024230419,-5.96150317322658));
#13322=CARTESIAN_POINT('Ctrl Pts',(81.3559667837468,24.3441154404782,-6.07263629121814));
#13323=CARTESIAN_POINT('Ctrl Pts',(83.2375327456932,25.1085013323846,-6.1837694092097));
#13324=CARTESIAN_POINT('Ctrl Pts',(84.9002572037943,23.9449122906456,-6.29490252720126));
#13325=CARTESIAN_POINT('Ctrl Pts',(84.8245132435218,21.9156011193624,-6.40603564519281));
#13326=CARTESIAN_POINT('Ctrl Pts',(83.0785411576668,20.8792259326071,-6.51716876318437));
#13327=CARTESIAN_POINT('Ctrl Pts',(81.2608665100943,21.7836403195853,-6.62830188117594));
#13328=CARTESIAN_POINT('Ctrl Pts',(81.0348243310523,23.801428440088,-6.73943499916749));
#13329=CARTESIAN_POINT('Ctrl Pts',(82.6074338771949,25.0856608096207,-6.85056811715905));
#13330=CARTESIAN_POINT('Ctrl Pts',(84.5393125238417,24.461042844733,-6.96170123515062));
#13331=CARTESIAN_POINT('Ctrl Pts',(85.0623632272481,22.499206657458,-7.07283435314217));
#13332=CARTESIAN_POINT('Ctrl Pts',(83.6978521824609,20.9957234208314,-7.18396747113373));
#13333=CARTESIAN_POINT('Ctrl Pts',(81.6946422355719,21.3266294006694,-7.29510058912529));
#13334=CARTESIAN_POINT('Ctrl Pts',(80.8861456477742,23.1890718194718,-7.40623370711685));
#13335=CARTESIAN_POINT('Ctrl Pts',(82.01233248831,24.8784673631472,-7.5173668251084));
#13336=CARTESIAN_POINT('Ctrl Pts',(84.0424711463996,24.848616093663,-7.62849994309996));
#13337=CARTESIAN_POINT('Ctrl Pts',(85.1184993622307,23.1268383871266,-7.73963306109152));
#13338=CARTESIAN_POINT('Ctrl Pts',(84.2555934870742,21.2889733103571,-7.85076617908308));
#13339=CARTESIAN_POINT('Ctrl Pts',(82.2435190786735,21.017107148155,-7.96189929707465));
#13340=CARTESIAN_POINT('Ctrl Pts',(80.9238057613034,22.560062598518,-8.0730324150662));
#13341=CARTESIAN_POINT('Ctrl Pts',(81.5043071409126,24.5056660601172,-8.18416553305777));
#13342=CARTESIAN_POINT('Ctrl Pts',(83.4537254892822,25.0732246882625,-8.29529865104932));
#13343=CARTESIAN_POINT('Ctrl Pts',(84.9878764142944,23.7432864767692,-8.40643176904088));
#13344=CARTESIAN_POINT('Ctrl Pts',(84.7026446014396,21.7330632280773,-8.51756488703244));
#13345=CARTESIAN_POINT('Ctrl Pts',(82.8590854346367,20.8823903782863,-8.628698005024));
#13346=CARTESIAN_POINT('Ctrl Pts',(81.1444968240326,21.9698372030455,-8.73983112301556));
#13347=CARTESIAN_POINT('Ctrl Pts',(81.12813775215,24.0001295661618,-8.85096424100711));
#13348=CARTESIAN_POINT('Ctrl Pts',(82.8249806851885,25.1150639857251,-8.96209735899869));
#13349=CARTESIAN_POINT('Ctrl Pts',(84.6820081838812,24.2942085973882,-9.07323047699023));
#13350=CARTESIAN_POINT('Ctrl Pts',(84.9995955894661,22.2888425611964,-9.18436359498179));
#13351=CARTESIAN_POINT('Ctrl Pts',(83.4870744082675,20.9343558038673,-9.29549671297336));
#13352=CARTESIAN_POINT('Ctrl Pts',(81.5287635575549,21.4704279178093,-9.40662983096491));
#13353=CARTESIAN_POINT('Ctrl Pts',(80.9169862062732,23.4064246047392,-9.51776294895648));
#13354=CARTESIAN_POINT('Ctrl Pts',(82.2116650656326,24.970445496697,-9.62889606694802));
#13355=CARTESIAN_POINT('Ctrl Pts',(84.2278590854866,24.7310371140978,-9.74002918493959));
#13356=CARTESIAN_POINT('Ctrl Pts',(85.1202681422402,22.9073154317199,-9.85116230293115));
#13357=CARTESIAN_POINT('Ctrl Pts',(84.0721243422749,21.1684223142607,-9.9622954209227));
#13358=CARTESIAN_POINT('Ctrl Pts',(82.0427301458566,21.1058611849855,-10.0734285389143));
#13359=CARTESIAN_POINT('Ctrl Pts',(80.8894669977249,22.7768904517888,-10.1845616569058));
#13360=CARTESIAN_POINT('Ctrl Pts',(81.6678467230445,24.6521183586212,-10.2956947748974));
#13361=CARTESIAN_POINT('Ctrl Pts',(83.6654655604762,25.0152625168986,-10.406827892889));
#13362=CARTESIAN_POINT('Ctrl Pts',(85.0540241244907,23.5339590997506,-10.5179610108805));
#13363=CARTESIAN_POINT('Ctrl Pts',(84.5626589641695,21.5639552980856,-10.6290941288721));
#13364=CARTESIAN_POINT('Ctrl Pts',(82.6410868141831,20.9082761297812,-10.7402272468636));
#13365=CARTESIAN_POINT('Ctrl Pts',(81.0480061385414,22.1670249769504,-10.8513603648552));
#13366=CARTESIAN_POINT('Ctrl Pts',(81.2414670746365,24.188145350792,-10.9624934828467));
#13367=CARTESIAN_POINT('Ctrl Pts',(83.0444065592057,25.1218283346434,-11.0736266008383));
#13368=CARTESIAN_POINT('Ctrl Pts',(84.8067034129645,24.1135305122798,-11.1847597188299));
#13369=CARTESIAN_POINT('Ctrl Pts',(84.9154341920251,22.0860857369438,-11.2958928368214));
#13370=CARTESIAN_POINT('Ctrl Pts',(83.2710842077889,20.8950912664717,-11.407025954813));
#13371=CARTESIAN_POINT('Ctrl Pts',(81.3786272868141,21.6305921173251,-11.5181590728045));
#13372=CARTESIAN_POINT('Ctrl Pts',(80.9701144895549,23.6194289617716,-11.6292921907961));
#13373=CARTESIAN_POINT('Ctrl Pts',(82.4194328069704,25.0413400399184,-11.7404253087876));
#13374=CARTESIAN_POINT('Ctrl Pts',(84.4001090703485,24.5949363671707,-11.8515584267792));
#13375=CARTESIAN_POINT('Ctrl Pts',(85.0993504047878,22.6887841551048,-11.9626915447708));
#13376=CARTESIAN_POINT('Ctrl Pts',(83.8771836191383,21.0674689336232,-12.0738246627623));
#13377=CARTESIAN_POINT('Ctrl Pts',(81.8521838596429,21.2148822077712,-12.1849577807539));
#13378=CARTESIAN_POINT('Ctrl Pts',(80.8777106094051,22.9961055469186,-12.2960908987455));
#13379=CARTESIAN_POINT('Ctrl Pts',(81.8456401419364,24.7808932428103,-12.407224016737));
#13380=CARTESIAN_POINT('Ctrl Pts',(83.8700852517286,24.935737347607,-12.5183571347286));
#13381=CARTESIAN_POINT('Ctrl Pts',(85.0981940929171,23.3189184419942,-12.6294902527201));
#13382=CARTESIAN_POINT('Ctrl Pts',(84.4059531161532,21.4102128257608,-12.7406233707117));
#13383=CARTESIAN_POINT('Ctrl Pts',(82.4269285097103,20.9565430048045,-12.8517564887032));
#13384=CARTESIAN_POINT('Ctrl Pts',(80.9724014870548,22.3731254555347,-12.9628896066948));
#13385=CARTESIAN_POINT('Ctrl Pts',(81.3736124289465,24.3634481629012,-13.0740227246864));
#13386=CARTESIAN_POINT('Ctrl Pts',(83.2633572898572,25.1058894467837,-13.1851558426779));
#13387=CARTESIAN_POINT('Ctrl Pts',(84.9120671934491,23.9209378219689,-13.2962889606695));
#13388=CARTESIAN_POINT('Ctrl Pts',(84.810777943364,21.8931076547286,-13.407422078661));
#13389=CARTESIAN_POINT('Ctrl Pts',(83.052193447989,20.8783489287391,-13.5185551966526));
#13390=CARTESIAN_POINT('Ctrl Pts',(81.2458394546959,21.8054087705393,-13.6296883146441));
#13391=CARTESIAN_POINT('Ctrl Pts',(81.0449622355604,23.825805524196,-13.7408214326357));
#13392=CARTESIAN_POINT('Ctrl Pts',(82.6334125279584,25.0903925587169,-13.8519545506273));
#13393=CARTESIAN_POINT('Ctrl Pts',(84.5573781035476,24.4417700464565,-13.9630876686188));
#13394=CARTESIAN_POINT('Ctrl Pts',(85.0559699408925,22.4735828401516,-14.0742207866104));
#13395=CARTESIAN_POINT('Ctrl Pts',(83.6728571662892,20.9871933381401,-14.185353904602));
#13396=CARTESIAN_POINT('Ctrl Pts',(81.6739190294089,21.343003716316,-14.2964870225935));
#13397=CARTESIAN_POINT('Ctrl Pts',(80.8886623914287,23.2153623121472,-14.4076201405851));
#13398=CARTESIAN_POINT('Ctrl Pts',(82.0357850331013,24.8906128431449,-14.5187532585766));
#13399=CARTESIAN_POINT('Ctrl Pts',(84.0653951659045,24.8355000866556,-14.6298863765682));
#13400=CARTESIAN_POINT('Ctrl Pts',(85.1199137047525,23.1004654055706,-14.7410194945597));
#13401=CARTESIAN_POINT('Ctrl Pts',(84.2342037911438,21.2734808324417,-14.8521526125513));
#13402=CARTESIAN_POINT('Ctrl Pts',(82.218901971897,21.0266745537741,-14.9632857305429));
#13403=CARTESIAN_POINT('Ctrl Pts',(80.918491847978,22.5859333984499,-15.0744188485344));
#13404=CARTESIAN_POINT('Ctrl Pts',(81.5231598397772,24.524162283149,-15.185551966526));
#13405=CARTESIAN_POINT('Ctrl Pts',(83.479490218418,25.0674178782403,-15.2966850845176));
#13406=CARTESIAN_POINT('Ctrl Pts',(84.9969719887346,23.7184912137708,-15.4078182025091));
#13407=CARTESIAN_POINT('Ctrl Pts',(84.6867469690484,21.7119731999103,-15.5189513205007));
#13408=CARTESIAN_POINT('Ctrl Pts',(82.8327435885193,20.8843078322508,-15.6300844384922));
#13409=CARTESIAN_POINT('Ctrl Pts',(81.1318221426133,21.9930075633158,-15.7412175564838));
#13410=CARTESIAN_POINT('Ctrl Pts',(81.140726047988,24.0233457013197,-15.8523506744754));
#13411=CARTESIAN_POINT('Ctrl Pts',(82.8513197381292,25.1170789829222,-15.9634837924669));
#13412=CARTESIAN_POINT('Ctrl Pts',(84.6979733397415,24.2731754439547,-16.0746169104585));
#13413=CARTESIAN_POINT('Ctrl Pts',(84.9906110399931,22.2640172271967,-16.18575002845));
#13414=CARTESIAN_POINT('Ctrl Pts',(83.4612911079274,20.9284482430803,-16.2968831464416));
#13415=CARTESIAN_POINT('Ctrl Pts',(81.509923111384,21.4888672380009,-16.4080162644331));
#13416=CARTESIAN_POINT('Ctrl Pts',(80.9220455065434,23.4322899851238,-16.5191493824247));
#13417=CARTESIAN_POINT('Ctrl Pts',(82.2365653414475,24.980152569805,-16.6302825004163));
#13418=CARTESIAN_POINT('Ctrl Pts',(84.2486697034967,24.7155243063022,-16.7414156184078));
#13419=CARTESIAN_POINT('Ctrl Pts',(85.1202273413273,22.8811406101142,-16.8525487363994));
#13420=CARTESIAN_POINT('Ctrl Pts',(84.0465956359117,21.1547504955482,-16.9636818543909));
#13421=CARTESIAN_POINT('Ctrl Pts',(82.6996852649168,21.1317394393839,-17.0377705997186));
#13422=CARTESIAN_POINT('Ctrl Pts',(82.1702141221325,21.4076511362656,-17.0748149723825));
#13423=CARTESIAN_POINT('Ctrl Pts',(82.5701357431142,21.3904122513352,-5.77555508285253));
#13424=CARTESIAN_POINT('Ctrl Pts',(82.0349325071233,21.5333462053945,-5.81259945551638));
#13425=CARTESIAN_POINT('Ctrl Pts',(81.1276324317026,22.3930144354877,-5.88668820084408));
#13426=CARTESIAN_POINT('Ctrl Pts',(81.4746130756331,24.2471135604047,-5.99782131883566));
#13427=CARTESIAN_POINT('Ctrl Pts',(83.2203905254512,24.9563353894757,-6.1089544368272));
#13428=CARTESIAN_POINT('Ctrl Pts',(84.7631197855041,23.8767200313077,-6.22008755481878));
#13429=CARTESIAN_POINT('Ctrl Pts',(84.6928421016609,21.9938598217058,-6.33122067281032));
#13430=CARTESIAN_POINT('Ctrl Pts',(83.0728730136016,21.0322775720369,-6.44235379080189));
#13431=CARTESIAN_POINT('Ctrl Pts',(81.3863759813341,21.8714223450666,-6.55348690879345));
#13432=CARTESIAN_POINT('Ctrl Pts',(81.1766467733975,23.7435910973332,-6.66462002678501));
#13433=CARTESIAN_POINT('Ctrl Pts',(82.6357645181641,24.9351432174288,-6.77575314477656));
#13434=CARTESIAN_POINT('Ctrl Pts',(84.4282236959502,24.3556025688913,-6.88688626276812));
#13435=CARTESIAN_POINT('Ctrl Pts',(84.9135269707684,22.5353478208521,-6.99801938075968));
#13436=CARTESIAN_POINT('Ctrl Pts',(83.6474897123384,21.1403676905955,-7.10915249875123));
#13437=CARTESIAN_POINT('Ctrl Pts',(81.7888470586882,21.447392907513,-7.22028561674281));
#13438=CARTESIAN_POINT('Ctrl Pts',(81.038697906451,23.175426918591,-7.33141873473436));
#13439=CARTESIAN_POINT('Ctrl Pts',(82.0836102987095,24.7429024701368,-7.44255185272592));
#13440=CARTESIAN_POINT('Ctrl Pts',(83.9672382771997,24.7152055016712,-7.55368497071747));
#13441=CARTESIAN_POINT('Ctrl Pts',(84.9656118833117,23.1176847373386,-7.66481808870904));
#13442=CARTESIAN_POINT('Ctrl Pts',(84.1649800433279,21.4124543751176,-7.7759512067006));
#13443=CARTESIAN_POINT('Ctrl Pts',(82.2981126570216,21.1602082009521,-7.88708432469216));
#13444=CARTESIAN_POINT('Ctrl Pts',(81.0736401717165,22.5918119213613,-7.99821744268371));
#13445=CARTESIAN_POINT('Ctrl Pts',(81.6122480327251,24.3970054241362,-8.10935056067527));
#13446=CARTESIAN_POINT('Ctrl Pts',(83.4209811102115,24.9236045838281,-8.22048367866682));
#13447=CARTESIAN_POINT('Ctrl Pts',(84.8444157086637,23.6896451127104,-8.3316167966584));
#13448=CARTESIAN_POINT('Ctrl Pts',(84.5797684537048,21.8244952919535,-8.44274991464993));
#13449=CARTESIAN_POINT('Ctrl Pts',(82.8692549315105,21.0352136465726,-8.55388303264152));
#13450=CARTESIAN_POINT('Ctrl Pts',(81.2784044417347,22.0441818055082,-8.66501615063305));
#13451=CARTESIAN_POINT('Ctrl Pts',(81.263225968394,23.9279523964684,-8.77614926862464));
#13452=CARTESIAN_POINT('Ctrl Pts',(82.8376114474537,24.9624244304365,-8.88728238661618));
#13453=CARTESIAN_POINT('Ctrl Pts',(84.5606213213977,24.2008083853429,-8.99841550460775));
#13454=CARTESIAN_POINT('Ctrl Pts',(84.8552891365203,22.3401652426527,-9.10954862259931));
#13455=CARTESIAN_POINT('Ctrl Pts',(83.4519233104416,21.0834288407163,-9.22068174059086));
#13456=CARTESIAN_POINT('Ctrl Pts',(81.634939483113,21.5808137992688,-9.33181485858243));
#13457=CARTESIAN_POINT('Ctrl Pts',(81.0673127691008,23.3770938273516,-9.44294797657398));
#13458=CARTESIAN_POINT('Ctrl Pts',(82.2685574786339,24.8282427423756,-9.55408109456554));
#13459=CARTESIAN_POINT('Ctrl Pts',(84.1392471730195,24.6061119406434,-9.6652142125571));
#13460=CARTESIAN_POINT('Ctrl Pts',(84.9672530143251,22.9140042748849,-9.77634733054867));
#13461=CARTESIAN_POINT('Ctrl Pts',(83.9947514665968,21.3006032815102,-9.88748044854021));
#13462=CARTESIAN_POINT('Ctrl Pts',(82.1118142236025,21.2425570525006,-9.99861356653178));
#13463=CARTESIAN_POINT('Ctrl Pts',(81.041779561819,22.7929917813227,-10.1097466845233));
#13464=CARTESIAN_POINT('Ctrl Pts',(81.7639853198639,24.5328885796424,-10.2208798025149));
#13465=CARTESIAN_POINT('Ctrl Pts',(83.6174403622332,24.8698254159668,-10.3320129205065));
#13466=CARTESIAN_POINT('Ctrl Pts',(84.9057896828708,23.4954244359871,-10.443146038498));
#13467=CARTESIAN_POINT('Ctrl Pts',(84.4498852745941,21.6675915124763,-10.5542791564896));
#13468=CARTESIAN_POINT('Ctrl Pts',(82.6669887960806,21.0592312798342,-10.6654122744811));
#13469=CARTESIAN_POINT('Ctrl Pts',(81.1888772785873,22.2271389678003,-10.7765453924727));
#13470=CARTESIAN_POINT('Ctrl Pts',(81.3683765608268,24.1023994919494,-10.8876785104643));
#13471=CARTESIAN_POINT('Ctrl Pts',(83.0412018346701,24.9687006110452,-10.9988116284558));
#13472=CARTESIAN_POINT('Ctrl Pts',(84.6763175677353,24.0331694436115,-11.1099447464474));
#13473=CARTESIAN_POINT('Ctrl Pts',(84.7772014835923,22.1520409362315,-11.2210778644389));
#13474=CARTESIAN_POINT('Ctrl Pts',(83.2515206516971,21.046997939356,-11.3322109824305));
#13475=CARTESIAN_POINT('Ctrl Pts',(81.4956382196122,21.7294192977939,-11.4433441004221));
#13476=CARTESIAN_POINT('Ctrl Pts',(81.116606900041,23.5747261244599,-11.5544772184136));
#13477=CARTESIAN_POINT('Ctrl Pts',(82.4613310751823,24.8940209810205,-11.6656103364052));
#13478=CARTESIAN_POINT('Ctrl Pts',(84.2990662521189,24.4798332878116,-11.7767434543967));
#13479=CARTESIAN_POINT('Ctrl Pts',(84.9478448643671,22.7112439239271,-11.8878765723883));
#13480=CARTESIAN_POINT('Ctrl Pts',(83.8138791903196,21.2069354861927,-11.9990096903798));
#13481=CARTESIAN_POINT('Ctrl Pts',(81.9350192473189,21.3437102658265,-12.1101428083714));
#13482=CARTESIAN_POINT('Ctrl Pts',(81.0308716064059,22.9963866011044,-12.221275926363));
#13483=CARTESIAN_POINT('Ctrl Pts',(81.9289477754486,24.6523700612737,-12.3324090443545));
#13484=CARTESIAN_POINT('Ctrl Pts',(83.8072930966055,24.7960394047134,-12.4435421623461));
#13485=CARTESIAN_POINT('Ctrl Pts',(84.9467720010023,23.2959027935373,-12.5546752803376));
#13486=CARTESIAN_POINT('Ctrl Pts',(84.3044885458827,21.5249442990955,-12.6658083983292));
#13487=CARTESIAN_POINT('Ctrl Pts',(82.4682858294022,21.1040148397481,-12.7769415163207));
#13488=CARTESIAN_POINT('Ctrl Pts',(81.1187288499188,22.418365624312,-12.8880746343123));
#13489=CARTESIAN_POINT('Ctrl Pts',(81.4909852731006,24.2650510824115,-12.9992077523039));
#13490=CARTESIAN_POINT('Ctrl Pts',(83.2443513685815,24.9539119979626,-13.1103408702954));
#13491=CARTESIAN_POINT('Ctrl Pts',(84.7740774739608,23.8544757477516,-13.221473988287));
#13492=CARTESIAN_POINT('Ctrl Pts',(84.6800980481614,21.9729896613604,-13.3326071062786));
#13493=CARTESIAN_POINT('Ctrl Pts',(83.0484267606719,21.0314638596256,-13.4437402242701));
#13494=CARTESIAN_POINT('Ctrl Pts',(81.3724333957525,21.8916198143882,-13.5548733422617));
#13495=CARTESIAN_POINT('Ctrl Pts',(81.1860530474464,23.7662089404431,-13.6660064602532));
#13496=CARTESIAN_POINT('Ctrl Pts',(82.6598683463564,24.9395334865117,-13.7771395782448));
#13497=CARTESIAN_POINT('Ctrl Pts',(84.4449855221666,24.337720646436,-13.8882726962363));
#13498=CARTESIAN_POINT('Ctrl Pts',(84.9075950739464,22.51157321856,-13.9994058142279));
#13499=CARTESIAN_POINT('Ctrl Pts',(83.6242985319745,21.1324532053695,-14.1105389322195));
#13500=CARTESIAN_POINT('Ctrl Pts',(81.7696194011205,21.4625855245088,-14.221672050211));
#13501=CARTESIAN_POINT('Ctrl Pts',(81.0410330222045,23.1998200837446,-14.3328051682026));
#13502=CARTESIAN_POINT('Ctrl Pts',(82.1053703244889,24.7541714373302,-14.4439382861941));
#13503=CARTESIAN_POINT('Ctrl Pts',(83.9885079202099,24.7030360482859,-14.5550714041857));
#13504=CARTESIAN_POINT('Ctrl Pts',(84.9669241558181,23.093215036347,-14.6662045221773));
#13505=CARTESIAN_POINT('Ctrl Pts',(84.145133995106,21.3980799555471,-14.7773376401688));
#13506=CARTESIAN_POINT('Ctrl Pts',(82.2752721131558,21.1690851477724,-14.8884707581604));
#13507=CARTESIAN_POINT('Ctrl Pts',(81.0687097519271,22.6158156820815,-14.9996038761519));
#13508=CARTESIAN_POINT('Ctrl Pts',(81.6297401734268,24.4141668150886,-15.1107369941435));
#13509=CARTESIAN_POINT('Ctrl Pts',(83.4448864550338,24.9182168386216,-15.2218701121351));
#13510=CARTESIAN_POINT('Ctrl Pts',(84.8528548753323,23.6666392697687,-15.3330032301266));
#13511=CARTESIAN_POINT('Ctrl Pts',(84.5650181187735,21.8049272851258,-15.4441363481182));
#13512=CARTESIAN_POINT('Ctrl Pts',(82.8448141189808,21.0369927220661,-15.5552694661097));
#13513=CARTESIAN_POINT('Ctrl Pts',(81.2666444644324,22.065680011408,-15.6664025841013));
#13514=CARTESIAN_POINT('Ctrl Pts',(81.274905794374,23.9494930737822,-15.7775357020929));
#13515=CARTESIAN_POINT('Ctrl Pts',(82.8620496683843,24.9642940096802,-15.8886688200844));
#13516=CARTESIAN_POINT('Ctrl Pts',(84.5754343067765,24.1812931487234,-15.999801938076));
#13517=CARTESIAN_POINT('Ctrl Pts',(84.8469529823893,22.3171314988683,-16.1109350560675));
#13518=CARTESIAN_POINT('Ctrl Pts',(83.4280007346583,21.077947615708,-16.2220681740591));
#13519=CARTESIAN_POINT('Ctrl Pts',(81.6174587108549,21.5979223939348,-16.3332012920506));
#13520=CARTESIAN_POINT('Ctrl Pts',(81.0720069507038,23.4010925596415,-16.4443344100422));
#13521=CARTESIAN_POINT('Ctrl Pts',(82.2916607558463,24.8372492771867,-16.5554675280338));
#13522=CARTESIAN_POINT('Ctrl Pts',(84.1585559341117,24.5917186583559,-16.6666006460253));
#13523=CARTESIAN_POINT('Ctrl Pts',(84.9672151579253,22.889718433072,-16.7777337640169));
#13524=CARTESIAN_POINT('Ctrl Pts',(83.9710651112984,21.2879181281384,-16.8888668820084));
#13525=CARTESIAN_POINT('Ctrl Pts',(82.7213583244171,21.2665677297147,-16.9629556273361));
#13526=CARTESIAN_POINT('Ctrl Pts',(82.2300979593295,21.5225674811446,-17.));
#13527=CARTESIAN_POINT('Ctrl Pts',(81.3361556106367,23.000944168981,-6.62148036339021));
#13528=CARTESIAN_POINT('Ctrl Pts',(81.335036709732,23.2166368660648,-6.63586025118848));
#13529=CARTESIAN_POINT('Ctrl Pts',(81.3739566403903,23.4319424195808,-6.65024013898675));
#13530=CARTESIAN_POINT('Ctrl Pts',(81.4547879321813,23.6301549919714,-6.66462002678502));
#13531=CARTESIAN_POINT('Ctrl Pts',(81.6630193549864,24.1407751373651,-6.70166439944887));
#13532=CARTESIAN_POINT('Ctrl Pts',(82.1493919365753,24.537959177397,-6.73870877211272));
#13533=CARTESIAN_POINT('Ctrl Pts',(82.6913214236674,24.6399610893233,-6.77575314477657));
#13534=CARTESIAN_POINT('Ctrl Pts',(83.2332509107595,24.7419630012497,-6.81279751744043));
#13535=CARTESIAN_POINT('Ctrl Pts',(83.8307373033549,24.5487827850705,-6.84984189010428));
#13536=CARTESIAN_POINT('Ctrl Pts',(84.210364378789,24.1488168856411,-6.88688626276813));
#13537=CARTESIAN_POINT('Ctrl Pts',(84.589991454223,23.7488509862116,-6.92393063543199));
#13538=CARTESIAN_POINT('Ctrl Pts',(84.7517592124957,23.1420994035318,-6.96097500809584));
#13539=CARTESIAN_POINT('Ctrl Pts',(84.6216368818937,22.6062269238159,-6.99801938075969));
#13540=CARTESIAN_POINT('Ctrl Pts',(84.4915145512917,22.0703544440999,-7.03506375342354));
#13541=CARTESIAN_POINT('Ctrl Pts',(84.069502131815,21.6053610673477,-7.07210812608739));
#13542=CARTESIAN_POINT('Ctrl Pts',(83.5487221464684,21.4240352484578,-7.10915249875125));
#13543=CARTESIAN_POINT('Ctrl Pts',(83.0279421611216,21.2427094295679,-7.1461968714151));
#13544=CARTESIAN_POINT('Ctrl Pts',(82.4083946099049,21.3450511685405,-7.18324124407896));
#13545=CARTESIAN_POINT('Ctrl Pts',(81.9735959755904,21.6842277065397,-7.22028561674282));
#13546=CARTESIAN_POINT('Ctrl Pts',(81.5776803526215,21.9930724906318,-7.25401719895862));
#13547=CARTESIAN_POINT('Ctrl Pts',(81.3349478237242,22.4982869634183,-7.28774878117441));
#13548=CARTESIAN_POINT('Ctrl Pts',(81.3317908287134,23.0008588708997,-7.32148036339021));
#13549=CARTESIAN_POINT('Ctrl Pts',(82.4698297828114,21.0148256743283,-6.));
#13550=CARTESIAN_POINT('Ctrl Pts',(82.4011651263259,21.0402496509185,-6.));
#13551=CARTESIAN_POINT('Ctrl Pts',(82.3342038137343,21.0695633264578,-6.));
#13552=CARTESIAN_POINT('Ctrl Pts',(82.269134779623,21.1024726694379,-6.));
#13553=CARTESIAN_POINT('Ctrl Pts',(82.2022546944968,21.1362979703666,-6.));
#13554=CARTESIAN_POINT('Ctrl Pts',(82.1373729168602,21.1739225674446,-6.));
#13555=CARTESIAN_POINT('Ctrl Pts',(82.0747258152859,21.2150718339324,-6.));
#13556=CARTESIAN_POINT('Ctrl Pts',(82.0217930857579,21.2498402899109,-6.));
#13557=CARTESIAN_POINT('Ctrl Pts',(81.9704560596044,21.2871261118042,-6.));
#13558=CARTESIAN_POINT('Ctrl Pts',(81.9208800568393,21.3267816542417,-6.));
#13559=CARTESIAN_POINT('Ctrl Pts',(81.8988503402036,21.3444030903036,-6.));
#13560=CARTESIAN_POINT('Ctrl Pts',(81.8771686550144,21.3624926256576,-6.));
#13561=CARTESIAN_POINT('Ctrl Pts',(81.8558510604217,21.3810380294145,-6.));
#13562=CARTESIAN_POINT('Ctrl Pts',(81.8441385158822,21.3912274467317,-6.));
#13563=CARTESIAN_POINT('Ctrl Pts',(81.832535898607,21.4015544856012,-6.));
#13564=CARTESIAN_POINT('Ctrl Pts',(81.8210460063917,21.4120171590794,-6.));
#13565=CARTESIAN_POINT('Ctrl Pts',(81.8104524191136,21.4216636590269,-6.));
#13566=CARTESIAN_POINT('Ctrl Pts',(81.7999532220216,21.4314269732589,-6.));
#13567=CARTESIAN_POINT('Ctrl Pts',(81.7895664958216,21.44129008872,-6.));
#13568=CARTESIAN_POINT('Ctrl Pts',(81.7364817397298,21.4916987611424,-6.));
#13569=CARTESIAN_POINT('Ctrl Pts',(81.6862369782681,21.5447958399209,-6.));
#13570=CARTESIAN_POINT('Ctrl Pts',(81.6390508775578,21.6003218536055,-6.));
#13571=CARTESIAN_POINT('Ctrl Pts',(81.5922309148136,21.6554170162255,-6.));
#13572=CARTESIAN_POINT('Ctrl Pts',(81.5484218215863,21.7129044490147,-6.));
#13573=CARTESIAN_POINT('Ctrl Pts',(81.5078820049586,21.7725549136341,-6.));
#13574=CARTESIAN_POINT('Ctrl Pts',(81.4741935898231,21.822124195942,-6.));
#13575=CARTESIAN_POINT('Ctrl Pts',(81.4427634303418,21.8731878200883,-6.));
#13576=CARTESIAN_POINT('Ctrl Pts',(81.4137674155173,21.9256207131518,-6.));
#13577=CARTESIAN_POINT('Ctrl Pts',(81.4016612624094,21.9475120190833,-6.));
#13578=CARTESIAN_POINT('Ctrl Pts',(81.3899797398811,21.9696420487289,-6.));
#13579=CARTESIAN_POINT('Ctrl Pts',(81.3787370903759,21.9920017823975,-6.));
#13580=CARTESIAN_POINT('Ctrl Pts',(81.3735362822328,22.0023453126204,-6.));
#13581=CARTESIAN_POINT('Ctrl Pts',(81.3684294032715,22.0127379983886,-6.));
#13582=CARTESIAN_POINT('Ctrl Pts',(81.3634179286217,22.0231789448313,-6.));
#13583=CARTESIAN_POINT('Ctrl Pts',(81.3581859277669,22.0340793373365,-6.));
#13584=CARTESIAN_POINT('Ctrl Pts',(81.3530615217638,22.045024878718,-6.));
#13585=CARTESIAN_POINT('Ctrl Pts',(81.3480477692262,22.0560102612827,-6.));
#13586=CARTESIAN_POINT('Ctrl Pts',(81.3195073639237,22.118543716704,-6.));
#13587=CARTESIAN_POINT('Ctrl Pts',(81.2945279303708,22.1824102238707,-6.));
#13588=CARTESIAN_POINT('Ctrl Pts',(81.2733329278551,22.2474053239885,-6.));
#13589=CARTESIAN_POINT('Ctrl Pts',(81.2541304646075,22.3062902436936,-6.));
#13590=CARTESIAN_POINT('Ctrl Pts',(81.2380346530873,22.3661021309141,-6.));
#13591=CARTESIAN_POINT('Ctrl Pts',(81.2252483675841,22.4266937631596,-6.));
#13592=CARTESIAN_POINT('Ctrl Pts',(81.2101158543187,22.4984036963139,-6.));
#13593=CARTESIAN_POINT('Ctrl Pts',(81.1996182649432,22.5712073072497,-6.));
#13594=CARTESIAN_POINT('Ctrl Pts',(81.1936804617054,22.6446815009142,-6.));
#13595=CARTESIAN_POINT('Ctrl Pts',(81.1923736340422,22.6608521460106,-6.));
#13596=CARTESIAN_POINT('Ctrl Pts',(81.1912878965242,22.677055190926,-6.));
#13597=CARTESIAN_POINT('Ctrl Pts',(81.1904228174184,22.693285960862,-6.));
#13598=CARTESIAN_POINT('Ctrl Pts',(81.1895274843029,22.7100843619741,-6.));
#13599=CARTESIAN_POINT('Ctrl Pts',(81.1888685034739,22.7269186557325,-6.));
#13600=CARTESIAN_POINT('Ctrl Pts',(81.1884459572869,22.7437493851286,-6.));
#13601=CARTESIAN_POINT('Ctrl Pts',(81.1867246939672,22.8123102147938,-6.));
#13602=CARTESIAN_POINT('Ctrl Pts',(81.1889150327053,22.8808986006225,-6.));
#13603=CARTESIAN_POINT('Ctrl Pts',(81.1948963902804,22.949176222518,-6.));
#13604=CARTESIAN_POINT('Ctrl Pts',(81.2008765126244,23.0174397441624,-6.));
#13605=CARTESIAN_POINT('Ctrl Pts',(81.2106465418321,23.0853937017974,-6.));
#13606=CARTESIAN_POINT('Ctrl Pts',(81.224135574421,23.1526849517223,-6.));
#13607=CARTESIAN_POINT('Ctrl Pts',(81.2338955665321,23.2013735484834,-6.));
#13608=CARTESIAN_POINT('Ctrl Pts',(81.2456035994461,23.2497149357491,-6.));
#13609=CARTESIAN_POINT('Ctrl Pts',(81.2592470183253,23.2975656941601,-6.));
#13610=CARTESIAN_POINT('Ctrl Pts',(81.2694833810369,23.3334670854062,-6.));
#13611=CARTESIAN_POINT('Ctrl Pts',(81.2808094559637,23.3690921381008,-6.));
#13612=CARTESIAN_POINT('Ctrl Pts',(81.2932238134428,23.4043761033473,-6.));
#13613=CARTESIAN_POINT('Ctrl Pts',(81.2973533007872,23.4161128918351,-6.));
#13614=CARTESIAN_POINT('Ctrl Pts',(81.3016000099352,23.427802745736,-6.));
#13615=CARTESIAN_POINT('Ctrl Pts',(81.3059632962339,23.43944310507,-6.));
#13616=CARTESIAN_POINT('Ctrl Pts',(81.3290872371389,23.5011330705975,-6.));
#13617=CARTESIAN_POINT('Ctrl Pts',(81.3554837692749,23.5614395006295,-6.));
#13618=CARTESIAN_POINT('Ctrl Pts',(81.3851028988208,23.6200283078873,-6.));
#13619=CARTESIAN_POINT('Ctrl Pts',(81.4059352451487,23.6612362144815,-6.));
#13620=CARTESIAN_POINT('Ctrl Pts',(81.4283626281757,23.7015939037268,-6.));
#13621=CARTESIAN_POINT('Ctrl Pts',(81.4523780545027,23.7409737879001,-6.));
#13622=CARTESIAN_POINT('Ctrl Pts',(81.460091064182,23.7536213846433,-6.));
#13623=CARTESIAN_POINT('Ctrl Pts',(81.4679690370099,23.7661697278492,-6.));
#13624=CARTESIAN_POINT('Ctrl Pts',(81.47600841658,23.7786089555933,-6.));
#13625=CARTESIAN_POINT('Ctrl Pts',(81.5102529542987,23.8315950846794,-6.));
#13626=CARTESIAN_POINT('Ctrl Pts',(81.5473532629023,23.8824974296264,-6.));
#13627=CARTESIAN_POINT('Ctrl Pts',(81.5872751057864,23.9310007715343,-6.));
#13628=CARTESIAN_POINT('Ctrl Pts',(81.6240617784761,23.9756950149413,-6.));
#13629=CARTESIAN_POINT('Ctrl Pts',(81.6632448080286,24.0183523539651,-6.));
#13630=CARTESIAN_POINT('Ctrl Pts',(81.7048188461966,24.0586932599642,-6.));
#13631=CARTESIAN_POINT('Ctrl Pts',(81.7126371936145,24.06627970651,-6.));
#13632=CARTESIAN_POINT('Ctrl Pts',(81.7205401543986,24.0737841268858,-6.));
#13633=CARTESIAN_POINT('Ctrl Pts',(81.7285261364169,24.0812058551231,-6.));
#13634=CARTESIAN_POINT('Origin',(83.,23.,-12.));
#13635=CARTESIAN_POINT('Origin',(83.,-23.,-18.));
#13636=CARTESIAN_POINT('Origin',(83.,23.,-18.));
#13637=CARTESIAN_POINT('Origin',(83.,-12.,-65.));
#13638=CARTESIAN_POINT('',(83.,-10.,-67.));
#13639=CARTESIAN_POINT('Origin',(83.,-10.,-65.));
#13640=CARTESIAN_POINT('',(83.,-14.,-67.));
#13641=CARTESIAN_POINT('',(83.,-12.,-67.));
#13642=CARTESIAN_POINT('Origin',(83.,-14.,-65.));
#13643=CARTESIAN_POINT('Origin',(83.,-2.22044604925031E-15,-40.));
#13644=CARTESIAN_POINT('',(83.,-10.,-44.));
#13645=CARTESIAN_POINT('Origin',(83.,-10.,-40.));
#13646=CARTESIAN_POINT('',(83.,-14.,-44.));
#13647=CARTESIAN_POINT('',(83.,-2.22044604925031E-15,-44.));
#13648=CARTESIAN_POINT('Origin',(83.,-14.,-40.));
#13649=CARTESIAN_POINT('Origin',(83.,-2.22044604925031E-15,-40.));
#13650=CARTESIAN_POINT('',(83.,14.,-44.));
#13651=CARTESIAN_POINT('Origin',(83.,14.,-40.));
#13652=CARTESIAN_POINT('',(83.,10.,-44.));
#13653=CARTESIAN_POINT('',(83.,-2.22044604925031E-15,-44.));
#13654=CARTESIAN_POINT('Origin',(83.,10.,-40.));
#13655=CARTESIAN_POINT('Origin',(77.,-10.,-70.));
#13656=CARTESIAN_POINT('',(77.,-10.,-50.));
#13657=CARTESIAN_POINT('',(77.,-14.,-50.));
#13658=CARTESIAN_POINT('',(77.,-11.,-50.));
#13659=CARTESIAN_POINT('',(77.,-10.,-70.));
#13660=CARTESIAN_POINT('',(77.,-10.,-70.));
#13661=CARTESIAN_POINT('',(77.,-14.,-70.));
#13662=CARTESIAN_POINT('',(77.,-10.,-70.));
#13663=CARTESIAN_POINT('',(77.,-14.,-70.));
#13664=CARTESIAN_POINT('Origin',(89.,-14.,-70.));
#13665=CARTESIAN_POINT('',(89.,-14.,-50.));
#13666=CARTESIAN_POINT('',(89.,-10.,-50.));
#13667=CARTESIAN_POINT('',(89.,-13.,-50.));
#13668=CARTESIAN_POINT('',(89.,-14.,-70.));
#13669=CARTESIAN_POINT('',(89.,-14.,-70.));
#13670=CARTESIAN_POINT('',(89.,-10.,-70.));
#13671=CARTESIAN_POINT('',(89.,-14.,-70.));
#13672=CARTESIAN_POINT('',(89.,-10.,-70.));
#13673=CARTESIAN_POINT('Origin',(83.,-12.,-70.));
#13674=CARTESIAN_POINT('',(89.,-10.,-70.));
#13675=CARTESIAN_POINT('',(77.,-14.,-70.));
#13676=CARTESIAN_POINT('Origin',(83.,-12.,-50.));
#13677=CARTESIAN_POINT('',(75.,-14.,-50.));
#13678=CARTESIAN_POINT('',(75.,-14.,-50.));
#13679=CARTESIAN_POINT('',(75.,-10.,-50.));
#13680=CARTESIAN_POINT('',(75.,-10.,-50.));
#13681=CARTESIAN_POINT('',(91.,-10.,-50.));
#13682=CARTESIAN_POINT('Origin',(83.,-12.,-50.));
#13683=CARTESIAN_POINT('',(91.,-10.,-50.));
#13684=CARTESIAN_POINT('',(91.,-10.,-50.));
#13685=CARTESIAN_POINT('',(91.,-14.,-50.));
#13686=CARTESIAN_POINT('',(91.,-14.,-50.));
#13687=CARTESIAN_POINT('',(75.,-14.,-50.));
#13688=CARTESIAN_POINT('Origin',(75.,10.,-50.));
#13689=CARTESIAN_POINT('',(75.,10.,-26.));
#13690=CARTESIAN_POINT('',(91.,10.,-26.));
#13691=CARTESIAN_POINT('',(79.,10.,-26.));
#13692=CARTESIAN_POINT('',(75.,10.,-50.));
#13693=CARTESIAN_POINT('',(75.,10.,-50.));
#13694=CARTESIAN_POINT('',(91.,10.,-50.));
#13695=CARTESIAN_POINT('',(75.,10.,-50.));
#13696=CARTESIAN_POINT('',(91.,10.,-50.));
#13697=CARTESIAN_POINT('Origin',(75.,14.,-50.));
#13698=CARTESIAN_POINT('',(75.,14.,-26.));
#13699=CARTESIAN_POINT('',(75.,7.,-26.));
#13700=CARTESIAN_POINT('',(75.,14.,-50.));
#13701=CARTESIAN_POINT('',(75.,14.,-50.));
#13702=CARTESIAN_POINT('',(75.,14.,-50.));
#13703=CARTESIAN_POINT('Origin',(91.,10.,-50.));
#13704=CARTESIAN_POINT('',(91.,14.,-26.));
#13705=CARTESIAN_POINT('',(91.,5.,-26.));
#13706=CARTESIAN_POINT('',(91.,14.,-50.));
#13707=CARTESIAN_POINT('',(91.,10.,-50.));
#13708=CARTESIAN_POINT('',(91.,14.,-50.));
#13709=CARTESIAN_POINT('Origin',(83.,12.,-50.));
#13710=CARTESIAN_POINT('',(91.,14.,-50.));
#13711=CARTESIAN_POINT('Origin',(83.,0.,-26.));
#13712=CARTESIAN_POINT('',(113.,14.,-26.));
#13713=CARTESIAN_POINT('',(113.,14.,-26.));
#13714=CARTESIAN_POINT('',(113.,-14.,-26.));
#13715=CARTESIAN_POINT('',(113.,-14.,-26.));
#13716=CARTESIAN_POINT('',(91.,-14.,-26.));
#13717=CARTESIAN_POINT('',(53.,-14.,-26.));
#13718=CARTESIAN_POINT('',(91.,-10.,-26.));
#13719=CARTESIAN_POINT('',(91.,-7.,-26.));
#13720=CARTESIAN_POINT('',(75.,-10.,-26.));
#13721=CARTESIAN_POINT('',(87.,-10.,-26.));
#13722=CARTESIAN_POINT('',(75.,-14.,-26.));
#13723=CARTESIAN_POINT('',(75.,-5.,-26.));
#13724=CARTESIAN_POINT('',(53.,-14.,-26.));
#13725=CARTESIAN_POINT('',(53.,-14.,-26.));
#13726=CARTESIAN_POINT('',(53.,14.,-26.));
#13727=CARTESIAN_POINT('',(53.,14.,-26.));
#13728=CARTESIAN_POINT('',(113.,14.,-26.));
#13729=CARTESIAN_POINT('',(94.,-4.,-26.));
#13730=CARTESIAN_POINT('',(102.,-4.,-26.));
#13731=CARTESIAN_POINT('',(92.5,-4.,-26.));
#13732=CARTESIAN_POINT('',(102.,4.,-26.));
#13733=CARTESIAN_POINT('',(102.,2.,-26.));
#13734=CARTESIAN_POINT('',(94.,4.,-26.));
#13735=CARTESIAN_POINT('',(88.5,4.,-26.));
#13736=CARTESIAN_POINT('',(94.,-2.,-26.));
#13737=CARTESIAN_POINT('',(64.,-4.,-26.));
#13738=CARTESIAN_POINT('',(72.,-4.,-26.));
#13739=CARTESIAN_POINT('',(77.5,-4.,-26.));
#13740=CARTESIAN_POINT('',(72.,4.,-26.));
#13741=CARTESIAN_POINT('',(72.,2.,-26.));
#13742=CARTESIAN_POINT('',(64.,4.,-26.));
#13743=CARTESIAN_POINT('',(73.5,4.,-26.));
#13744=CARTESIAN_POINT('',(64.,-2.,-26.));
#13745=CARTESIAN_POINT('Origin',(91.,-10.,-50.));
#13746=CARTESIAN_POINT('',(75.,-10.,-50.));
#13747=CARTESIAN_POINT('',(91.,-10.,-50.));
#13748=CARTESIAN_POINT('Origin',(91.,-14.,-50.));
#13749=CARTESIAN_POINT('',(91.,-14.,-50.));
#13750=CARTESIAN_POINT('Origin',(75.,-10.,-50.));
#13751=CARTESIAN_POINT('',(75.,-14.,-50.));
#13752=CARTESIAN_POINT('Origin',(53.,-14.,-26.));
#13753=CARTESIAN_POINT('',(113.,-14.,-12.));
#13754=CARTESIAN_POINT('',(113.,-14.,-26.));
#13755=CARTESIAN_POINT('',(88.,-14.,-12.));
#13756=CARTESIAN_POINT('',(53.,-14.,-12.));
#13757=CARTESIAN_POINT('',(88.,-14.,-20.));
#13758=CARTESIAN_POINT('',(88.,-14.,-23.));
#13759=CARTESIAN_POINT('',(78.,-14.,-20.));
#13760=CARTESIAN_POINT('',(68.,-14.,-20.));
#13761=CARTESIAN_POINT('',(78.,-14.,-12.));
#13762=CARTESIAN_POINT('',(78.,-14.,-23.));
#13763=CARTESIAN_POINT('',(53.,-14.,-12.));
#13764=CARTESIAN_POINT('',(53.,-14.,-12.));
#13765=CARTESIAN_POINT('',(53.,-14.,-26.));
#13766=CARTESIAN_POINT('Origin',(72.,-4.,-12.));
#13767=CARTESIAN_POINT('',(72.,-4.,-12.));
#13768=CARTESIAN_POINT('',(64.,-4.,-12.));
#13769=CARTESIAN_POINT('',(77.5,-4.,-12.));
#13770=CARTESIAN_POINT('',(72.,-4.,-12.));
#13771=CARTESIAN_POINT('',(64.,-4.,-12.));
#13772=CARTESIAN_POINT('Origin',(72.,4.,-12.));
#13773=CARTESIAN_POINT('',(72.,4.,-12.));
#13774=CARTESIAN_POINT('',(72.,2.,-12.));
#13775=CARTESIAN_POINT('',(72.,4.,-12.));
#13776=CARTESIAN_POINT('Origin',(64.,4.,-12.));
#13777=CARTESIAN_POINT('',(64.,4.,-12.));
#13778=CARTESIAN_POINT('',(73.5,4.,-12.));
#13779=CARTESIAN_POINT('',(64.,4.,-12.));
#13780=CARTESIAN_POINT('Origin',(64.,-4.,-12.));
#13781=CARTESIAN_POINT('',(64.,-2.,-12.));
#13782=CARTESIAN_POINT('Origin',(102.,-4.,-12.));
#13783=CARTESIAN_POINT('',(102.,-4.,-12.));
#13784=CARTESIAN_POINT('',(94.,-4.,-12.));
#13785=CARTESIAN_POINT('',(92.5,-4.,-12.));
#13786=CARTESIAN_POINT('',(102.,-4.,-12.));
#13787=CARTESIAN_POINT('',(94.,-4.,-12.));
#13788=CARTESIAN_POINT('Origin',(102.,4.,-12.));
#13789=CARTESIAN_POINT('',(102.,4.,-12.));
#13790=CARTESIAN_POINT('',(102.,2.,-12.));
#13791=CARTESIAN_POINT('',(102.,4.,-12.));
#13792=CARTESIAN_POINT('Origin',(94.,4.,-12.));
#13793=CARTESIAN_POINT('',(94.,4.,-12.));
#13794=CARTESIAN_POINT('',(88.5,4.,-12.));
#13795=CARTESIAN_POINT('',(94.,4.,-12.));
#13796=CARTESIAN_POINT('Origin',(94.,-4.,-12.));
#13797=CARTESIAN_POINT('',(94.,-2.,-12.));
#13798=CARTESIAN_POINT('Origin',(78.,30.,-20.));
#13799=CARTESIAN_POINT('',(78.,14.,-12.));
#13800=CARTESIAN_POINT('',(78.,14.,-20.));
#13801=CARTESIAN_POINT('',(78.,14.,-23.));
#13802=CARTESIAN_POINT('',(78.,15.,-12.));
#13803=CARTESIAN_POINT('',(78.,-30.,-20.));
#13804=CARTESIAN_POINT('',(78.,30.,-20.));
#13805=CARTESIAN_POINT('',(78.,-30.,-6.));
#13806=CARTESIAN_POINT('',(78.,-30.,-20.));
#13807=CARTESIAN_POINT('',(78.,30.,-6.));
#13808=CARTESIAN_POINT('',(78.,30.,-6.));
#13809=CARTESIAN_POINT('',(78.,30.,-20.));
#13810=CARTESIAN_POINT('',(78.,30.,-20.));
#13811=CARTESIAN_POINT('',(78.,30.,-20.));
#13812=CARTESIAN_POINT('Origin',(83.,0.,-20.));
#13813=CARTESIAN_POINT('',(88.,-30.,-20.));
#13814=CARTESIAN_POINT('',(88.,-30.,-20.));
#13815=CARTESIAN_POINT('',(78.,-30.,-20.));
#13816=CARTESIAN_POINT('Origin',(83.,0.,-20.));
#13817=CARTESIAN_POINT('',(88.,14.,-20.));
#13818=CARTESIAN_POINT('',(98.,14.,-20.));
#13819=CARTESIAN_POINT('',(88.,30.,-20.));
#13820=CARTESIAN_POINT('',(88.,30.,-20.));
#13821=CARTESIAN_POINT('',(88.,-30.,-20.));
#13822=CARTESIAN_POINT('Origin',(88.,30.,-20.));
#13823=CARTESIAN_POINT('',(88.,30.,-6.));
#13824=CARTESIAN_POINT('',(88.,30.,-6.));
#13825=CARTESIAN_POINT('',(88.,30.,-20.));
#13826=CARTESIAN_POINT('Origin',(88.,-30.,-20.));
#13827=CARTESIAN_POINT('',(88.,14.,-12.));
#13828=CARTESIAN_POINT('',(88.,14.,-23.));
#13829=CARTESIAN_POINT('',(88.,-30.,-6.));
#13830=CARTESIAN_POINT('',(88.,-30.,-6.));
#13831=CARTESIAN_POINT('',(88.,-30.,-20.));
#13832=CARTESIAN_POINT('',(88.,-15.,-12.));
#13833=CARTESIAN_POINT('Origin',(78.,-30.,-20.));
#13834=CARTESIAN_POINT('',(78.,-30.,-6.));
#13835=CARTESIAN_POINT('Origin',(83.,0.,-6.));
#13836=CARTESIAN_POINT('Origin',(83.,0.,-12.));
#13837=CARTESIAN_POINT('',(53.,14.,-12.));
#13838=CARTESIAN_POINT('',(113.,14.,-12.));
#13839=CARTESIAN_POINT('',(53.,14.,-12.));
#13840=CARTESIAN_POINT('Origin',(83.,0.,-12.));
#13841=CARTESIAN_POINT('',(113.,14.,-12.));
#13842=CARTESIAN_POINT('',(113.,-14.,-12.));
#13843=CARTESIAN_POINT('',(113.,14.,-12.));
#13844=CARTESIAN_POINT('Origin',(113.,14.,-26.));
#13845=CARTESIAN_POINT('',(53.,14.,-26.));
#13846=CARTESIAN_POINT('',(113.,14.,-26.));
#13847=CARTESIAN_POINT('Origin',(113.,-14.,-26.));
#13848=CARTESIAN_POINT('Origin',(53.,14.,-26.));
#19824=UNCERTAINTY_MEASURE_WITH_UNIT(LENGTH_MEASURE(0.01),#19864,
'DISTANCE_ACCURACY_VALUE',
'Maximum model space distance between geometric entities at asserted c
onnectivities');
#19842=UNCERTAINTY_MEASURE_WITH_UNIT(LENGTH_MEASURE(0.01),#19864,
'DISTANCE_ACCURACY_VALUE',
'Maximum model space distance between geometric entities at asserted c
onnectivities');
#19845=(
GEOMETRIC_REPRESENTATION_CONTEXT(3)
GLOBAL_UNCERTAINTY_ASSIGNED_CONTEXT((#19824))
GLOBAL_UNIT_ASSIGNED_CONTEXT((#19864,#19866,#19867))
REPRESENTATION_CONTEXT('','3D')
);
#19863=(
GEOMETRIC_REPRESENTATION_CONTEXT(3)
GLOBAL_UNCERTAINTY_ASSIGNED_CONTEXT((#19842))
GLOBAL_UNIT_ASSIGNED_CONTEXT((#19864,#19866,#19867))
REPRESENTATION_CONTEXT('','3D')
);
#19864=(
LENGTH_UNIT()
NAMED_UNIT(*)
SI_UNIT(.MILLI.,.METRE.)
);
#19866=(
NAMED_UNIT(*)
PLANE_ANGLE_UNIT()
SI_UNIT($,.RADIAN.)
);
#19867=(
NAMED_UNIT(*)
SI_UNIT($,.STERADIAN.)
SOLID_ANGLE_UNIT()
);
#19870=SHAPE_DEFINITION_REPRESENTATION(#19890,#19936);
#19890=PRODUCT_DEFINITION_SHAPE('',$,#19957);
#19936=SHAPE_REPRESENTATION('',(#6703),#19845);
#19954=PRODUCT_DEFINITION_CONTEXT('part definition',#20016,'design');
#19957=PRODUCT_DEFINITION('Guide housing','Guide housing',#19977,#19954);
#19977=PRODUCT_DEFINITION_FORMATION('',$,#20020);
#20016=APPLICATION_CONTEXT(
'Core Data for Automotive Mechanical Design Process');
#20017=PRODUCT_CONTEXT('part definition',#20016,'mechanical');
#20020=PRODUCT('Guide housing','Guide housing',$,(#20017));
#20040=PRESENTATION_STYLE_ASSIGNMENT((#20047));
#20047=SURFACE_STYLE_USAGE(.BOTH.,#20054);
#20054=SURFACE_SIDE_STYLE('',(#20061));
#20061=SURFACE_STYLE_FILL_AREA(#20068);
#20068=FILL_AREA_STYLE('Light blue',(#20075));
#20075=FILL_AREA_STYLE_COLOUR('Light blue',#20082);
#20082=COLOUR_RGB('Light blue',0.662745098039216,0.831372549019608,0.949019607843137);
ENDSEC;
END-ISO-10303-21;
